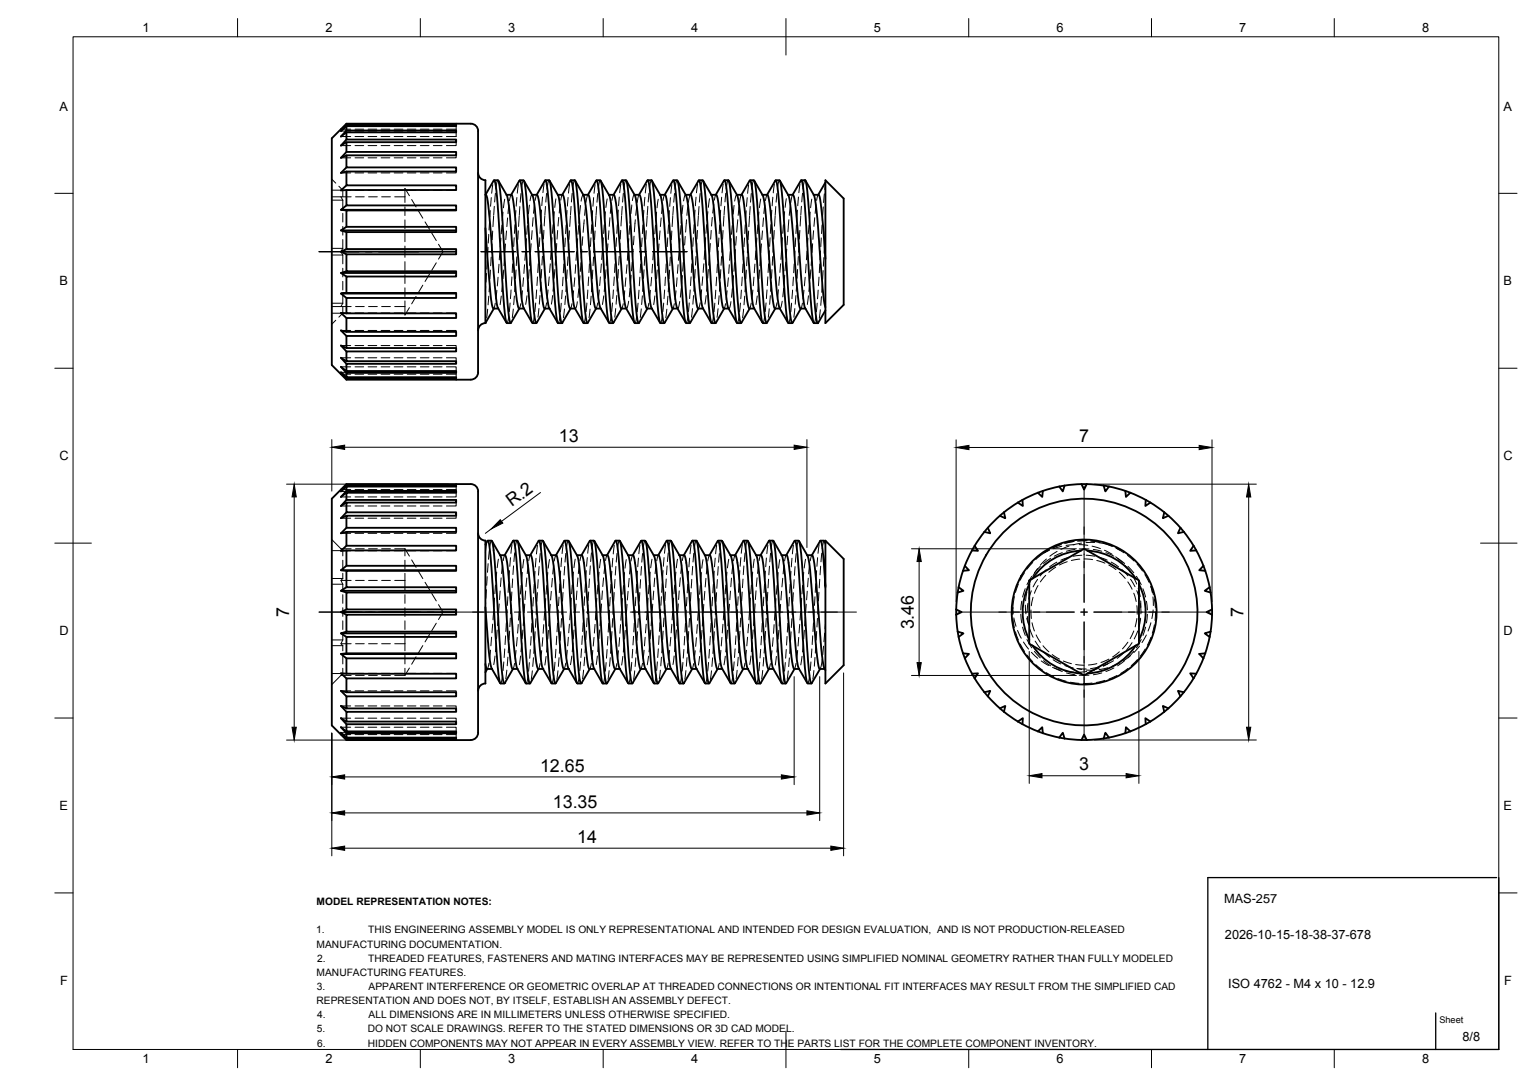
ISO-10303-21;
HEADER;
FILE_DESCRIPTION((''),'2;1');
FILE_NAME('ISO 4762 - M4 x 10 - 12.9.step','2026-10-05T22:33:56+05:00',(''),(''),'','','');
FILE_SCHEMA (('AUTOMOTIVE_DESIGN { 1 0 10303 214 3 1 1 }'));
ENDSEC;
DATA;
#10=MECHANICAL_DESIGN_GEOMETRIC_PRESENTATION_REPRESENTATION('',(#433),#16942);
#231=(
BOUNDED_CURVE()
B_SPLINE_CURVE(2,(#15819,#15820,#15821),.UNSPECIFIED.,.F.,.F.)
B_SPLINE_CURVE_WITH_KNOTS((3,3),(0.0385503582642466,0.0599944283303575),
 .UNSPECIFIED.)
CURVE()
GEOMETRIC_REPRESENTATION_ITEM()
RATIONAL_B_SPLINE_CURVE((1.0010577858677,1.00082309557272,1.))
REPRESENTATION_ITEM('')
) ;
#232=(
BOUNDED_CURVE()
B_SPLINE_CURVE(2,(#15833,#15834,#15835),.UNSPECIFIED.,.F.,.F.)
B_SPLINE_CURVE_WITH_KNOTS((3,3),(0.,0.0214440700661964),.UNSPECIFIED.)
CURVE()
GEOMETRIC_REPRESENTATION_ITEM()
RATIONAL_B_SPLINE_CURVE((1.,1.00082309556609,1.00105778585917))
REPRESENTATION_ITEM('')
) ;
#233=(
BOUNDED_CURVE()
B_SPLINE_CURVE(2,(#16126,#16127,#16128),.UNSPECIFIED.,.F.,.F.)
B_SPLINE_CURVE_WITH_KNOTS((3,3),(0.0385503582641958,0.0599944283303579),
 .UNSPECIFIED.)
CURVE()
GEOMETRIC_REPRESENTATION_ITEM()
RATIONAL_B_SPLINE_CURVE((1.00105778586472,1.00082309557041,1.))
REPRESENTATION_ITEM('')
) ;
#234=(
BOUNDED_CURVE()
B_SPLINE_CURVE(2,(#16135,#16136,#16137),.UNSPECIFIED.,.F.,.F.)
B_SPLINE_CURVE_WITH_KNOTS((3,3),(0.,0.0214440700661411),.UNSPECIFIED.)
CURVE()
GEOMETRIC_REPRESENTATION_ITEM()
RATIONAL_B_SPLINE_CURVE((1.,1.00082309557092,1.00105778586538))
REPRESENTATION_ITEM('')
) ;
#235=(
BOUNDED_CURVE()
B_SPLINE_CURVE(2,(#16140,#16141,#16142),.UNSPECIFIED.,.F.,.F.)
B_SPLINE_CURVE_WITH_KNOTS((3,3),(0.0385503582642588,0.0599944283303573),
 .UNSPECIFIED.)
CURVE()
GEOMETRIC_REPRESENTATION_ITEM()
RATIONAL_B_SPLINE_CURVE((1.00105778587296,1.00082309557682,1.))
REPRESENTATION_ITEM('')
) ;
#236=(
BOUNDED_CURVE()
B_SPLINE_CURVE(2,(#16149,#16150,#16151),.UNSPECIFIED.,.F.,.F.)
B_SPLINE_CURVE_WITH_KNOTS((3,3),(0.,0.0214440700661923),.UNSPECIFIED.)
CURVE()
GEOMETRIC_REPRESENTATION_ITEM()
RATIONAL_B_SPLINE_CURVE((1.,1.00082309556743,1.00105778586089))
REPRESENTATION_ITEM('')
) ;
#237=(
BOUNDED_CURVE()
B_SPLINE_CURVE(2,(#16154,#16155,#16156),.UNSPECIFIED.,.F.,.F.)
B_SPLINE_CURVE_WITH_KNOTS((3,3),(0.0385503582642198,0.0599944283303572),
 .UNSPECIFIED.)
CURVE()
GEOMETRIC_REPRESENTATION_ITEM()
RATIONAL_B_SPLINE_CURVE((1.00105778586562,1.00082309557111,1.))
REPRESENTATION_ITEM('')
) ;
#238=(
BOUNDED_CURVE()
B_SPLINE_CURVE(2,(#16163,#16164,#16165),.UNSPECIFIED.,.F.,.F.)
B_SPLINE_CURVE_WITH_KNOTS((3,3),(0.,0.0214440700661772),.UNSPECIFIED.)
CURVE()
GEOMETRIC_REPRESENTATION_ITEM()
RATIONAL_B_SPLINE_CURVE((1.,1.00082309556912,1.00105778586306))
REPRESENTATION_ITEM('')
) ;
#239=(
BOUNDED_CURVE()
B_SPLINE_CURVE(2,(#16168,#16169,#16170),.UNSPECIFIED.,.F.,.F.)
B_SPLINE_CURVE_WITH_KNOTS((3,3),(0.0385503582641919,0.0599944283303571),
 .UNSPECIFIED.)
CURVE()
GEOMETRIC_REPRESENTATION_ITEM()
RATIONAL_B_SPLINE_CURVE((1.00105778586425,1.00082309557004,1.))
REPRESENTATION_ITEM('')
) ;
#240=(
BOUNDED_CURVE()
B_SPLINE_CURVE(2,(#16177,#16178,#16179),.UNSPECIFIED.,.F.,.F.)
B_SPLINE_CURVE_WITH_KNOTS((3,3),(0.,0.02144407006609),.UNSPECIFIED.)
CURVE()
GEOMETRIC_REPRESENTATION_ITEM()
RATIONAL_B_SPLINE_CURVE((1.,1.0008230955718,1.00105778586652))
REPRESENTATION_ITEM('')
) ;
#241=(
BOUNDED_CURVE()
B_SPLINE_CURVE(2,(#16182,#16183,#16184),.UNSPECIFIED.,.F.,.F.)
B_SPLINE_CURVE_WITH_KNOTS((3,3),(0.0385503582642022,0.0599944283303558),
 .UNSPECIFIED.)
CURVE()
GEOMETRIC_REPRESENTATION_ITEM()
RATIONAL_B_SPLINE_CURVE((1.00105778586255,1.00082309556872,1.))
REPRESENTATION_ITEM('')
) ;
#242=(
BOUNDED_CURVE()
B_SPLINE_CURVE(2,(#16191,#16192,#16193),.UNSPECIFIED.,.F.,.F.)
B_SPLINE_CURVE_WITH_KNOTS((3,3),(0.,0.0214440700661625),.UNSPECIFIED.)
CURVE()
GEOMETRIC_REPRESENTATION_ITEM()
RATIONAL_B_SPLINE_CURVE((1.,1.00082309557089,1.00105778586534))
REPRESENTATION_ITEM('')
) ;
#243=(
BOUNDED_CURVE()
B_SPLINE_CURVE(2,(#16196,#16197,#16198),.UNSPECIFIED.,.F.,.F.)
B_SPLINE_CURVE_WITH_KNOTS((3,3),(0.038550358264205,0.0599944283303565),
 .UNSPECIFIED.)
CURVE()
GEOMETRIC_REPRESENTATION_ITEM()
RATIONAL_B_SPLINE_CURVE((1.00105778586624,1.00082309557159,1.))
REPRESENTATION_ITEM('')
) ;
#244=(
BOUNDED_CURVE()
B_SPLINE_CURVE(2,(#16205,#16206,#16207),.UNSPECIFIED.,.F.,.F.)
B_SPLINE_CURVE_WITH_KNOTS((3,3),(0.,0.0214440700661342),.UNSPECIFIED.)
CURVE()
GEOMETRIC_REPRESENTATION_ITEM()
RATIONAL_B_SPLINE_CURVE((1.,1.00082309557258,1.00105778586751))
REPRESENTATION_ITEM('')
) ;
#245=(
BOUNDED_CURVE()
B_SPLINE_CURVE(2,(#16210,#16211,#16212),.UNSPECIFIED.,.F.,.F.)
B_SPLINE_CURVE_WITH_KNOTS((3,3),(0.0385503582641691,0.0599944283303568),
 .UNSPECIFIED.)
CURVE()
GEOMETRIC_REPRESENTATION_ITEM()
RATIONAL_B_SPLINE_CURVE((1.00105778586269,1.00082309556883,1.))
REPRESENTATION_ITEM('')
) ;
#246=(
BOUNDED_CURVE()
B_SPLINE_CURVE(2,(#16219,#16220,#16221),.UNSPECIFIED.,.F.,.F.)
B_SPLINE_CURVE_WITH_KNOTS((3,3),(0.,0.0214440700661154),.UNSPECIFIED.)
CURVE()
GEOMETRIC_REPRESENTATION_ITEM()
RATIONAL_B_SPLINE_CURVE((1.,1.00082309557543,1.00105778587117))
REPRESENTATION_ITEM('')
) ;
#247=(
BOUNDED_CURVE()
B_SPLINE_CURVE(2,(#16224,#16225,#16226),.UNSPECIFIED.,.F.,.F.)
B_SPLINE_CURVE_WITH_KNOTS((3,3),(0.0385503582642171,0.0599944283303574),
 .UNSPECIFIED.)
CURVE()
GEOMETRIC_REPRESENTATION_ITEM()
RATIONAL_B_SPLINE_CURVE((1.00105778586904,1.00082309557377,1.))
REPRESENTATION_ITEM('')
) ;
#248=(
BOUNDED_CURVE()
B_SPLINE_CURVE(2,(#16233,#16234,#16235),.UNSPECIFIED.,.F.,.F.)
B_SPLINE_CURVE_WITH_KNOTS((3,3),(0.,0.0214440700661167),.UNSPECIFIED.)
CURVE()
GEOMETRIC_REPRESENTATION_ITEM()
RATIONAL_B_SPLINE_CURVE((1.,1.00082309557365,1.00105778586889))
REPRESENTATION_ITEM('')
) ;
#249=(
BOUNDED_CURVE()
B_SPLINE_CURVE(2,(#16238,#16239,#16240),.UNSPECIFIED.,.F.,.F.)
B_SPLINE_CURVE_WITH_KNOTS((3,3),(0.0385503582642811,0.0599944283303564),
 .UNSPECIFIED.)
CURVE()
GEOMETRIC_REPRESENTATION_ITEM()
RATIONAL_B_SPLINE_CURVE((1.00105778587046,1.00082309557487,1.))
REPRESENTATION_ITEM('')
) ;
#250=(
BOUNDED_CURVE()
B_SPLINE_CURVE(2,(#16247,#16248,#16249),.UNSPECIFIED.,.F.,.F.)
B_SPLINE_CURVE_WITH_KNOTS((3,3),(0.,0.0214440700661453),.UNSPECIFIED.)
CURVE()
GEOMETRIC_REPRESENTATION_ITEM()
RATIONAL_B_SPLINE_CURVE((1.,1.00082309557136,1.00105778586595))
REPRESENTATION_ITEM('')
) ;
#251=(
BOUNDED_CURVE()
B_SPLINE_CURVE(2,(#16252,#16253,#16254),.UNSPECIFIED.,.F.,.F.)
B_SPLINE_CURVE_WITH_KNOTS((3,3),(0.0385503582642705,0.0599944283303552),
 .UNSPECIFIED.)
CURVE()
GEOMETRIC_REPRESENTATION_ITEM()
RATIONAL_B_SPLINE_CURVE((1.00105778586715,1.0008230955723,1.))
REPRESENTATION_ITEM('')
) ;
#252=(
BOUNDED_CURVE()
B_SPLINE_CURVE(2,(#16261,#16262,#16263),.UNSPECIFIED.,.F.,.F.)
B_SPLINE_CURVE_WITH_KNOTS((3,3),(0.,0.0214440700661215),.UNSPECIFIED.)
CURVE()
GEOMETRIC_REPRESENTATION_ITEM()
RATIONAL_B_SPLINE_CURVE((1.,1.00082309557137,1.00105778586595))
REPRESENTATION_ITEM('')
) ;
#253=(
BOUNDED_CURVE()
B_SPLINE_CURVE(2,(#16266,#16267,#16268),.UNSPECIFIED.,.F.,.F.)
B_SPLINE_CURVE_WITH_KNOTS((3,3),(0.0385503582641931,0.0599944283303567),
 .UNSPECIFIED.)
CURVE()
GEOMETRIC_REPRESENTATION_ITEM()
RATIONAL_B_SPLINE_CURVE((1.00105778586386,1.00082309556974,1.))
REPRESENTATION_ITEM('')
) ;
#254=(
BOUNDED_CURVE()
B_SPLINE_CURVE(2,(#16275,#16276,#16277),.UNSPECIFIED.,.F.,.F.)
B_SPLINE_CURVE_WITH_KNOTS((3,3),(0.,0.0214440700661656),.UNSPECIFIED.)
CURVE()
GEOMETRIC_REPRESENTATION_ITEM()
RATIONAL_B_SPLINE_CURVE((1.,1.00082309557042,1.00105778586474))
REPRESENTATION_ITEM('')
) ;
#255=(
BOUNDED_CURVE()
B_SPLINE_CURVE(2,(#16280,#16281,#16282),.UNSPECIFIED.,.F.,.F.)
B_SPLINE_CURVE_WITH_KNOTS((3,3),(0.0385503582642439,0.0599944283303563),
 .UNSPECIFIED.)
CURVE()
GEOMETRIC_REPRESENTATION_ITEM()
RATIONAL_B_SPLINE_CURVE((1.00105778586994,1.00082309557447,1.))
REPRESENTATION_ITEM('')
) ;
#256=(
BOUNDED_CURVE()
B_SPLINE_CURVE(2,(#16289,#16290,#16291),.UNSPECIFIED.,.F.,.F.)
B_SPLINE_CURVE_WITH_KNOTS((3,3),(0.,0.0214440700660658),.UNSPECIFIED.)
CURVE()
GEOMETRIC_REPRESENTATION_ITEM()
RATIONAL_B_SPLINE_CURVE((1.,1.00082309557484,1.00105778587042))
REPRESENTATION_ITEM('')
) ;
#257=(
BOUNDED_CURVE()
B_SPLINE_CURVE(2,(#16294,#16295,#16296),.UNSPECIFIED.,.F.,.F.)
B_SPLINE_CURVE_WITH_KNOTS((3,3),(0.0385503582642125,0.0599944283303565),
 .UNSPECIFIED.)
CURVE()
GEOMETRIC_REPRESENTATION_ITEM()
RATIONAL_B_SPLINE_CURVE((1.00105778586599,1.0008230955714,1.))
REPRESENTATION_ITEM('')
) ;
#258=(
BOUNDED_CURVE()
B_SPLINE_CURVE(2,(#16303,#16304,#16305),.UNSPECIFIED.,.F.,.F.)
B_SPLINE_CURVE_WITH_KNOTS((3,3),(0.,0.0214440700661045),.UNSPECIFIED.)
CURVE()
GEOMETRIC_REPRESENTATION_ITEM()
RATIONAL_B_SPLINE_CURVE((1.,1.00082309557375,1.00105778586901))
REPRESENTATION_ITEM('')
) ;
#259=(
BOUNDED_CURVE()
B_SPLINE_CURVE(2,(#16308,#16309,#16310),.UNSPECIFIED.,.F.,.F.)
B_SPLINE_CURVE_WITH_KNOTS((3,3),(0.0385503582642445,0.0599944283303561),
 .UNSPECIFIED.)
CURVE()
GEOMETRIC_REPRESENTATION_ITEM()
RATIONAL_B_SPLINE_CURVE((1.00105778586579,1.00082309557124,1.))
REPRESENTATION_ITEM('')
) ;
#260=(
BOUNDED_CURVE()
B_SPLINE_CURVE(2,(#16317,#16318,#16319),.UNSPECIFIED.,.F.,.F.)
B_SPLINE_CURVE_WITH_KNOTS((3,3),(0.,0.021444070066132),.UNSPECIFIED.)
CURVE()
GEOMETRIC_REPRESENTATION_ITEM()
RATIONAL_B_SPLINE_CURVE((1.,1.00082309557227,1.00105778586711))
REPRESENTATION_ITEM('')
) ;
#261=(
BOUNDED_CURVE()
B_SPLINE_CURVE(2,(#16322,#16323,#16324),.UNSPECIFIED.,.F.,.F.)
B_SPLINE_CURVE_WITH_KNOTS((3,3),(0.03855035826422,0.0599944283303558),
 .UNSPECIFIED.)
CURVE()
GEOMETRIC_REPRESENTATION_ITEM()
RATIONAL_B_SPLINE_CURVE((1.00105778586627,1.00082309557161,1.))
REPRESENTATION_ITEM('')
) ;
#262=(
BOUNDED_CURVE()
B_SPLINE_CURVE(2,(#16331,#16332,#16333),.UNSPECIFIED.,.F.,.F.)
B_SPLINE_CURVE_WITH_KNOTS((3,3),(0.,0.0214440700661134),.UNSPECIFIED.)
CURVE()
GEOMETRIC_REPRESENTATION_ITEM()
RATIONAL_B_SPLINE_CURVE((1.,1.00082309557282,1.00105778586782))
REPRESENTATION_ITEM('')
) ;
#263=(
BOUNDED_CURVE()
B_SPLINE_CURVE(2,(#16336,#16337,#16338),.UNSPECIFIED.,.F.,.F.)
B_SPLINE_CURVE_WITH_KNOTS((3,3),(0.0385503582642076,0.0599944283303568),
 .UNSPECIFIED.)
CURVE()
GEOMETRIC_REPRESENTATION_ITEM()
RATIONAL_B_SPLINE_CURVE((1.00105778586756,1.00082309557262,1.))
REPRESENTATION_ITEM('')
) ;
#264=(
BOUNDED_CURVE()
B_SPLINE_CURVE(2,(#16345,#16346,#16347),.UNSPECIFIED.,.F.,.F.)
B_SPLINE_CURVE_WITH_KNOTS((3,3),(0.,0.0214440700660783),.UNSPECIFIED.)
CURVE()
GEOMETRIC_REPRESENTATION_ITEM()
RATIONAL_B_SPLINE_CURVE((1.,1.00082309557531,1.00105778587102))
REPRESENTATION_ITEM('')
) ;
#265=(
BOUNDED_CURVE()
B_SPLINE_CURVE(2,(#16350,#16351,#16352),.UNSPECIFIED.,.F.,.F.)
B_SPLINE_CURVE_WITH_KNOTS((3,3),(0.0385503582642354,0.0599944283303562),
 .UNSPECIFIED.)
CURVE()
GEOMETRIC_REPRESENTATION_ITEM()
RATIONAL_B_SPLINE_CURVE((1.0010577858655,1.00082309557101,1.))
REPRESENTATION_ITEM('')
) ;
#266=(
BOUNDED_CURVE()
B_SPLINE_CURVE(2,(#16359,#16360,#16361),.UNSPECIFIED.,.F.,.F.)
B_SPLINE_CURVE_WITH_KNOTS((3,3),(0.,0.021444070066152),.UNSPECIFIED.)
CURVE()
GEOMETRIC_REPRESENTATION_ITEM()
RATIONAL_B_SPLINE_CURVE((1.,1.00082309556975,1.00105778586387))
REPRESENTATION_ITEM('')
) ;
#267=(
BOUNDED_CURVE()
B_SPLINE_CURVE(2,(#16364,#16365,#16366),.UNSPECIFIED.,.F.,.F.)
B_SPLINE_CURVE_WITH_KNOTS((3,3),(0.0385503582642177,0.0599944283303568),
 .UNSPECIFIED.)
CURVE()
GEOMETRIC_REPRESENTATION_ITEM()
RATIONAL_B_SPLINE_CURVE((1.00105778586644,1.00082309557175,1.))
REPRESENTATION_ITEM('')
) ;
#268=(
BOUNDED_CURVE()
B_SPLINE_CURVE(2,(#16373,#16374,#16375),.UNSPECIFIED.,.F.,.F.)
B_SPLINE_CURVE_WITH_KNOTS((3,3),(0.,0.0214440700661323),.UNSPECIFIED.)
CURVE()
GEOMETRIC_REPRESENTATION_ITEM()
RATIONAL_B_SPLINE_CURVE((1.,1.00082309557161,1.00105778586626))
REPRESENTATION_ITEM('')
) ;
#269=(
BOUNDED_CURVE()
B_SPLINE_CURVE(2,(#16378,#16379,#16380),.UNSPECIFIED.,.F.,.F.)
B_SPLINE_CURVE_WITH_KNOTS((3,3),(0.0385503582642313,0.0599944283303566),
 .UNSPECIFIED.)
CURVE()
GEOMETRIC_REPRESENTATION_ITEM()
RATIONAL_B_SPLINE_CURVE((1.00105778586689,1.0008230955721,1.))
REPRESENTATION_ITEM('')
) ;
#270=(
BOUNDED_CURVE()
B_SPLINE_CURVE(2,(#16387,#16388,#16389),.UNSPECIFIED.,.F.,.F.)
B_SPLINE_CURVE_WITH_KNOTS((3,3),(0.,0.0214440700661231),.UNSPECIFIED.)
CURVE()
GEOMETRIC_REPRESENTATION_ITEM()
RATIONAL_B_SPLINE_CURVE((1.,1.00082309557192,1.00105778586666))
REPRESENTATION_ITEM('')
) ;
#271=(
BOUNDED_CURVE()
B_SPLINE_CURVE(2,(#16392,#16393,#16394),.UNSPECIFIED.,.F.,.F.)
B_SPLINE_CURVE_WITH_KNOTS((3,3),(0.0385503582642438,0.0599944283303561),
 .UNSPECIFIED.)
CURVE()
GEOMETRIC_REPRESENTATION_ITEM()
RATIONAL_B_SPLINE_CURVE((1.00105778586773,1.00082309557275,1.))
REPRESENTATION_ITEM('')
) ;
#272=(
BOUNDED_CURVE()
B_SPLINE_CURVE(2,(#16401,#16402,#16403),.UNSPECIFIED.,.F.,.F.)
B_SPLINE_CURVE_WITH_KNOTS((3,3),(0.,0.0214440700661489),.UNSPECIFIED.)
CURVE()
GEOMETRIC_REPRESENTATION_ITEM()
RATIONAL_B_SPLINE_CURVE((1.,1.00082309557108,1.00105778586558))
REPRESENTATION_ITEM('')
) ;
#273=(
BOUNDED_CURVE()
B_SPLINE_CURVE(2,(#16406,#16407,#16408),.UNSPECIFIED.,.F.,.F.)
B_SPLINE_CURVE_WITH_KNOTS((3,3),(0.0385503582642491,0.0599944283303561),
 .UNSPECIFIED.)
CURVE()
GEOMETRIC_REPRESENTATION_ITEM()
RATIONAL_B_SPLINE_CURVE((1.00105778586862,1.00082309557344,1.))
REPRESENTATION_ITEM('')
) ;
#274=(
BOUNDED_CURVE()
B_SPLINE_CURVE(2,(#16415,#16416,#16417),.UNSPECIFIED.,.F.,.F.)
B_SPLINE_CURVE_WITH_KNOTS((3,3),(0.,0.0214440700660912),.UNSPECIFIED.)
CURVE()
GEOMETRIC_REPRESENTATION_ITEM()
RATIONAL_B_SPLINE_CURVE((1.,1.00082309557531,1.00105778587103))
REPRESENTATION_ITEM('')
) ;
#275=(
BOUNDED_CURVE()
B_SPLINE_CURVE(2,(#16420,#16421,#16422),.UNSPECIFIED.,.F.,.F.)
B_SPLINE_CURVE_WITH_KNOTS((3,3),(0.0385503582642475,0.0599944283303563),
 .UNSPECIFIED.)
CURVE()
GEOMETRIC_REPRESENTATION_ITEM()
RATIONAL_B_SPLINE_CURVE((1.0010577858671,1.00082309557226,1.))
REPRESENTATION_ITEM('')
) ;
#276=(
BOUNDED_CURVE()
B_SPLINE_CURVE(2,(#16429,#16430,#16431),.UNSPECIFIED.,.F.,.F.)
B_SPLINE_CURVE_WITH_KNOTS((3,3),(0.,0.0214440700661173),.UNSPECIFIED.)
CURVE()
GEOMETRIC_REPRESENTATION_ITEM()
RATIONAL_B_SPLINE_CURVE((1.,1.00082309557298,1.00105778586803))
REPRESENTATION_ITEM('')
) ;
#277=(
BOUNDED_CURVE()
B_SPLINE_CURVE(2,(#16434,#16435,#16436),.UNSPECIFIED.,.F.,.F.)
B_SPLINE_CURVE_WITH_KNOTS((3,3),(0.0385503582641958,0.0599944283303564),
 .UNSPECIFIED.)
CURVE()
GEOMETRIC_REPRESENTATION_ITEM()
RATIONAL_B_SPLINE_CURVE((1.00105778586416,1.00082309556997,1.))
REPRESENTATION_ITEM('')
) ;
#278=(
BOUNDED_CURVE()
B_SPLINE_CURVE(2,(#16443,#16444,#16445),.UNSPECIFIED.,.F.,.F.)
B_SPLINE_CURVE_WITH_KNOTS((3,3),(0.,0.0214440700660895),.UNSPECIFIED.)
CURVE()
GEOMETRIC_REPRESENTATION_ITEM()
RATIONAL_B_SPLINE_CURVE((1.,1.00082309557376,1.00105778586903))
REPRESENTATION_ITEM('')
) ;
#279=(
BOUNDED_CURVE()
B_SPLINE_CURVE(2,(#16448,#16449,#16450),.UNSPECIFIED.,.F.,.F.)
B_SPLINE_CURVE_WITH_KNOTS((3,3),(0.0385503582642543,0.0599944283303558),
 .UNSPECIFIED.)
CURVE()
GEOMETRIC_REPRESENTATION_ITEM()
RATIONAL_B_SPLINE_CURVE((1.00105778586867,1.00082309557348,1.))
REPRESENTATION_ITEM('')
) ;
#280=(
BOUNDED_CURVE()
B_SPLINE_CURVE(2,(#16457,#16458,#16459),.UNSPECIFIED.,.F.,.F.)
B_SPLINE_CURVE_WITH_KNOTS((3,3),(0.,0.0214440700661381),.UNSPECIFIED.)
CURVE()
GEOMETRIC_REPRESENTATION_ITEM()
RATIONAL_B_SPLINE_CURVE((1.,1.00082309557261,1.00105778586756))
REPRESENTATION_ITEM('')
) ;
#281=(
BOUNDED_CURVE()
B_SPLINE_CURVE(2,(#16462,#16463,#16464),.UNSPECIFIED.,.F.,.F.)
B_SPLINE_CURVE_WITH_KNOTS((3,3),(0.0385503582642087,0.0599944283303561),
 .UNSPECIFIED.)
CURVE()
GEOMETRIC_REPRESENTATION_ITEM()
RATIONAL_B_SPLINE_CURVE((1.00105778586395,1.0008230955698,1.))
REPRESENTATION_ITEM('')
) ;
#282=(
BOUNDED_CURVE()
B_SPLINE_CURVE(2,(#16471,#16472,#16473),.UNSPECIFIED.,.F.,.F.)
B_SPLINE_CURVE_WITH_KNOTS((3,3),(0.,0.0214440700661082),.UNSPECIFIED.)
CURVE()
GEOMETRIC_REPRESENTATION_ITEM()
RATIONAL_B_SPLINE_CURVE((1.,1.00082309557413,1.00105778586951))
REPRESENTATION_ITEM('')
) ;
#283=(
BOUNDED_CURVE()
B_SPLINE_CURVE(2,(#16476,#16477,#16478),.UNSPECIFIED.,.F.,.F.)
B_SPLINE_CURVE_WITH_KNOTS((3,3),(0.0385503582642435,0.0599944283303565),
 .UNSPECIFIED.)
CURVE()
GEOMETRIC_REPRESENTATION_ITEM()
RATIONAL_B_SPLINE_CURVE((1.00105778586698,1.00082309557217,1.))
REPRESENTATION_ITEM('')
) ;
#284=(
BOUNDED_CURVE()
B_SPLINE_CURVE(2,(#16485,#16486,#16487),.UNSPECIFIED.,.F.,.F.)
B_SPLINE_CURVE_WITH_KNOTS((3,3),(0.,0.0214440700661165),.UNSPECIFIED.)
CURVE()
GEOMETRIC_REPRESENTATION_ITEM()
RATIONAL_B_SPLINE_CURVE((1.,1.00082309557299,1.00105778586805))
REPRESENTATION_ITEM('')
) ;
#285=(
BOUNDED_CURVE()
B_SPLINE_CURVE(2,(#16490,#16491,#16492),.UNSPECIFIED.,.F.,.F.)
B_SPLINE_CURVE_WITH_KNOTS((3,3),(0.0385503582642354,0.0599944283303561),
 .UNSPECIFIED.)
CURVE()
GEOMETRIC_REPRESENTATION_ITEM()
RATIONAL_B_SPLINE_CURVE((1.00105778586729,1.00082309557241,1.))
REPRESENTATION_ITEM('')
) ;
#286=(
BOUNDED_CURVE()
B_SPLINE_CURVE(2,(#16499,#16500,#16501),.UNSPECIFIED.,.F.,.F.)
B_SPLINE_CURVE_WITH_KNOTS((3,3),(0.,0.0214440700661208),.UNSPECIFIED.)
CURVE()
GEOMETRIC_REPRESENTATION_ITEM()
RATIONAL_B_SPLINE_CURVE((1.,1.00082309557164,1.0010577858663))
REPRESENTATION_ITEM('')
) ;
#287=(
BOUNDED_CURVE()
B_SPLINE_CURVE(2,(#16504,#16505,#16506),.UNSPECIFIED.,.F.,.F.)
B_SPLINE_CURVE_WITH_KNOTS((3,3),(0.0385503582642138,0.0599944283303558),
 .UNSPECIFIED.)
CURVE()
GEOMETRIC_REPRESENTATION_ITEM()
RATIONAL_B_SPLINE_CURVE((1.0010577858656,1.00082309557109,1.))
REPRESENTATION_ITEM('')
) ;
#288=(
BOUNDED_CURVE()
B_SPLINE_CURVE(2,(#16513,#16514,#16515),.UNSPECIFIED.,.F.,.F.)
B_SPLINE_CURVE_WITH_KNOTS((3,3),(0.,0.0214440700661239),.UNSPECIFIED.)
CURVE()
GEOMETRIC_REPRESENTATION_ITEM()
RATIONAL_B_SPLINE_CURVE((1.,1.00082309557102,1.0010577858655))
REPRESENTATION_ITEM('')
) ;
#289=(
BOUNDED_CURVE()
B_SPLINE_CURVE(2,(#16518,#16519,#16520),.UNSPECIFIED.,.F.,.F.)
B_SPLINE_CURVE_WITH_KNOTS((3,3),(0.0385503582643101,0.0599944283303554),
 .UNSPECIFIED.)
CURVE()
GEOMETRIC_REPRESENTATION_ITEM()
RATIONAL_B_SPLINE_CURVE((1.00105778587441,1.00082309557795,1.))
REPRESENTATION_ITEM('')
) ;
#290=(
BOUNDED_CURVE()
B_SPLINE_CURVE(2,(#16527,#16528,#16529),.UNSPECIFIED.,.F.,.F.)
B_SPLINE_CURVE_WITH_KNOTS((3,3),(0.,0.021444070066082),.UNSPECIFIED.)
CURVE()
GEOMETRIC_REPRESENTATION_ITEM()
RATIONAL_B_SPLINE_CURVE((1.,1.0008230955747,1.00105778587023))
REPRESENTATION_ITEM('')
) ;
#291=(
BOUNDED_CURVE()
B_SPLINE_CURVE(2,(#16532,#16533,#16534),.UNSPECIFIED.,.F.,.F.)
B_SPLINE_CURVE_WITH_KNOTS((3,3),(0.0385503582643354,0.0599944283303546),
 .UNSPECIFIED.)
CURVE()
GEOMETRIC_REPRESENTATION_ITEM()
RATIONAL_B_SPLINE_CURVE((1.00105778587483,1.00082309557827,1.))
REPRESENTATION_ITEM('')
) ;
#292=(
BOUNDED_CURVE()
B_SPLINE_CURVE(2,(#16541,#16542,#16543),.UNSPECIFIED.,.F.,.F.)
B_SPLINE_CURVE_WITH_KNOTS((3,3),(0.,0.0214440700660534),.UNSPECIFIED.)
CURVE()
GEOMETRIC_REPRESENTATION_ITEM()
RATIONAL_B_SPLINE_CURVE((1.,1.0008230955765,1.00105778587255))
REPRESENTATION_ITEM('')
) ;
#293=(
BOUNDED_CURVE()
B_SPLINE_CURVE(2,(#16546,#16547,#16548),.UNSPECIFIED.,.F.,.F.)
B_SPLINE_CURVE_WITH_KNOTS((3,3),(0.038550358264337,0.0599944283303554),
 .UNSPECIFIED.)
CURVE()
GEOMETRIC_REPRESENTATION_ITEM()
RATIONAL_B_SPLINE_CURVE((1.00105778587529,1.00082309557863,1.))
REPRESENTATION_ITEM('')
) ;
#294=(
BOUNDED_CURVE()
B_SPLINE_CURVE(2,(#16555,#16556,#16557),.UNSPECIFIED.,.F.,.F.)
B_SPLINE_CURVE_WITH_KNOTS((3,3),(0.,0.0214440700660699),.UNSPECIFIED.)
CURVE()
GEOMETRIC_REPRESENTATION_ITEM()
RATIONAL_B_SPLINE_CURVE((1.,1.00082309557688,1.00105778587304))
REPRESENTATION_ITEM('')
) ;
#295=(
BOUNDED_CURVE()
B_SPLINE_CURVE(2,(#16560,#16561,#16562),.UNSPECIFIED.,.F.,.F.)
B_SPLINE_CURVE_WITH_KNOTS((3,3),(0.0385503582642283,0.0599944283303555),
 .UNSPECIFIED.)
CURVE()
GEOMETRIC_REPRESENTATION_ITEM()
RATIONAL_B_SPLINE_CURVE((1.00105778586715,1.0008230955723,1.))
REPRESENTATION_ITEM('')
) ;
#296=(
BOUNDED_CURVE()
B_SPLINE_CURVE(2,(#16569,#16570,#16571),.UNSPECIFIED.,.F.,.F.)
B_SPLINE_CURVE_WITH_KNOTS((3,3),(0.,0.0214440700660926),.UNSPECIFIED.)
CURVE()
GEOMETRIC_REPRESENTATION_ITEM()
RATIONAL_B_SPLINE_CURVE((1.,1.00082309557397,1.0010577858693))
REPRESENTATION_ITEM('')
) ;
#297=(
BOUNDED_CURVE()
B_SPLINE_CURVE(2,(#16574,#16575,#16576),.UNSPECIFIED.,.F.,.F.)
B_SPLINE_CURVE_WITH_KNOTS((3,3),(0.0385503582642555,0.0599944283303555),
 .UNSPECIFIED.)
CURVE()
GEOMETRIC_REPRESENTATION_ITEM()
RATIONAL_B_SPLINE_CURVE((1.00105778587096,1.00082309557526,1.))
REPRESENTATION_ITEM('')
) ;
#298=(
BOUNDED_CURVE()
B_SPLINE_CURVE(2,(#16583,#16584,#16585),.UNSPECIFIED.,.F.,.F.)
B_SPLINE_CURVE_WITH_KNOTS((3,3),(0.,0.0214440700660555),.UNSPECIFIED.)
CURVE()
GEOMETRIC_REPRESENTATION_ITEM()
RATIONAL_B_SPLINE_CURVE((1.,1.00082309557703,1.00105778587323))
REPRESENTATION_ITEM('')
) ;
#299=(
BOUNDED_CURVE()
B_SPLINE_CURVE(2,(#16588,#16589,#16590),.UNSPECIFIED.,.F.,.F.)
B_SPLINE_CURVE_WITH_KNOTS((3,3),(0.0385503582642982,0.059994428330355),
 .UNSPECIFIED.)
CURVE()
GEOMETRIC_REPRESENTATION_ITEM()
RATIONAL_B_SPLINE_CURVE((1.00105778587101,1.0008230955753,1.))
REPRESENTATION_ITEM('')
) ;
#300=(
BOUNDED_CURVE()
B_SPLINE_CURVE(2,(#16597,#16598,#16599),.UNSPECIFIED.,.F.,.F.)
B_SPLINE_CURVE_WITH_KNOTS((3,3),(0.,0.0214440700660737),.UNSPECIFIED.)
CURVE()
GEOMETRIC_REPRESENTATION_ITEM()
RATIONAL_B_SPLINE_CURVE((1.,1.00082309557534,1.00105778587106))
REPRESENTATION_ITEM('')
) ;
#301=(
BOUNDED_CURVE()
B_SPLINE_CURVE(2,(#16602,#16603,#16604),.UNSPECIFIED.,.F.,.F.)
B_SPLINE_CURVE_WITH_KNOTS((3,3),(0.0385503582642702,0.0599944283303555),
 .UNSPECIFIED.)
CURVE()
GEOMETRIC_REPRESENTATION_ITEM()
RATIONAL_B_SPLINE_CURVE((1.00105778587074,1.00082309557509,1.))
REPRESENTATION_ITEM('')
) ;
#302=(
BOUNDED_CURVE()
B_SPLINE_CURVE(2,(#16611,#16612,#16613),.UNSPECIFIED.,.F.,.F.)
B_SPLINE_CURVE_WITH_KNOTS((3,3),(0.,0.0214440700660954),.UNSPECIFIED.)
CURVE()
GEOMETRIC_REPRESENTATION_ITEM()
RATIONAL_B_SPLINE_CURVE((1.,1.00082309557337,1.00105778586853))
REPRESENTATION_ITEM('')
) ;
#303=(
BOUNDED_CURVE()
B_SPLINE_CURVE(2,(#16626,#16627,#16628),.UNSPECIFIED.,.F.,.F.)
B_SPLINE_CURVE_WITH_KNOTS((3,3),(0.,0.0128119220385747),.UNSPECIFIED.)
CURVE()
GEOMETRIC_REPRESENTATION_ITEM()
RATIONAL_B_SPLINE_CURVE((1.,1.00225826788916,1.0035731078451))
REPRESENTATION_ITEM('')
) ;
#304=(
BOUNDED_CURVE()
B_SPLINE_CURVE(2,(#16632,#16633,#16634),.UNSPECIFIED.,.F.,.F.)
B_SPLINE_CURVE_WITH_KNOTS((3,3),(0.0485234510605496,0.0613353730991217),
 .UNSPECIFIED.)
CURVE()
GEOMETRIC_REPRESENTATION_ITEM()
RATIONAL_B_SPLINE_CURVE((1.00357310784516,1.0022582678892,1.))
REPRESENTATION_ITEM('')
) ;
#305=(
BOUNDED_CURVE()
B_SPLINE_CURVE(2,(#16636,#16637,#16638),.UNSPECIFIED.,.F.,.F.)
B_SPLINE_CURVE_WITH_KNOTS((3,3),(0.,0.0128119217509423),.UNSPECIFIED.)
CURVE()
GEOMETRIC_REPRESENTATION_ITEM()
RATIONAL_B_SPLINE_CURVE((1.,1.00225826778645,1.00357310769076))
REPRESENTATION_ITEM('')
) ;
#306=(
BOUNDED_CURVE()
B_SPLINE_CURVE(2,(#16642,#16643,#16644),.UNSPECIFIED.,.F.,.F.)
B_SPLINE_CURVE_WITH_KNOTS((3,3),(0.0485234554560875,0.0613353722533859),
 .UNSPECIFIED.)
CURVE()
GEOMETRIC_REPRESENTATION_ITEM()
RATIONAL_B_SPLINE_CURVE((1.00357310667489,1.00225826691386,1.))
REPRESENTATION_ITEM('')
) ;
#307=(
BOUNDED_CURVE()
B_SPLINE_CURVE(2,(#16646,#16647,#16648),.UNSPECIFIED.,.F.,.F.)
B_SPLINE_CURVE_WITH_KNOTS((3,3),(0.,0.0128119162220165),.UNSPECIFIED.)
CURVE()
GEOMETRIC_REPRESENTATION_ITEM()
RATIONAL_B_SPLINE_CURVE((1.,1.00225826670891,1.00357310636695))
REPRESENTATION_ITEM('')
) ;
#308=(
BOUNDED_CURVE()
B_SPLINE_CURVE(2,(#16652,#16653,#16654),.UNSPECIFIED.,.F.,.F.)
B_SPLINE_CURVE_WITH_KNOTS((3,3),(0.048523459293524,0.0613353705619148),
 .UNSPECIFIED.)
CURVE()
GEOMETRIC_REPRESENTATION_ITEM()
RATIONAL_B_SPLINE_CURVE((1.00357310535024,1.00225826583579,1.))
REPRESENTATION_ITEM('')
) ;
#309=(
BOUNDED_CURVE()
B_SPLINE_CURVE(2,(#16656,#16657,#16658),.UNSPECIFIED.,.F.,.F.)
B_SPLINE_CURVE_WITH_KNOTS((3,3),(0.,0.0128119109807577),.UNSPECIFIED.)
CURVE()
GEOMETRIC_REPRESENTATION_ITEM()
RATIONAL_B_SPLINE_CURVE((1.,1.002258265733,1.00357310519577))
REPRESENTATION_ITEM('')
) ;
#310=(
BOUNDED_CURVE()
B_SPLINE_CURVE(2,(#16662,#16663,#16664),.UNSPECIFIED.,.F.,.F.)
B_SPLINE_CURVE_WITH_KNOTS((3,3),(0.0485234587354268,0.0613353697161783),
 .UNSPECIFIED.)
CURVE()
GEOMETRIC_REPRESENTATION_ITEM()
RATIONAL_B_SPLINE_CURVE((1.00357310519621,1.00225826573327,1.))
REPRESENTATION_ITEM('')
) ;
#311=(
BOUNDED_CURVE()
B_SPLINE_CURVE(2,(#16666,#16667,#16668),.UNSPECIFIED.,.F.,.F.)
B_SPLINE_CURVE_WITH_KNOTS((3,3),(0.,0.0128119112683924),.UNSPECIFIED.)
CURVE()
GEOMETRIC_REPRESENTATION_ITEM()
RATIONAL_B_SPLINE_CURVE((1.,1.00225826583572,1.00357310535012))
REPRESENTATION_ITEM('')
) ;
#312=(
BOUNDED_CURVE()
B_SPLINE_CURVE(2,(#16672,#16673,#16674),.UNSPECIFIED.,.F.,.F.)
B_SPLINE_CURVE_WITH_KNOTS((3,3),(0.0485234543398934,0.0613353705619145),
 .UNSPECIFIED.)
CURVE()
GEOMETRIC_REPRESENTATION_ITEM()
RATIONAL_B_SPLINE_CURVE((1.00357310636678,1.0022582667088,1.))
REPRESENTATION_ITEM('')
) ;
#313=(
BOUNDED_CURVE()
B_SPLINE_CURVE(2,(#16677,#16678,#16679),.UNSPECIFIED.,.F.,.F.)
B_SPLINE_CURVE_WITH_KNOTS((3,3),(0.,0.0128119167973088),.UNSPECIFIED.)
CURVE()
GEOMETRIC_REPRESENTATION_ITEM()
RATIONAL_B_SPLINE_CURVE((1.,1.00225826691344,1.00357310667422))
REPRESENTATION_ITEM('')
) ;
#314=(
BOUNDED_CURVE()
B_SPLINE_CURVE(2,(#16682,#16683,#16684),.UNSPECIFIED.,.F.,.F.)
B_SPLINE_CURVE_WITH_KNOTS((3,3),(0.0485234505024517,0.0613353722533853),
 .UNSPECIFIED.)
CURVE()
GEOMETRIC_REPRESENTATION_ITEM()
RATIONAL_B_SPLINE_CURVE((1.00357310769125,1.00225826778676,1.))
REPRESENTATION_ITEM('')
) ;
#317=TOROIDAL_SURFACE('',#8634,2.154,0.2) ;
#318=TOROIDAL_SURFACE('',#8827,3.3,0.2) ;
#413=B_SPLINE_SURFACE_WITH_KNOTS('',3,3,((#14885,#14886,#14887,#14888,#14889,
#14890,#14891,#14892,#14893,#14894,#14895,#14896,#14897,#14898,#14899,#14900,
#14901,#14902,#14903,#14904,#14905,#14906,#14907,#14908,#14909,#14910,#14911,
#14912,#14913,#14914,#14915,#14916,#14917,#14918,#14919,#14920,#14921,#14922,
#14923,#14924,#14925,#14926,#14927,#14928,#14929,#14930,#14931,#14932,#14933,
#14934,#14935,#14936,#14937,#14938,#14939,#14940,#14941,#14942,#14943,#14944,
#14945,#14946,#14947,#14948,#14949,#14950,#14951,#14952,#14953,#14954,#14955,
#14956,#14957,#14958,#14959,#14960,#14961,#14962,#14963,#14964,#14965,#14966,
#14967,#14968,#14969,#14970,#14971,#14972,#14973),(#14974,#14975,#14976,
#14977,#14978,#14979,#14980,#14981,#14982,#14983,#14984,#14985,#14986,#14987,
#14988,#14989,#14990,#14991,#14992,#14993,#14994,#14995,#14996,#14997,#14998,
#14999,#15000,#15001,#15002,#15003,#15004,#15005,#15006,#15007,#15008,#15009,
#15010,#15011,#15012,#15013,#15014,#15015,#15016,#15017,#15018,#15019,#15020,
#15021,#15022,#15023,#15024,#15025,#15026,#15027,#15028,#15029,#15030,#15031,
#15032,#15033,#15034,#15035,#15036,#15037,#15038,#15039,#15040,#15041,#15042,
#15043,#15044,#15045,#15046,#15047,#15048,#15049,#15050,#15051,#15052,#15053,
#15054,#15055,#15056,#15057,#15058,#15059,#15060,#15061,#15062),(#15063,
#15064,#15065,#15066,#15067,#15068,#15069,#15070,#15071,#15072,#15073,#15074,
#15075,#15076,#15077,#15078,#15079,#15080,#15081,#15082,#15083,#15084,#15085,
#15086,#15087,#15088,#15089,#15090,#15091,#15092,#15093,#15094,#15095,#15096,
#15097,#15098,#15099,#15100,#15101,#15102,#15103,#15104,#15105,#15106,#15107,
#15108,#15109,#15110,#15111,#15112,#15113,#15114,#15115,#15116,#15117,#15118,
#15119,#15120,#15121,#15122,#15123,#15124,#15125,#15126,#15127,#15128,#15129,
#15130,#15131,#15132,#15133,#15134,#15135,#15136,#15137,#15138,#15139,#15140,
#15141,#15142,#15143,#15144,#15145,#15146,#15147,#15148,#15149,#15150,#15151),
(#15152,#15153,#15154,#15155,#15156,#15157,#15158,#15159,#15160,#15161,
#15162,#15163,#15164,#15165,#15166,#15167,#15168,#15169,#15170,#15171,#15172,
#15173,#15174,#15175,#15176,#15177,#15178,#15179,#15180,#15181,#15182,#15183,
#15184,#15185,#15186,#15187,#15188,#15189,#15190,#15191,#15192,#15193,#15194,
#15195,#15196,#15197,#15198,#15199,#15200,#15201,#15202,#15203,#15204,#15205,
#15206,#15207,#15208,#15209,#15210,#15211,#15212,#15213,#15214,#15215,#15216,
#15217,#15218,#15219,#15220,#15221,#15222,#15223,#15224,#15225,#15226,#15227,
#15228,#15229,#15230,#15231,#15232,#15233,#15234,#15235,#15236,#15237,#15238,
#15239,#15240)),.UNSPECIFIED.,.F.,.F.,.F.,(4,4),(4,1,1,1,1,1,1,1,1,1,1,
1,1,1,1,1,1,1,1,1,1,1,1,1,1,1,1,1,1,1,1,1,1,1,1,1,1,1,1,1,1,1,1,1,1,1,1,
1,1,1,1,1,1,1,1,1,1,1,1,1,1,1,1,1,1,1,1,1,1,1,1,1,1,1,1,1,1,1,1,1,1,1,1,
1,1,1,4),(0.,0.0460148164544131),(8.31058692273963,9.30525837539851,10.2999298280574,
11.2946012807163,12.2892727333752,13.2839441860341,14.2786156386929,15.2732870913518,
16.2679585440107,17.2626299966696,18.2573014493285,19.2519729019874,20.2466443546463,
21.2413158073051,22.235987259964,23.2306587126229,24.2253301652818,25.2200016179407,
26.2146730705996,27.2093445232584,28.2040159759173,29.1986874285762,30.1933588812351,
31.188030333894,32.1827017865529,33.1773732392118,34.1720446918706,35.1667161445295,
36.1613875971884,37.1560590498473,38.1507305025062,39.1454019551651,40.1400734078239,
41.1347448604828,42.1294163131417,43.1240877658006,44.1187592184595,45.1134306711184,
46.1081021237773,47.1027735764361,48.097445029095,49.0921164817539,50.0867879344128,
51.0814593870717,52.0761308397306,53.0708022923895,54.0654737450483,55.0601451977072,
56.0548166503661,57.049488103025,58.0441595556839,59.0388310083428,60.0335024610017,
61.0281739136605,62.0228453663194,63.0175168189783,64.0121882716372,65.0068597242961,
66.001531176955,66.9962026296138,67.9908740822727,68.9855455349316,69.9802169875905,
70.9748884402494,71.9695598929083,72.9642313455672,73.958902798226,74.9535742508849,
75.9482457035438,76.9429171562027,77.9375886088616,78.9322600615205,79.9269315141794,
80.9216029668382,81.9162744194971,82.910945872156,83.9056173248149,84.9002887774738,
85.8949602301327,86.8896316827915,87.8843031354504,88.8789745881093,89.8736460407682,
90.8683174934271,91.862988946086,92.8576603987449,93.8523318514037),
 .UNSPECIFIED.) ;
#414=B_SPLINE_SURFACE_WITH_KNOTS('',3,3,((#15446,#15447,#15448,#15449,#15450,
#15451,#15452,#15453,#15454,#15455,#15456,#15457,#15458,#15459,#15460,#15461,
#15462,#15463,#15464,#15465,#15466,#15467,#15468,#15469,#15470,#15471,#15472,
#15473,#15474,#15475,#15476,#15477,#15478,#15479,#15480,#15481,#15482,#15483,
#15484,#15485,#15486,#15487,#15488,#15489,#15490,#15491,#15492,#15493,#15494,
#15495,#15496,#15497,#15498,#15499,#15500,#15501,#15502,#15503,#15504,#15505,
#15506,#15507,#15508,#15509,#15510,#15511,#15512,#15513,#15514,#15515,#15516,
#15517,#15518,#15519,#15520,#15521,#15522,#15523,#15524,#15525,#15526,#15527,
#15528,#15529,#15530,#15531,#15532,#15533,#15534),(#15535,#15536,#15537,
#15538,#15539,#15540,#15541,#15542,#15543,#15544,#15545,#15546,#15547,#15548,
#15549,#15550,#15551,#15552,#15553,#15554,#15555,#15556,#15557,#15558,#15559,
#15560,#15561,#15562,#15563,#15564,#15565,#15566,#15567,#15568,#15569,#15570,
#15571,#15572,#15573,#15574,#15575,#15576,#15577,#15578,#15579,#15580,#15581,
#15582,#15583,#15584,#15585,#15586,#15587,#15588,#15589,#15590,#15591,#15592,
#15593,#15594,#15595,#15596,#15597,#15598,#15599,#15600,#15601,#15602,#15603,
#15604,#15605,#15606,#15607,#15608,#15609,#15610,#15611,#15612,#15613,#15614,
#15615,#15616,#15617,#15618,#15619,#15620,#15621,#15622,#15623),(#15624,
#15625,#15626,#15627,#15628,#15629,#15630,#15631,#15632,#15633,#15634,#15635,
#15636,#15637,#15638,#15639,#15640,#15641,#15642,#15643,#15644,#15645,#15646,
#15647,#15648,#15649,#15650,#15651,#15652,#15653,#15654,#15655,#15656,#15657,
#15658,#15659,#15660,#15661,#15662,#15663,#15664,#15665,#15666,#15667,#15668,
#15669,#15670,#15671,#15672,#15673,#15674,#15675,#15676,#15677,#15678,#15679,
#15680,#15681,#15682,#15683,#15684,#15685,#15686,#15687,#15688,#15689,#15690,
#15691,#15692,#15693,#15694,#15695,#15696,#15697,#15698,#15699,#15700,#15701,
#15702,#15703,#15704,#15705,#15706,#15707,#15708,#15709,#15710,#15711,#15712),
(#15713,#15714,#15715,#15716,#15717,#15718,#15719,#15720,#15721,#15722,
#15723,#15724,#15725,#15726,#15727,#15728,#15729,#15730,#15731,#15732,#15733,
#15734,#15735,#15736,#15737,#15738,#15739,#15740,#15741,#15742,#15743,#15744,
#15745,#15746,#15747,#15748,#15749,#15750,#15751,#15752,#15753,#15754,#15755,
#15756,#15757,#15758,#15759,#15760,#15761,#15762,#15763,#15764,#15765,#15766,
#15767,#15768,#15769,#15770,#15771,#15772,#15773,#15774,#15775,#15776,#15777,
#15778,#15779,#15780,#15781,#15782,#15783,#15784,#15785,#15786,#15787,#15788,
#15789,#15790,#15791,#15792,#15793,#15794,#15795,#15796,#15797,#15798,#15799,
#15800,#15801)),.UNSPECIFIED.,.F.,.F.,.F.,(4,4),(4,1,1,1,1,1,1,1,1,1,1,
1,1,1,1,1,1,1,1,1,1,1,1,1,1,1,1,1,1,1,1,1,1,1,1,1,1,1,1,1,1,1,1,1,1,1,1,
1,1,1,1,1,1,1,1,1,1,1,1,1,1,1,1,1,1,1,1,1,1,1,1,1,1,1,1,1,1,1,1,1,1,1,1,
1,1,1,4),(0.,0.0460148164544131),(11.6154215191105,12.6100929717694,13.6047644244283,
14.5994358770872,15.594107329746,16.5887787824049,17.5834502350638,18.5781216877227,
19.5727931403816,20.5674645930405,21.5621360456994,22.5568074983582,23.5514789510171,
24.546150403676,25.5408218563349,26.5354933089938,27.5301647616527,28.5248362143116,
29.5195076669704,30.5141791196293,31.5088505722882,32.5035220249471,33.498193477606,
34.4928649302649,35.4875363829238,36.4822078355826,37.4768792882415,38.4715507409004,
39.4662221935593,40.4608936462182,41.4555650988771,42.450236551536,43.4449080041948,
44.4395794568537,45.4342509095126,46.4289223621715,47.4235938148304,48.4182652674893,
49.4129367201481,50.407608172807,51.4022796254659,52.3969510781248,53.3916225307837,
54.3862939834426,55.3809654361015,56.3756368887603,57.3703083414192,58.3649797940781,
59.359651246737,60.3543226993959,61.3489941520548,62.3436656047136,63.3383370573725,
64.3330085100314,65.3276799626903,66.3223514153492,67.3170228680081,68.311694320667,
69.3063657733259,70.3010372259847,71.2957086786436,72.2903801313025,73.2850515839614,
74.2797230366203,75.2743944892792,76.2690659419381,77.2637373945969,78.2584088472558,
79.2530802999147,80.2477517525736,81.2424232052325,82.2370946578914,83.2317661105503,
84.2264375632091,85.221109015868,86.2157804685269,87.2104519211858,88.2051233738447,
89.1997948265036,90.1944662791624,91.1891377318213,92.1838091844802,93.1784806371391,
94.173152089798,95.1678235424569,96.1624949951158,97.1571664477746),
 .UNSPECIFIED.) ;
#419=SHAPE_REPRESENTATION_RELATIONSHIP('SRR','None',#17023,#426) ;
#426=ADVANCED_BREP_SHAPE_REPRESENTATION('',(#440),#16939) ;
#433=STYLED_ITEM('',(#17067),#440) ;
#440=MANIFOLD_SOLID_BREP('ISO 4762 - M4 x 10 - 12.9',#8182) ;
#625=B_SPLINE_CURVE_WITH_KNOTS('',3,(#13724,#13725,#13726,#13727,#13728,
#13729,#13730,#13731,#13732,#13733),.UNSPECIFIED.,.F.,.F.,(4,3,3,4),(-4.09254174883839,
-3.97868581063554,-2.98401435797666,-2.06514013327809),.UNSPECIFIED.) ;
#626=B_SPLINE_CURVE_WITH_KNOTS('',3,(#13736,#13737,#13738,#13739,#13740,
#13741,#13742),.UNSPECIFIED.,.F.,.F.,(4,3,4),(0.,0.994671452658877,1.11419103802963),
 .UNSPECIFIED.) ;
#627=B_SPLINE_CURVE_WITH_KNOTS('',3,(#13747,#13748,#13749,#13750,#13751,
#13752,#13753,#13754,#13755,#13756,#13757,#13758,#13759,#13760,#13761,#13762,
#13763,#13764,#13765,#13766,#13767,#13768),.UNSPECIFIED.,.F.,.F.,(4,3,3,
3,3,3,3,4),(-10.375727056018,-9.94671452658885,-8.95204307392997,-7.95737162127108,
-6.96270016861219,-5.96802871595331,-4.97335726329442,-4.09254174883839),
 .UNSPECIFIED.) ;
#628=B_SPLINE_CURVE_WITH_KNOTS('',3,(#13769,#13770,#13771,#13772,#13773,
#13774,#13775,#13776,#13777,#13778,#13779,#13780,#13781,#13782,#13783,#13784,
#13785,#13786,#13787,#13788,#13789,#13790),.UNSPECIFIED.,.F.,.F.,(4,3,3,
3,3,3,3,4),(1.11419103802963,1.98934290531777,2.98401435797665,3.97868581063554,
4.97335726329443,5.96802871595332,6.96270016861221,7.3973763452092),
 .UNSPECIFIED.) ;
#629=B_SPLINE_CURVE_WITH_KNOTS('',3,(#13795,#13796,#13797,#13798,#13799,
#13800,#13801,#13802,#13803,#13804,#13805,#13806,#13807,#13808,#13809,#13810,
#13811,#13812,#13813,#13814,#13815,#13816),.UNSPECIFIED.,.F.,.F.,(4,3,3,
3,3,3,3,4),(-16.6589123631976,-15.9147432425422,-14.9200717898833,-13.9254003372244,
-12.9307288845655,-11.9360574319066,-10.9413859792477,-10.375727056018),
 .UNSPECIFIED.) ;
#630=B_SPLINE_CURVE_WITH_KNOTS('',3,(#13817,#13818,#13819,#13820,#13821,
#13822,#13823,#13824,#13825,#13826,#13827,#13828,#13829,#13830,#13831,#13832,
#13833,#13834,#13835,#13836,#13837,#13838),.UNSPECIFIED.,.F.,.F.,(4,3,3,
3,3,3,3,4),(7.3973763452092,7.95737162127109,8.95204307392997,9.94671452658885,
10.9413859792477,11.9360574319066,12.9307288845655,13.6805616523888),
 .UNSPECIFIED.) ;
#631=B_SPLINE_CURVE_WITH_KNOTS('',3,(#13843,#13844,#13845,#13846,#13847,
#13848,#13849,#13850,#13851,#13852,#13853,#13854,#13855,#13856,#13857,#13858,
#13859,#13860,#13861,#13862,#13863,#13864,#13865,#13866,#13867),
 .UNSPECIFIED.,.F.,.F.,(4,3,3,3,3,3,3,3,4),(-22.9420976703771,-22.8774434111544,
-21.8827719584955,-20.8881005058366,-19.8934290531777,-18.8987576005188,
-17.9040861478599,-16.9094146952011,-16.6589123631976),.UNSPECIFIED.) ;
#632=B_SPLINE_CURVE_WITH_KNOTS('',3,(#13868,#13869,#13870,#13871,#13872,
#13873,#13874,#13875,#13876,#13877,#13878,#13879,#13880,#13881,#13882,#13883,
#13884,#13885,#13886,#13887,#13888,#13889,#13890,#13891,#13892),
 .UNSPECIFIED.,.F.,.F.,(4,3,3,3,3,3,3,3,4),(13.6805616523888,13.9254003372244,
14.9200717898833,15.9147432425422,16.909414695201,17.9040861478599,18.8987576005188,
19.8934290531777,19.9637469595684),.UNSPECIFIED.) ;
#633=B_SPLINE_CURVE_WITH_KNOTS('',3,(#13897,#13898,#13899,#13900,#13901,
#13902,#13903,#13904,#13905,#13906,#13907,#13908,#13909,#13910,#13911,#13912,
#13913,#13914,#13915,#13916,#13917,#13918),.UNSPECIFIED.,.F.,.F.,(4,3,3,
3,3,3,3,4),(-29.2252829775567,-28.8454721271077,-27.8508006744488,-26.8561292217899,
-25.861457769131,-24.8667863164721,-23.8721148638132,-22.9420976703771),
 .UNSPECIFIED.) ;
#634=B_SPLINE_CURVE_WITH_KNOTS('',3,(#13919,#13920,#13921,#13922,#13923,
#13924,#13925,#13926,#13927,#13928,#13929,#13930,#13931,#13932,#13933,#13934,
#13935,#13936,#13937,#13938,#13939,#13940),.UNSPECIFIED.,.F.,.F.,(4,3,3,
3,3,3,3,4),(19.9637469595684,20.8881005058366,21.8827719584955,22.8774434111544,
23.8721148638132,24.8667863164721,25.861457769131,26.246932266748),
 .UNSPECIFIED.) ;
#635=B_SPLINE_CURVE_WITH_KNOTS('',3,(#13945,#13946,#13947,#13948,#13949,
#13950,#13951,#13952,#13953,#13954,#13955,#13956,#13957,#13958,#13959,#13960,
#13961,#13962,#13963,#13964,#13965,#13966),.UNSPECIFIED.,.F.,.F.,(4,3,3,
3,3,3,3,4),(-35.5084682847363,-34.813500843061,-33.8188293904021,-32.8241579377432,
-31.8294864850843,-30.8348150324254,-29.8401435797666,-29.2252829775567),
 .UNSPECIFIED.) ;
#636=B_SPLINE_CURVE_WITH_KNOTS('',3,(#13967,#13968,#13969,#13970,#13971,
#13972,#13973,#13974,#13975,#13976,#13977,#13978,#13979,#13980,#13981,#13982,
#13983,#13984,#13985,#13986,#13987,#13988),.UNSPECIFIED.,.F.,.F.,(4,3,3,
3,3,3,3,4),(26.246932266748,26.8561292217899,27.8508006744488,28.8454721271077,
29.8401435797665,30.8348150324254,31.8294864850843,32.5301175739276),
 .UNSPECIFIED.) ;
#637=B_SPLINE_CURVE_WITH_KNOTS('',3,(#13993,#13994,#13995,#13996,#13997,
#13998,#13999,#14000,#14001,#14002,#14003,#14004,#14005,#14006,#14007,#14008,
#14009,#14010,#14011,#14012,#14013,#14014,#14015,#14016,#14017),
 .UNSPECIFIED.,.F.,.F.,(4,3,3,3,3,3,3,3,4),(-41.7916535919159,-41.7762010116732,
-40.7815295590143,-39.7868581063554,-38.7921866536965,-37.7975152010376,
-36.8028437483788,-35.8081722957199,-35.5084682847363),.UNSPECIFIED.) ;
#638=B_SPLINE_CURVE_WITH_KNOTS('',3,(#14018,#14019,#14020,#14021,#14022,
#14023,#14024,#14025,#14026,#14027,#14028,#14029,#14030,#14031,#14032,#14033,
#14034,#14035,#14036,#14037,#14038,#14039,#14040,#14041,#14042),
 .UNSPECIFIED.,.F.,.F.,(4,3,3,3,3,3,3,3,4),(32.5301175739276,32.8241579377432,
33.8188293904021,34.813500843061,35.8081722957199,36.8028437483787,37.7975152010376,
38.7921866536965,38.8133028811071),.UNSPECIFIED.) ;
#639=B_SPLINE_CURVE_WITH_KNOTS('',3,(#14047,#14048,#14049,#14050,#14051,
#14052,#14053,#14054,#14055,#14056,#14057,#14058,#14059,#14060,#14061,#14062,
#14063,#14064,#14065,#14066,#14067,#14068),.UNSPECIFIED.,.F.,.F.,(4,3,3,
3,3,3,3,4),(-48.0748388990955,-47.7442297276265,-46.7495582749676,-45.7548868223087,
-44.7602153696498,-43.765543916991,-42.7708724643321,-41.7916535919159),
 .UNSPECIFIED.) ;
#640=B_SPLINE_CURVE_WITH_KNOTS('',3,(#14069,#14070,#14071,#14072,#14073,
#14074,#14075,#14076,#14077,#14078,#14079,#14080,#14081,#14082,#14083,#14084,
#14085,#14086,#14087,#14088,#14089,#14090),.UNSPECIFIED.,.F.,.F.,(4,3,3,
3,3,3,3,4),(38.8133028811071,39.7868581063554,40.7815295590143,41.7762010116732,
42.7708724643321,43.7655439169909,44.7602153696498,45.0964881882867),
 .UNSPECIFIED.) ;
#641=B_SPLINE_CURVE_WITH_KNOTS('',3,(#14095,#14096,#14097,#14098,#14099,
#14100,#14101,#14102,#14103,#14104,#14105,#14106,#14107,#14108,#14109,#14110,
#14111,#14112,#14113,#14114,#14115,#14116),.UNSPECIFIED.,.F.,.F.,(4,3,3,
3,3,3,3,4),(-54.3580242062751,-53.7122584435798,-52.7175869909209,-51.722915538262,
-50.7282440856032,-49.7335726329443,-48.7389011802854,-48.0748388990955),
 .UNSPECIFIED.) ;
#642=B_SPLINE_CURVE_WITH_KNOTS('',3,(#14117,#14118,#14119,#14120,#14121,
#14122,#14123,#14124,#14125,#14126,#14127,#14128,#14129,#14130,#14131,#14132,
#14133,#14134,#14135,#14136,#14137,#14138),.UNSPECIFIED.,.F.,.F.,(4,3,3,
3,3,3,3,4),(45.0964881882867,45.7548868223087,46.7495582749676,47.7442297276265,
48.7389011802854,49.7335726329443,50.7282440856031,51.3796734954663),
 .UNSPECIFIED.) ;
#643=B_SPLINE_CURVE_WITH_KNOTS('',3,(#14143,#14144,#14145,#14146,#14147,
#14148,#14149,#14150,#14151,#14152,#14153,#14154,#14155,#14156,#14157,#14158,
#14159,#14160,#14161,#14162,#14163,#14164),.UNSPECIFIED.,.F.,.F.,(4,3,3,
3,3,3,3,4),(-60.6412095134547,-59.6802871595331,-58.6856157068742,-57.6909442542154,
-56.6962728015565,-55.7016013488976,-54.7069298962387,-54.3580242062751),
 .UNSPECIFIED.) ;
#644=B_SPLINE_CURVE_WITH_KNOTS('',3,(#14165,#14166,#14167,#14168,#14169,
#14170,#14171,#14172,#14173,#14174,#14175,#14176,#14177,#14178,#14179,#14180,
#14181,#14182,#14183,#14184,#14185,#14186),.UNSPECIFIED.,.F.,.F.,(4,3,3,
3,3,3,3,4),(51.3796734954663,51.722915538262,52.7175869909209,53.7122584435798,
54.7069298962387,55.7016013488976,56.6962728015565,57.6628588026459),
 .UNSPECIFIED.) ;
#645=B_SPLINE_CURVE_WITH_KNOTS('',3,(#14191,#14192,#14193,#14194,#14195,
#14196,#14197,#14198,#14199,#14200,#14201,#14202,#14203,#14204,#14205,#14206,
#14207,#14208,#14209,#14210,#14211,#14212,#14213,#14214,#14215),
 .UNSPECIFIED.,.F.,.F.,(4,3,3,3,3,3,3,3,4),(-66.9243948206343,-66.6429873281453,
-65.6483158754864,-64.6536444228275,-63.6589729701686,-62.6643015175098,
-61.6696300648509,-60.674958612192,-60.6412095134547),.UNSPECIFIED.) ;
#646=B_SPLINE_CURVE_WITH_KNOTS('',3,(#14216,#14217,#14218,#14219,#14220,
#14221,#14222,#14223,#14224,#14225,#14226,#14227,#14228,#14229,#14230,#14231,
#14232,#14233,#14234,#14235,#14236,#14237,#14238,#14239,#14240),
 .UNSPECIFIED.,.F.,.F.,(4,3,3,3,3,3,3,3,4),(57.6628588026459,57.6909442542153,
58.6856157068742,59.6802871595331,60.674958612192,61.6696300648509,62.6643015175098,
63.6589729701687,63.9460441098255),.UNSPECIFIED.) ;
#647=B_SPLINE_CURVE_WITH_KNOTS('',3,(#14245,#14246,#14247,#14248,#14249,
#14250,#14251,#14252,#14253,#14254,#14255,#14256,#14257,#14258,#14259,#14260,
#14261,#14262,#14263,#14264,#14265,#14266),.UNSPECIFIED.,.F.,.F.,(4,3,3,
3,3,3,3,4),(-73.2075801278139,-72.6110160440986,-71.6163445914397,-70.6216731387808,
-69.627001686122,-68.6323302334631,-67.6376587808042,-66.9243948206343),
 .UNSPECIFIED.) ;
#648=B_SPLINE_CURVE_WITH_KNOTS('',3,(#14267,#14268,#14269,#14270,#14271,
#14272,#14273,#14274,#14275,#14276,#14277,#14278,#14279,#14280,#14281,#14282,
#14283,#14284,#14285,#14286,#14287,#14288),.UNSPECIFIED.,.F.,.F.,(4,3,3,
3,3,3,3,4),(63.9460441098255,64.6536444228276,65.6483158754864,66.6429873281453,
67.6376587808042,68.6323302334631,69.627001686122,70.2292294170051),
 .UNSPECIFIED.) ;
#649=B_SPLINE_CURVE_WITH_KNOTS('',3,(#14293,#14294,#14295,#14296,#14297,
#14298,#14299,#14300,#14301,#14302,#14303,#14304,#14305,#14306,#14307,#14308,
#14309,#14310,#14311,#14312,#14313,#14314),.UNSPECIFIED.,.F.,.F.,(4,3,3,
3,3,3,3,4),(-79.4907654349935,-78.5790447600519,-77.5843733073931,-76.5897018547342,
-75.5950304020753,-74.6003589494164,-73.6056874967575,-73.2075801278139),
 .UNSPECIFIED.) ;
#650=B_SPLINE_CURVE_WITH_KNOTS('',3,(#14315,#14316,#14317,#14318,#14319,
#14320,#14321,#14322,#14323,#14324,#14325,#14326,#14327,#14328,#14329,#14330,
#14331,#14332,#14333,#14334,#14335,#14336),.UNSPECIFIED.,.F.,.F.,(4,3,3,
3,3,3,3,4),(70.2292294170051,70.6216731387808,71.6163445914397,72.6110160440986,
73.6056874967575,74.6003589494164,75.5950304020753,76.5124147241847),
 .UNSPECIFIED.) ;
#651=B_SPLINE_CURVE_WITH_KNOTS('',3,(#14343,#14344,#14345,#14346,#14347,
#14348,#14349,#14350,#14351,#14352,#14353,#14354,#14355,#14356,#14357,#14358,
#14359,#14360,#14361,#14362,#14363,#14364),.UNSPECIFIED.,.F.,.F.,(4,3,3,
3,3,3,3,4),(-85.5417449286641,-84.5470734760052,-83.5524020233464,-82.5577305706875,
-81.5630591180286,-80.5683876653697,-79.5737162127108,-79.4907654349935),
 .UNSPECIFIED.) ;
#652=B_SPLINE_CURVE_WITH_KNOTS('',3,(#14365,#14366,#14367,#14368,#14369,
#14370,#14371,#14372,#14373,#14374,#14375,#14376,#14377,#14378,#14379,#14380,
#14381,#14382,#14383,#14384,#14385,#14386,#14387,#14388,#14389),
 .UNSPECIFIED.,.F.,.F.,(4,3,3,3,3,3,3,3,4),(76.5124147241847,76.5897018547341,
77.584373307393,78.5790447600519,79.5737162127108,80.5683876653697,81.5630591180286,
82.5577305706875,82.7956000313643),.UNSPECIFIED.) ;
#653=B_SPLINE_CURVE_WITH_KNOTS('',3,(#14395,#14396,#14397,#14398,#14399,
#14400,#14401,#14402),.UNSPECIFIED.,.F.,.F.,(4,1,1,1,1,4),(91.106186954104,
91.1891377318213,92.1838091844802,93.1784806371391,94.173152089798,95.0920263144966),
 .UNSPECIFIED.) ;
#654=B_SPLINE_CURVE_WITH_KNOTS('',3,(#14405,#14406,#14407,#14408,#14409,
#14410),.UNSPECIFIED.,.F.,.F.,(4,1,1,4),(91.106186954104,91.862988946086,
92.8576603987449,93.8523318514037),.UNSPECIFIED.) ;
#655=B_SPLINE_CURVE_WITH_KNOTS('',3,(#14415,#14416,#14417,#14418,#14419,
#14420,#14421,#14422,#14423,#14424),.UNSPECIFIED.,.F.,.F.,(4,1,1,1,1,1,
1,4),(84.8230016469244,85.221109015868,86.2157804685269,87.2104519211858,
88.2051233738447,89.1997948265036,90.1944662791624,91.106186954104),
 .UNSPECIFIED.) ;
#656=B_SPLINE_CURVE_WITH_KNOTS('',3,(#14425,#14426,#14427,#14428,#14429,
#14430,#14431,#14432,#14433,#14434,#14435),.UNSPECIFIED.,.F.,.F.,(4,1,1,
1,1,1,1,1,4),(84.8230016469244,84.9002887774738,85.8949602301327,86.8896316827915,
87.8843031354504,88.8789745881093,89.8736460407682,90.8683174934271,91.106186954104),
 .UNSPECIFIED.) ;
#657=B_SPLINE_CURVE_WITH_KNOTS('',3,(#14440,#14441,#14442,#14443,#14444,
#14445,#14446,#14447,#14448,#14449),.UNSPECIFIED.,.F.,.F.,(4,1,1,1,1,1,
1,4),(78.5398163397448,79.2530802999147,80.2477517525736,81.2424232052325,
82.2370946578914,83.2317661105503,84.2264375632091,84.8230016469244),
 .UNSPECIFIED.) ;
#658=B_SPLINE_CURVE_WITH_KNOTS('',3,(#14450,#14451,#14452,#14453,#14454,
#14455,#14456,#14457,#14458,#14459),.UNSPECIFIED.,.F.,.F.,(4,1,1,1,1,1,
1,4),(78.5398163397448,78.9322600615205,79.9269315141794,80.9216029668382,
81.9162744194971,82.910945872156,83.9056173248149,84.8230016469244),
 .UNSPECIFIED.) ;
#659=B_SPLINE_CURVE_WITH_KNOTS('',3,(#14464,#14465,#14466,#14467,#14468,
#14469,#14470,#14471,#14472,#14473,#14474),.UNSPECIFIED.,.F.,.F.,(4,1,1,
1,1,1,1,1,4),(72.2566310325652,72.2903801313025,73.2850515839614,74.2797230366203,
75.2743944892792,76.2690659419381,77.2637373945969,78.2584088472558,78.5398163397448),
 .UNSPECIFIED.) ;
#660=B_SPLINE_CURVE_WITH_KNOTS('',3,(#14475,#14476,#14477,#14478,#14479,
#14480,#14481,#14482,#14483,#14484),.UNSPECIFIED.,.F.,.F.,(4,1,1,1,1,1,
1,4),(72.2566310325652,72.9642313455672,73.958902798226,74.9535742508849,
75.9482457035438,76.9429171562027,77.9375886088616,78.5398163397448),
 .UNSPECIFIED.) ;
#661=B_SPLINE_CURVE_WITH_KNOTS('',3,(#14489,#14490,#14491,#14492,#14493,
#14494,#14495,#14496,#14497,#14498),.UNSPECIFIED.,.F.,.F.,(4,1,1,1,1,1,
1,4),(65.9734457253856,66.3223514153492,67.3170228680081,68.311694320667,
69.3063657733259,70.3010372259847,71.2957086786436,72.2566310325652),
 .UNSPECIFIED.) ;
#662=B_SPLINE_CURVE_WITH_KNOTS('',3,(#14499,#14500,#14501,#14502,#14503,
#14504,#14505,#14506,#14507,#14508,#14509),.UNSPECIFIED.,.F.,.F.,(4,1,1,
1,1,1,1,1,4),(65.9734457253856,66.001531176955,66.9962026296138,67.9908740822727,
68.9855455349316,69.9802169875905,70.9748884402494,71.9695598929083,72.2566310325652),
 .UNSPECIFIED.) ;
#663=B_SPLINE_CURVE_WITH_KNOTS('',3,(#14514,#14515,#14516,#14517,#14518,
#14519,#14520,#14521,#14522,#14523),.UNSPECIFIED.,.F.,.F.,(4,1,1,1,1,1,
1,4),(59.6902604182061,60.3543226993959,61.3489941520548,62.3436656047136,
63.3383370573725,64.3330085100314,65.3276799626903,65.9734457253856),
 .UNSPECIFIED.) ;
#664=B_SPLINE_CURVE_WITH_KNOTS('',3,(#14524,#14525,#14526,#14527,#14528,
#14529,#14530,#14531,#14532,#14533),.UNSPECIFIED.,.F.,.F.,(4,1,1,1,1,1,
1,4),(59.690260418206,60.0335024610017,61.0281739136605,62.0228453663194,
63.0175168189783,64.0121882716372,65.0068597242961,65.9734457253856),
 .UNSPECIFIED.) ;
#665=B_SPLINE_CURVE_WITH_KNOTS('',3,(#14538,#14539,#14540,#14541,#14542,
#14543,#14544,#14545,#14546,#14547),.UNSPECIFIED.,.F.,.F.,(4,1,1,1,1,1,
1,4),(53.4070751110265,54.3862939834426,55.3809654361015,56.3756368887603,
57.3703083414192,58.3649797940781,59.359651246737,59.6902604182061),
 .UNSPECIFIED.) ;
#666=B_SPLINE_CURVE_WITH_KNOTS('',3,(#14548,#14549,#14550,#14551,#14552,
#14553,#14554,#14555,#14556,#14557),.UNSPECIFIED.,.F.,.F.,(4,1,1,1,1,1,
1,4),(53.4070751110265,54.0654737450483,55.0601451977072,56.0548166503661,
57.049488103025,58.0441595556839,59.0388310083428,59.690260418206),
 .UNSPECIFIED.) ;
#667=B_SPLINE_CURVE_WITH_KNOTS('',3,(#14562,#14563,#14564,#14565,#14566,
#14567,#14568,#14569,#14570,#14571,#14572),.UNSPECIFIED.,.F.,.F.,(4,1,1,
1,1,1,1,1,4),(47.1238898038469,47.4235938148304,48.4182652674893,49.4129367201481,
50.407608172807,51.4022796254659,52.3969510781248,53.3916225307837,53.4070751110265),
 .UNSPECIFIED.) ;
#668=B_SPLINE_CURVE_WITH_KNOTS('',3,(#14573,#14574,#14575,#14576,#14577,
#14578,#14579,#14580,#14581,#14582),.UNSPECIFIED.,.F.,.F.,(4,1,1,1,1,1,
1,4),(47.1238898038469,48.097445029095,49.0921164817539,50.0867879344128,
51.0814593870717,52.0761308397306,53.0708022923895,53.4070751110265),
 .UNSPECIFIED.) ;
#669=B_SPLINE_CURVE_WITH_KNOTS('',3,(#14587,#14588,#14589,#14590,#14591,
#14592,#14593,#14594,#14595,#14596),.UNSPECIFIED.,.F.,.F.,(4,1,1,1,1,1,
1,4),(40.8407044966672,41.4555650988771,42.450236551536,43.4449080041948,
44.4395794568537,45.4342509095126,46.4289223621715,47.1238898038469),
 .UNSPECIFIED.) ;
#670=B_SPLINE_CURVE_WITH_KNOTS('',3,(#14597,#14598,#14599,#14600,#14601,
#14602,#14603,#14604,#14605,#14606,#14607),.UNSPECIFIED.,.F.,.F.,(4,1,1,
1,1,1,1,1,4),(40.8407044966673,41.1347448604828,42.1294163131417,43.1240877658006,
44.1187592184595,45.1134306711184,46.1081021237773,47.1027735764361,47.1238898038469),
 .UNSPECIFIED.) ;
#671=B_SPLINE_CURVE_WITH_KNOTS('',3,(#14612,#14613,#14614,#14615,#14616,
#14617,#14618,#14619,#14620,#14621),.UNSPECIFIED.,.F.,.F.,(4,1,1,1,1,1,
1,4),(34.5575191894877,35.4875363829238,36.4822078355826,37.4768792882415,
38.4715507409004,39.4662221935593,40.4608936462182,40.8407044966672),
 .UNSPECIFIED.) ;
#672=B_SPLINE_CURVE_WITH_KNOTS('',3,(#14622,#14623,#14624,#14625,#14626,
#14627,#14628,#14629,#14630,#14631),.UNSPECIFIED.,.F.,.F.,(4,1,1,1,1,1,
1,4),(34.5575191894877,35.1667161445295,36.1613875971884,37.1560590498473,
38.1507305025062,39.1454019551651,40.1400734078239,40.8407044966673),
 .UNSPECIFIED.) ;
#673=B_SPLINE_CURVE_WITH_KNOTS('',3,(#14636,#14637,#14638,#14639,#14640,
#14641,#14642,#14643,#14644,#14645,#14646),.UNSPECIFIED.,.F.,.F.,(4,1,1,
1,1,1,1,1,4),(28.2743338823081,28.5248362143116,29.5195076669704,30.5141791196293,
31.5088505722882,32.5035220249471,33.498193477606,34.4928649302649,34.5575191894877),
 .UNSPECIFIED.) ;
#674=B_SPLINE_CURVE_WITH_KNOTS('',3,(#14647,#14648,#14649,#14650,#14651,
#14652,#14653,#14654,#14655,#14656),.UNSPECIFIED.,.F.,.F.,(4,1,1,1,1,1,
1,4),(28.2743338823081,29.1986874285762,30.1933588812351,31.188030333894,
32.1827017865529,33.1773732392118,34.1720446918706,34.5575191894877),
 .UNSPECIFIED.) ;
#675=B_SPLINE_CURVE_WITH_KNOTS('',3,(#14661,#14662,#14663,#14664,#14665,
#14666,#14667,#14668,#14669,#14670),.UNSPECIFIED.,.F.,.F.,(4,1,1,1,1,1,
1,4),(21.9911485751285,22.5568074983582,23.5514789510171,24.546150403676,
25.5408218563349,26.5354933089938,27.5301647616527,28.2743338823081),
 .UNSPECIFIED.) ;
#676=B_SPLINE_CURVE_WITH_KNOTS('',3,(#14671,#14672,#14673,#14674,#14675,
#14676,#14677,#14678,#14679,#14680,#14681),.UNSPECIFIED.,.F.,.F.,(4,1,1,
1,1,1,1,1,4),(21.9911485751285,22.235987259964,23.2306587126229,24.2253301652818,
25.2200016179407,26.2146730705996,27.2093445232584,28.2040159759173,28.2743338823081),
 .UNSPECIFIED.) ;
#677=B_SPLINE_CURVE_WITH_KNOTS('',3,(#14686,#14687,#14688,#14689,#14690,
#14691,#14692,#14693,#14694,#14695),.UNSPECIFIED.,.F.,.F.,(4,1,1,1,1,1,
1,4),(15.7079632679489,16.5887787824049,17.5834502350638,18.5781216877227,
19.5727931403816,20.5674645930405,21.5621360456994,21.9911485751285),
 .UNSPECIFIED.) ;
#678=B_SPLINE_CURVE_WITH_KNOTS('',3,(#14696,#14697,#14698,#14699,#14700,
#14701,#14702,#14703,#14704,#14705),.UNSPECIFIED.,.F.,.F.,(4,1,1,1,1,1,
1,4),(15.7079632679489,16.2679585440107,17.2626299966696,18.2573014493285,
19.2519729019874,20.2466443546463,21.2413158073051,21.9911485751285),
 .UNSPECIFIED.) ;
#679=B_SPLINE_CURVE_WITH_KNOTS('',3,(#14707,#14708,#14709,#14710,#14711,
#14712,#14713,#14714,#14715,#14716,#14717,#14718,#14719,#14720,#14721,#14722,
#14723,#14724,#14725,#14726,#14727,#14728,#14729,#14730,#14731,#14732,#14733,
#14734,#14735,#14736,#14737,#14738,#14739,#14740,#14741,#14742,#14743,#14744,
#14745,#14746,#14747,#14748,#14749,#14750,#14751,#14752,#14753,#14754,#14755,
#14756,#14757,#14758,#14759,#14760,#14761,#14762,#14763,#14764,#14765,#14766,
#14767,#14768,#14769,#14770,#14771,#14772,#14773,#14774,#14775,#14776,#14777,
#14778,#14779,#14780,#14781,#14782,#14783,#14784,#14785,#14786,#14787,#14788,
#14789,#14790,#14791,#14792,#14793,#14794),.UNSPECIFIED.,.F.,.F.,(4,3,3,
3,3,3,3,3,3,3,3,3,3,3,3,3,3,3,3,3,3,3,3,3,3,3,3,3,3,4),(-0.366397579005862,
-0.354400153901985,-0.336404777063956,-0.325308561006329,-0.321425114196814,
-0.302615912560535,-0.288115700084732,-0.282369417309185,-0.278676253632104,
-0.259267773940829,-0.239450435117437,-0.226241379526605,-0.219675125726992,
-0.215147934128903,-0.211940642009688,-0.191508203259365,-0.186614212754108,
-0.166896800453023,-0.156170429838319,-0.146894080558608,-0.143763204851242,
-0.123283757624856,-0.102374268823611,-0.0813088122791208,-0.0759017170823301,
-0.0722481990532672,-0.0506067082153849,-0.0289141439014962,-0.00768477071724965,
0.),.UNSPECIFIED.) ;
#680=B_SPLINE_CURVE_WITH_KNOTS('',3,(#14797,#14798,#14799,#14800,#14801,
#14802,#14803,#14804,#14805,#14806,#14807,#14808,#14809,#14810,#14811,#14812,
#14813,#14814,#14815,#14816,#14817,#14818,#14819,#14820,#14821,#14822,#14823,
#14824,#14825,#14826,#14827,#14828,#14829,#14830,#14831,#14832,#14833,#14834,
#14835,#14836,#14837,#14838,#14839,#14840,#14841,#14842,#14843,#14844,#14845,
#14846,#14847,#14848,#14849,#14850,#14851,#14852,#14853,#14854,#14855,#14856,
#14857,#14858,#14859,#14860,#14861,#14862,#14863,#14864,#14865,#14866,#14867,
#14868,#14869,#14870,#14871,#14872,#14873,#14874,#14875,#14876,#14877,#14878,
#14879,#14880,#14881,#14882,#14883,#14884),.UNSPECIFIED.,.F.,.F.,(4,3,3,
3,3,3,3,3,3,3,3,3,3,3,3,3,3,3,3,3,3,3,3,3,3,3,3,3,3,4),(-0.364629307890639,
-0.349849466571909,-0.328248388013126,-0.317414684226437,-0.313033716262076,
-0.291718379827004,-0.275966596123573,-0.26769149370129,-0.263902447125792,
-0.26027159190815,-0.239539956910309,-0.219314376336061,-0.205911809801935,
-0.194395827041001,-0.191067917075939,-0.171483017238108,-0.165704110199559,
-0.144723738467068,-0.135144345214647,-0.126400867612846,-0.123094476845862,
-0.103639598986686,-0.0842677857508656,-0.0652966313372813,-0.0619884758863919,
-0.0584739564360926,-0.0398922435233024,-0.0216481816196747,-0.00398472010826969,
0.),.UNSPECIFIED.) ;
#681=B_SPLINE_CURVE_WITH_KNOTS('',3,(#15241,#15242,#15243,#15244),
 .UNSPECIFIED.,.F.,.F.,(4,4),(82.7956000313643,83.4766047953861),
 .UNSPECIFIED.) ;
#682=B_SPLINE_CURVE_WITH_KNOTS('',3,(#15246,#15247,#15248,#15249,#15250,
#15251,#15252,#15253,#15254,#15255,#15256,#15257,#15258,#15259,#15260,#15261,
#15262,#15263,#15264,#15265,#15266,#15267,#15268,#15269,#15270,#15271,#15272,
#15273,#15274,#15275,#15276,#15277,#15278,#15279,#15280,#15281,#15282,#15283,
#15284,#15285,#15286,#15287,#15288,#15289,#15290,#15291,#15292,#15293,#15294,
#15295,#15296,#15297,#15298,#15299,#15300,#15301,#15302,#15303,#15304,#15305,
#15306,#15307,#15308,#15309,#15310,#15311,#15312,#15313,#15314,#15315,#15316,
#15317,#15318,#15319,#15320,#15321,#15322,#15323,#15324,#15325,#15326,#15327,
#15328,#15329,#15330,#15331,#15332,#15333),.UNSPECIFIED.,.F.,.F.,(4,3,3,
3,3,3,3,3,3,3,3,3,3,3,3,3,3,3,3,3,3,3,3,3,3,3,3,3,3,4),(-0.366397579005832,
-0.35440015390196,-0.336404774950202,-0.325308556551589,-0.321425108353319,
-0.302615905227926,-0.288115693668699,-0.282369381594845,-0.278676239117541,
-0.259267757976344,-0.239450419326581,-0.226241367683462,-0.219675101906396,
-0.215147723883162,-0.211940603206927,-0.19150816459754,-0.186614212754105,
-0.166896799655008,-0.15617042880848,-0.146894076502295,-0.14376319718546,
-0.123283748791081,-0.102374258882692,-0.0813088023174796,-0.0759017003095587,
-0.0722481957683859,-0.0506067042383249,-0.0289141405258821,-0.00768477040946941,
0.),.UNSPECIFIED.) ;
#683=B_SPLINE_CURVE_WITH_KNOTS('',3,(#15334,#15335,#15336,#15337,#15338,
#15339,#15340,#15341,#15342),.UNSPECIFIED.,.F.,.F.,(4,1,1,1,1,1,4),(10.3757270560177,
11.2946012807163,12.2892727333752,13.2839441860341,14.2786156386929,15.2732870913518,
15.7079632679489),.UNSPECIFIED.) ;
#684=B_SPLINE_CURVE_WITH_KNOTS('',3,(#15347,#15348,#15349,#15350,#15351,
#15352,#15353,#15354,#15355,#15356,#15357,#15358,#15359,#15360,#15361,#15362,
#15363,#15364,#15365,#15366,#15367,#15368,#15369,#15370,#15371,#15372,#15373,
#15374,#15375,#15376,#15377,#15378,#15379,#15380,#15381,#15382,#15383,#15384,
#15385,#15386,#15387,#15388,#15389,#15390,#15391,#15392,#15393,#15394,#15395,
#15396,#15397,#15398,#15399,#15400,#15401,#15402,#15403,#15404,#15405,#15406,
#15407,#15408,#15409,#15410,#15411,#15412,#15413,#15414,#15415,#15416,#15417,
#15418,#15419,#15420,#15421,#15422,#15423,#15424,#15425,#15426,#15427,#15428,
#15429,#15430,#15431,#15432,#15433,#15434),.UNSPECIFIED.,.F.,.F.,(4,3,3,
3,3,3,3,3,3,3,3,3,3,3,3,3,3,3,3,3,3,3,3,3,3,3,3,3,3,4),(-0.364629307890559,
-0.349849466571842,-0.328248388005598,-0.317414684778512,-0.313033717426747,
-0.291718381011116,-0.275966597159668,-0.267691495007892,-0.263902448445838,
-0.260271592580404,-0.239539957901017,-0.219314379339481,-0.205911812054494,
-0.194395830861808,-0.191067922191916,-0.171483024299037,-0.165704110199532,
-0.144723710840863,-0.135144314569244,-0.126400708769428,-0.123094450949365,
-0.103639573299063,-0.0842677588660923,-0.0652966020700892,-0.0619884278297192,
-0.0584739451235707,-0.0398922301008105,-0.0216481651996582,-0.00398470002455966,
0.),.UNSPECIFIED.) ;
#685=B_SPLINE_CURVE_WITH_KNOTS('',3,(#15438,#15439,#15440,#15441,#15442,
#15443,#15444,#15445),.UNSPECIFIED.,.F.,.F.,(4,1,1,1,1,4),(11.6154215191105,
12.6100929717694,13.6047644244283,14.5994358770872,15.594107329746,15.7079632679489),
 .UNSPECIFIED.) ;
#729=FACE_BOUND('',#1827,.T.) ;
#730=FACE_BOUND('',#1942,.T.) ;
#836=PLANE('',#8627) ;
#837=PLANE('',#8629) ;
#838=PLANE('',#8639) ;
#839=PLANE('',#8643) ;
#840=PLANE('',#8644) ;
#841=PLANE('',#8645) ;
#842=PLANE('',#8647) ;
#843=PLANE('',#8722) ;
#844=PLANE('',#8723) ;
#845=PLANE('',#8724) ;
#846=PLANE('',#8725) ;
#847=PLANE('',#8726) ;
#848=PLANE('',#8727) ;
#849=PLANE('',#8728) ;
#850=PLANE('',#8729) ;
#851=PLANE('',#8730) ;
#852=PLANE('',#8731) ;
#853=PLANE('',#8732) ;
#854=PLANE('',#8733) ;
#855=PLANE('',#8734) ;
#856=PLANE('',#8735) ;
#857=PLANE('',#8736) ;
#858=PLANE('',#8737) ;
#859=PLANE('',#8738) ;
#860=PLANE('',#8739) ;
#861=PLANE('',#8740) ;
#862=PLANE('',#8741) ;
#863=PLANE('',#8742) ;
#864=PLANE('',#8743) ;
#865=PLANE('',#8744) ;
#866=PLANE('',#8745) ;
#867=PLANE('',#8746) ;
#868=PLANE('',#8747) ;
#869=PLANE('',#8748) ;
#870=PLANE('',#8749) ;
#871=PLANE('',#8750) ;
#872=PLANE('',#8751) ;
#873=PLANE('',#8752) ;
#874=PLANE('',#8753) ;
#875=PLANE('',#8754) ;
#876=PLANE('',#8755) ;
#877=PLANE('',#8756) ;
#878=PLANE('',#8757) ;
#879=PLANE('',#8758) ;
#880=PLANE('',#8759) ;
#881=PLANE('',#8760) ;
#882=PLANE('',#8761) ;
#883=PLANE('',#8762) ;
#884=PLANE('',#8763) ;
#885=PLANE('',#8764) ;
#886=PLANE('',#8765) ;
#887=PLANE('',#8766) ;
#888=PLANE('',#8767) ;
#889=PLANE('',#8768) ;
#890=PLANE('',#8769) ;
#891=PLANE('',#8770) ;
#892=PLANE('',#8771) ;
#893=PLANE('',#8772) ;
#894=PLANE('',#8773) ;
#895=PLANE('',#8774) ;
#896=PLANE('',#8775) ;
#897=PLANE('',#8776) ;
#898=PLANE('',#8777) ;
#899=PLANE('',#8778) ;
#900=PLANE('',#8779) ;
#901=PLANE('',#8780) ;
#902=PLANE('',#8781) ;
#903=PLANE('',#8782) ;
#904=PLANE('',#8783) ;
#905=PLANE('',#8784) ;
#906=PLANE('',#8785) ;
#907=PLANE('',#8786) ;
#908=PLANE('',#8787) ;
#909=PLANE('',#8788) ;
#910=PLANE('',#8789) ;
#911=PLANE('',#8790) ;
#912=PLANE('',#8791) ;
#913=PLANE('',#8792) ;
#914=PLANE('',#8793) ;
#915=PLANE('',#8794) ;
#916=PLANE('',#8795) ;
#917=PLANE('',#8796) ;
#918=PLANE('',#8797) ;
#919=PLANE('',#8798) ;
#920=PLANE('',#8799) ;
#921=PLANE('',#8800) ;
#922=PLANE('',#8801) ;
#923=PLANE('',#8802) ;
#924=PLANE('',#8803) ;
#925=PLANE('',#8804) ;
#926=PLANE('',#8805) ;
#927=PLANE('',#8806) ;
#928=PLANE('',#8807) ;
#929=PLANE('',#8808) ;
#930=PLANE('',#8809) ;
#931=PLANE('',#8810) ;
#932=PLANE('',#8811) ;
#933=PLANE('',#8812) ;
#934=PLANE('',#8813) ;
#935=PLANE('',#8814) ;
#936=PLANE('',#8815) ;
#937=PLANE('',#8816) ;
#938=PLANE('',#8817) ;
#939=PLANE('',#8818) ;
#940=PLANE('',#8819) ;
#941=PLANE('',#8820) ;
#942=PLANE('',#8821) ;
#943=PLANE('',#8822) ;
#944=PLANE('',#8823) ;
#945=PLANE('',#8824) ;
#946=PLANE('',#8825) ;
#947=PLANE('',#8826) ;
#948=PLANE('',#8831) ;
#949=PLANE('',#8852) ;
#950=PLANE('',#8853) ;
#951=PLANE('',#8854) ;
#952=PLANE('',#8855) ;
#953=PLANE('',#8856) ;
#954=PLANE('',#8857) ;
#955=PLANE('',#8858) ;
#956=PLANE('',#8859) ;
#957=PLANE('',#8860) ;
#958=PLANE('',#8861) ;
#959=PLANE('',#8863) ;
#960=PLANE('',#8865) ;
#961=PLANE('',#8867) ;
#962=PLANE('',#8869) ;
#963=PLANE('',#8871) ;
#964=PLANE('',#8874) ;
#965=PLANE('',#8875) ;
#966=PLANE('',#8876) ;
#1018=CYLINDRICAL_SURFACE('',#8597,1.954) ;
#1019=CYLINDRICAL_SURFACE('',#8599,1.954) ;
#1020=CYLINDRICAL_SURFACE('',#8600,1.954) ;
#1021=CYLINDRICAL_SURFACE('',#8601,1.954) ;
#1022=CYLINDRICAL_SURFACE('',#8602,1.954) ;
#1023=CYLINDRICAL_SURFACE('',#8603,1.954) ;
#1024=CYLINDRICAL_SURFACE('',#8604,1.954) ;
#1025=CYLINDRICAL_SURFACE('',#8605,1.954) ;
#1026=CYLINDRICAL_SURFACE('',#8606,1.954) ;
#1027=CYLINDRICAL_SURFACE('',#8607,1.954) ;
#1028=CYLINDRICAL_SURFACE('',#8608,1.954) ;
#1029=CYLINDRICAL_SURFACE('',#8609,1.954) ;
#1030=CYLINDRICAL_SURFACE('',#8610,1.954) ;
#1031=CYLINDRICAL_SURFACE('',#8611,1.954) ;
#1032=CYLINDRICAL_SURFACE('',#8613,1.5555) ;
#1033=CYLINDRICAL_SURFACE('',#8615,1.5555) ;
#1034=CYLINDRICAL_SURFACE('',#8616,1.5555) ;
#1035=CYLINDRICAL_SURFACE('',#8617,1.5555) ;
#1036=CYLINDRICAL_SURFACE('',#8618,1.5555) ;
#1037=CYLINDRICAL_SURFACE('',#8619,1.5555) ;
#1038=CYLINDRICAL_SURFACE('',#8620,1.5555) ;
#1039=CYLINDRICAL_SURFACE('',#8621,1.5555) ;
#1040=CYLINDRICAL_SURFACE('',#8622,1.5555) ;
#1041=CYLINDRICAL_SURFACE('',#8623,1.5555) ;
#1042=CYLINDRICAL_SURFACE('',#8624,1.5555) ;
#1043=CYLINDRICAL_SURFACE('',#8625,1.5555) ;
#1044=CYLINDRICAL_SURFACE('',#8626,1.5555) ;
#1045=CYLINDRICAL_SURFACE('',#8633,1.5555) ;
#1046=CYLINDRICAL_SURFACE('',#8637,1.954) ;
#1047=CYLINDRICAL_SURFACE('',#8648,3.5) ;
#1048=CYLINDRICAL_SURFACE('',#8840,1.68205080756887) ;
#1049=CYLINDRICAL_SURFACE('',#8842,1.68205080756887) ;
#1050=CYLINDRICAL_SURFACE('',#8844,1.68205080756887) ;
#1051=CYLINDRICAL_SURFACE('',#8846,1.68205080756887) ;
#1052=CYLINDRICAL_SURFACE('',#8848,1.68205080756887) ;
#1053=CYLINDRICAL_SURFACE('',#8850,1.68205080756887) ;
#1307=FACE_OUTER_BOUND('',#1792,.T.) ;
#1308=FACE_OUTER_BOUND('',#1793,.T.) ;
#1309=FACE_OUTER_BOUND('',#1794,.T.) ;
#1310=FACE_OUTER_BOUND('',#1795,.T.) ;
#1311=FACE_OUTER_BOUND('',#1796,.T.) ;
#1312=FACE_OUTER_BOUND('',#1797,.T.) ;
#1313=FACE_OUTER_BOUND('',#1798,.T.) ;
#1314=FACE_OUTER_BOUND('',#1799,.T.) ;
#1315=FACE_OUTER_BOUND('',#1800,.T.) ;
#1316=FACE_OUTER_BOUND('',#1801,.T.) ;
#1317=FACE_OUTER_BOUND('',#1802,.T.) ;
#1318=FACE_OUTER_BOUND('',#1803,.T.) ;
#1319=FACE_OUTER_BOUND('',#1804,.T.) ;
#1320=FACE_OUTER_BOUND('',#1805,.T.) ;
#1321=FACE_OUTER_BOUND('',#1806,.T.) ;
#1322=FACE_OUTER_BOUND('',#1807,.T.) ;
#1323=FACE_OUTER_BOUND('',#1808,.T.) ;
#1324=FACE_OUTER_BOUND('',#1809,.T.) ;
#1325=FACE_OUTER_BOUND('',#1810,.T.) ;
#1326=FACE_OUTER_BOUND('',#1811,.T.) ;
#1327=FACE_OUTER_BOUND('',#1812,.T.) ;
#1328=FACE_OUTER_BOUND('',#1813,.T.) ;
#1329=FACE_OUTER_BOUND('',#1814,.T.) ;
#1330=FACE_OUTER_BOUND('',#1815,.T.) ;
#1331=FACE_OUTER_BOUND('',#1816,.T.) ;
#1332=FACE_OUTER_BOUND('',#1817,.T.) ;
#1333=FACE_OUTER_BOUND('',#1818,.T.) ;
#1334=FACE_OUTER_BOUND('',#1819,.T.) ;
#1335=FACE_OUTER_BOUND('',#1820,.T.) ;
#1336=FACE_OUTER_BOUND('',#1821,.T.) ;
#1337=FACE_OUTER_BOUND('',#1822,.T.) ;
#1338=FACE_OUTER_BOUND('',#1823,.T.) ;
#1339=FACE_OUTER_BOUND('',#1824,.T.) ;
#1340=FACE_OUTER_BOUND('',#1825,.T.) ;
#1341=FACE_OUTER_BOUND('',#1826,.T.) ;
#1342=FACE_OUTER_BOUND('',#1828,.T.) ;
#1343=FACE_OUTER_BOUND('',#1829,.T.) ;
#1344=FACE_OUTER_BOUND('',#1830,.T.) ;
#1345=FACE_OUTER_BOUND('',#1831,.T.) ;
#1346=FACE_OUTER_BOUND('',#1832,.T.) ;
#1347=FACE_OUTER_BOUND('',#1833,.T.) ;
#1348=FACE_OUTER_BOUND('',#1834,.T.) ;
#1349=FACE_OUTER_BOUND('',#1835,.T.) ;
#1350=FACE_OUTER_BOUND('',#1836,.T.) ;
#1351=FACE_OUTER_BOUND('',#1837,.T.) ;
#1352=FACE_OUTER_BOUND('',#1838,.T.) ;
#1353=FACE_OUTER_BOUND('',#1839,.T.) ;
#1354=FACE_OUTER_BOUND('',#1840,.T.) ;
#1355=FACE_OUTER_BOUND('',#1841,.T.) ;
#1356=FACE_OUTER_BOUND('',#1842,.T.) ;
#1357=FACE_OUTER_BOUND('',#1843,.T.) ;
#1358=FACE_OUTER_BOUND('',#1844,.T.) ;
#1359=FACE_OUTER_BOUND('',#1845,.T.) ;
#1360=FACE_OUTER_BOUND('',#1846,.T.) ;
#1361=FACE_OUTER_BOUND('',#1847,.T.) ;
#1362=FACE_OUTER_BOUND('',#1848,.T.) ;
#1363=FACE_OUTER_BOUND('',#1849,.T.) ;
#1364=FACE_OUTER_BOUND('',#1850,.T.) ;
#1365=FACE_OUTER_BOUND('',#1851,.T.) ;
#1366=FACE_OUTER_BOUND('',#1852,.T.) ;
#1367=FACE_OUTER_BOUND('',#1853,.T.) ;
#1368=FACE_OUTER_BOUND('',#1854,.T.) ;
#1369=FACE_OUTER_BOUND('',#1855,.T.) ;
#1370=FACE_OUTER_BOUND('',#1856,.T.) ;
#1371=FACE_OUTER_BOUND('',#1857,.T.) ;
#1372=FACE_OUTER_BOUND('',#1858,.T.) ;
#1373=FACE_OUTER_BOUND('',#1859,.T.) ;
#1374=FACE_OUTER_BOUND('',#1860,.T.) ;
#1375=FACE_OUTER_BOUND('',#1861,.T.) ;
#1376=FACE_OUTER_BOUND('',#1862,.T.) ;
#1377=FACE_OUTER_BOUND('',#1863,.T.) ;
#1378=FACE_OUTER_BOUND('',#1864,.T.) ;
#1379=FACE_OUTER_BOUND('',#1865,.T.) ;
#1380=FACE_OUTER_BOUND('',#1866,.T.) ;
#1381=FACE_OUTER_BOUND('',#1867,.T.) ;
#1382=FACE_OUTER_BOUND('',#1868,.T.) ;
#1383=FACE_OUTER_BOUND('',#1869,.T.) ;
#1384=FACE_OUTER_BOUND('',#1870,.T.) ;
#1385=FACE_OUTER_BOUND('',#1871,.T.) ;
#1386=FACE_OUTER_BOUND('',#1872,.T.) ;
#1387=FACE_OUTER_BOUND('',#1873,.T.) ;
#1388=FACE_OUTER_BOUND('',#1874,.T.) ;
#1389=FACE_OUTER_BOUND('',#1875,.T.) ;
#1390=FACE_OUTER_BOUND('',#1876,.T.) ;
#1391=FACE_OUTER_BOUND('',#1877,.T.) ;
#1392=FACE_OUTER_BOUND('',#1878,.T.) ;
#1393=FACE_OUTER_BOUND('',#1879,.T.) ;
#1394=FACE_OUTER_BOUND('',#1880,.T.) ;
#1395=FACE_OUTER_BOUND('',#1881,.T.) ;
#1396=FACE_OUTER_BOUND('',#1882,.T.) ;
#1397=FACE_OUTER_BOUND('',#1883,.T.) ;
#1398=FACE_OUTER_BOUND('',#1884,.T.) ;
#1399=FACE_OUTER_BOUND('',#1885,.T.) ;
#1400=FACE_OUTER_BOUND('',#1886,.T.) ;
#1401=FACE_OUTER_BOUND('',#1887,.T.) ;
#1402=FACE_OUTER_BOUND('',#1888,.T.) ;
#1403=FACE_OUTER_BOUND('',#1889,.T.) ;
#1404=FACE_OUTER_BOUND('',#1890,.T.) ;
#1405=FACE_OUTER_BOUND('',#1891,.T.) ;
#1406=FACE_OUTER_BOUND('',#1892,.T.) ;
#1407=FACE_OUTER_BOUND('',#1893,.T.) ;
#1408=FACE_OUTER_BOUND('',#1894,.T.) ;
#1409=FACE_OUTER_BOUND('',#1895,.T.) ;
#1410=FACE_OUTER_BOUND('',#1896,.T.) ;
#1411=FACE_OUTER_BOUND('',#1897,.T.) ;
#1412=FACE_OUTER_BOUND('',#1898,.T.) ;
#1413=FACE_OUTER_BOUND('',#1899,.T.) ;
#1414=FACE_OUTER_BOUND('',#1900,.T.) ;
#1415=FACE_OUTER_BOUND('',#1901,.T.) ;
#1416=FACE_OUTER_BOUND('',#1902,.T.) ;
#1417=FACE_OUTER_BOUND('',#1903,.T.) ;
#1418=FACE_OUTER_BOUND('',#1904,.T.) ;
#1419=FACE_OUTER_BOUND('',#1905,.T.) ;
#1420=FACE_OUTER_BOUND('',#1906,.T.) ;
#1421=FACE_OUTER_BOUND('',#1907,.T.) ;
#1422=FACE_OUTER_BOUND('',#1908,.T.) ;
#1423=FACE_OUTER_BOUND('',#1909,.T.) ;
#1424=FACE_OUTER_BOUND('',#1910,.T.) ;
#1425=FACE_OUTER_BOUND('',#1911,.T.) ;
#1426=FACE_OUTER_BOUND('',#1912,.T.) ;
#1427=FACE_OUTER_BOUND('',#1913,.T.) ;
#1428=FACE_OUTER_BOUND('',#1914,.T.) ;
#1429=FACE_OUTER_BOUND('',#1915,.T.) ;
#1430=FACE_OUTER_BOUND('',#1916,.T.) ;
#1431=FACE_OUTER_BOUND('',#1917,.T.) ;
#1432=FACE_OUTER_BOUND('',#1918,.T.) ;
#1433=FACE_OUTER_BOUND('',#1919,.T.) ;
#1434=FACE_OUTER_BOUND('',#1920,.T.) ;
#1435=FACE_OUTER_BOUND('',#1921,.T.) ;
#1436=FACE_OUTER_BOUND('',#1922,.T.) ;
#1437=FACE_OUTER_BOUND('',#1923,.T.) ;
#1438=FACE_OUTER_BOUND('',#1924,.T.) ;
#1439=FACE_OUTER_BOUND('',#1925,.T.) ;
#1440=FACE_OUTER_BOUND('',#1926,.T.) ;
#1441=FACE_OUTER_BOUND('',#1927,.T.) ;
#1442=FACE_OUTER_BOUND('',#1928,.T.) ;
#1443=FACE_OUTER_BOUND('',#1929,.T.) ;
#1444=FACE_OUTER_BOUND('',#1930,.T.) ;
#1445=FACE_OUTER_BOUND('',#1931,.T.) ;
#1446=FACE_OUTER_BOUND('',#1932,.T.) ;
#1447=FACE_OUTER_BOUND('',#1933,.T.) ;
#1448=FACE_OUTER_BOUND('',#1934,.T.) ;
#1449=FACE_OUTER_BOUND('',#1935,.T.) ;
#1450=FACE_OUTER_BOUND('',#1936,.T.) ;
#1451=FACE_OUTER_BOUND('',#1937,.T.) ;
#1452=FACE_OUTER_BOUND('',#1938,.T.) ;
#1453=FACE_OUTER_BOUND('',#1939,.T.) ;
#1454=FACE_OUTER_BOUND('',#1940,.T.) ;
#1455=FACE_OUTER_BOUND('',#1941,.T.) ;
#1456=FACE_OUTER_BOUND('',#1943,.T.) ;
#1457=FACE_OUTER_BOUND('',#1944,.T.) ;
#1458=FACE_OUTER_BOUND('',#1945,.T.) ;
#1459=FACE_OUTER_BOUND('',#1946,.T.) ;
#1460=FACE_OUTER_BOUND('',#1947,.T.) ;
#1461=FACE_OUTER_BOUND('',#1948,.T.) ;
#1462=FACE_OUTER_BOUND('',#1949,.T.) ;
#1463=FACE_OUTER_BOUND('',#1950,.T.) ;
#1464=FACE_OUTER_BOUND('',#1951,.T.) ;
#1465=FACE_OUTER_BOUND('',#1952,.T.) ;
#1466=FACE_OUTER_BOUND('',#1953,.T.) ;
#1467=FACE_OUTER_BOUND('',#1954,.T.) ;
#1468=FACE_OUTER_BOUND('',#1955,.T.) ;
#1469=FACE_OUTER_BOUND('',#1956,.T.) ;
#1470=FACE_OUTER_BOUND('',#1957,.T.) ;
#1471=FACE_OUTER_BOUND('',#1958,.T.) ;
#1472=FACE_OUTER_BOUND('',#1959,.T.) ;
#1473=FACE_OUTER_BOUND('',#1960,.T.) ;
#1474=FACE_OUTER_BOUND('',#1961,.T.) ;
#1475=FACE_OUTER_BOUND('',#1962,.T.) ;
#1476=FACE_OUTER_BOUND('',#1963,.T.) ;
#1477=FACE_OUTER_BOUND('',#1964,.T.) ;
#1478=FACE_OUTER_BOUND('',#1965,.T.) ;
#1479=FACE_OUTER_BOUND('',#1966,.T.) ;
#1480=FACE_OUTER_BOUND('',#1967,.T.) ;
#1481=FACE_OUTER_BOUND('',#1968,.T.) ;
#1792=EDGE_LOOP('',(#6627,#6628,#6629,#6630)) ;
#1793=EDGE_LOOP('',(#6631,#6632,#6633,#6634)) ;
#1794=EDGE_LOOP('',(#6635,#6636,#6637,#6638)) ;
#1795=EDGE_LOOP('',(#6639,#6640,#6641,#6642)) ;
#1796=EDGE_LOOP('',(#6643,#6644,#6645,#6646)) ;
#1797=EDGE_LOOP('',(#6647,#6648,#6649,#6650)) ;
#1798=EDGE_LOOP('',(#6651,#6652,#6653,#6654)) ;
#1799=EDGE_LOOP('',(#6655,#6656,#6657,#6658)) ;
#1800=EDGE_LOOP('',(#6659,#6660,#6661,#6662)) ;
#1801=EDGE_LOOP('',(#6663,#6664,#6665,#6666)) ;
#1802=EDGE_LOOP('',(#6667,#6668,#6669,#6670)) ;
#1803=EDGE_LOOP('',(#6671,#6672,#6673,#6674)) ;
#1804=EDGE_LOOP('',(#6675,#6676,#6677,#6678)) ;
#1805=EDGE_LOOP('',(#6679,#6680,#6681,#6682,#6683)) ;
#1806=EDGE_LOOP('',(#6684,#6685,#6686,#6687)) ;
#1807=EDGE_LOOP('',(#6688,#6689,#6690,#6691)) ;
#1808=EDGE_LOOP('',(#6692,#6693,#6694,#6695)) ;
#1809=EDGE_LOOP('',(#6696,#6697,#6698,#6699)) ;
#1810=EDGE_LOOP('',(#6700,#6701,#6702,#6703)) ;
#1811=EDGE_LOOP('',(#6704,#6705,#6706,#6707)) ;
#1812=EDGE_LOOP('',(#6708,#6709,#6710,#6711)) ;
#1813=EDGE_LOOP('',(#6712,#6713,#6714,#6715)) ;
#1814=EDGE_LOOP('',(#6716,#6717,#6718,#6719)) ;
#1815=EDGE_LOOP('',(#6720,#6721,#6722,#6723)) ;
#1816=EDGE_LOOP('',(#6724,#6725,#6726,#6727)) ;
#1817=EDGE_LOOP('',(#6728,#6729,#6730,#6731)) ;
#1818=EDGE_LOOP('',(#6732,#6733,#6734,#6735)) ;
#1819=EDGE_LOOP('',(#6736,#6737,#6738,#6739)) ;
#1820=EDGE_LOOP('',(#6740,#6741,#6742,#6743,#6744,#6745,#6746,#6747,#6748,
#6749,#6750,#6751,#6752,#6753,#6754,#6755,#6756,#6757,#6758,#6759,#6760,
#6761,#6762,#6763,#6764,#6765,#6766,#6767,#6768,#6769,#6770)) ;
#1821=EDGE_LOOP('',(#6771,#6772,#6773,#6774,#6775)) ;
#1822=EDGE_LOOP('',(#6776,#6777,#6778,#6779)) ;
#1823=EDGE_LOOP('',(#6780,#6781,#6782,#6783,#6784,#6785,#6786,#6787,#6788,
#6789,#6790,#6791,#6792,#6793,#6794,#6795,#6796,#6797,#6798,#6799,#6800,
#6801,#6802,#6803,#6804,#6805,#6806,#6807,#6808,#6809)) ;
#1824=EDGE_LOOP('',(#6810,#6811,#6812,#6813,#6814,#6815)) ;
#1825=EDGE_LOOP('',(#6816,#6817,#6818)) ;
#1826=EDGE_LOOP('',(#6819)) ;
#1827=EDGE_LOOP('',(#6820)) ;
#1828=EDGE_LOOP('',(#6821,#6822,#6823,#6824,#6825,#6826)) ;
#1829=EDGE_LOOP('',(#6827)) ;
#1830=EDGE_LOOP('',(#6828,#6829,#6830,#6831)) ;
#1831=EDGE_LOOP('',(#6832,#6833,#6834)) ;
#1832=EDGE_LOOP('',(#6835,#6836,#6837,#6838)) ;
#1833=EDGE_LOOP('',(#6839,#6840,#6841,#6842,#6843,#6844,#6845,#6846,#6847,
#6848,#6849,#6850,#6851,#6852,#6853,#6854,#6855,#6856,#6857,#6858,#6859,
#6860,#6861,#6862,#6863,#6864,#6865,#6866,#6867,#6868,#6869,#6870,#6871,
#6872,#6873,#6874,#6875,#6876,#6877,#6878,#6879,#6880,#6881,#6882,#6883,
#6884,#6885,#6886,#6887,#6888,#6889,#6890,#6891,#6892,#6893,#6894,#6895,
#6896,#6897,#6898,#6899,#6900,#6901,#6902,#6903,#6904,#6905,#6906,#6907,
#6908,#6909,#6910,#6911,#6912,#6913,#6914,#6915,#6916,#6917,#6918,#6919,
#6920,#6921,#6922,#6923,#6924,#6925,#6926,#6927,#6928,#6929,#6930,#6931,
#6932,#6933,#6934,#6935,#6936,#6937,#6938,#6939,#6940,#6941,#6942,#6943,
#6944,#6945,#6946,#6947,#6948,#6949,#6950,#6951,#6952,#6953,#6954,#6955,
#6956,#6957,#6958,#6959,#6960,#6961,#6962,#6963,#6964,#6965,#6966,#6967,
#6968,#6969,#6970,#6971,#6972,#6973,#6974,#6975,#6976,#6977,#6978,#6979,
#6980,#6981,#6982,#6983,#6984,#6985,#6986)) ;
#1834=EDGE_LOOP('',(#6987,#6988,#6989,#6990)) ;
#1835=EDGE_LOOP('',(#6991,#6992,#6993)) ;
#1836=EDGE_LOOP('',(#6994,#6995,#6996,#6997)) ;
#1837=EDGE_LOOP('',(#6998,#6999,#7000,#7001)) ;
#1838=EDGE_LOOP('',(#7002,#7003,#7004)) ;
#1839=EDGE_LOOP('',(#7005,#7006,#7007,#7008)) ;
#1840=EDGE_LOOP('',(#7009,#7010,#7011,#7012)) ;
#1841=EDGE_LOOP('',(#7013,#7014,#7015)) ;
#1842=EDGE_LOOP('',(#7016,#7017,#7018,#7019)) ;
#1843=EDGE_LOOP('',(#7020,#7021,#7022,#7023)) ;
#1844=EDGE_LOOP('',(#7024,#7025,#7026)) ;
#1845=EDGE_LOOP('',(#7027,#7028,#7029,#7030)) ;
#1846=EDGE_LOOP('',(#7031,#7032,#7033,#7034)) ;
#1847=EDGE_LOOP('',(#7035,#7036,#7037)) ;
#1848=EDGE_LOOP('',(#7038,#7039,#7040,#7041)) ;
#1849=EDGE_LOOP('',(#7042,#7043,#7044,#7045)) ;
#1850=EDGE_LOOP('',(#7046,#7047,#7048)) ;
#1851=EDGE_LOOP('',(#7049,#7050,#7051,#7052)) ;
#1852=EDGE_LOOP('',(#7053,#7054,#7055,#7056)) ;
#1853=EDGE_LOOP('',(#7057,#7058,#7059)) ;
#1854=EDGE_LOOP('',(#7060,#7061,#7062,#7063)) ;
#1855=EDGE_LOOP('',(#7064,#7065,#7066,#7067)) ;
#1856=EDGE_LOOP('',(#7068,#7069,#7070,#7071)) ;
#1857=EDGE_LOOP('',(#7072,#7073,#7074,#7075)) ;
#1858=EDGE_LOOP('',(#7076,#7077,#7078,#7079)) ;
#1859=EDGE_LOOP('',(#7080,#7081,#7082)) ;
#1860=EDGE_LOOP('',(#7083,#7084,#7085,#7086)) ;
#1861=EDGE_LOOP('',(#7087,#7088,#7089,#7090)) ;
#1862=EDGE_LOOP('',(#7091,#7092,#7093)) ;
#1863=EDGE_LOOP('',(#7094,#7095,#7096,#7097)) ;
#1864=EDGE_LOOP('',(#7098,#7099,#7100,#7101)) ;
#1865=EDGE_LOOP('',(#7102,#7103,#7104)) ;
#1866=EDGE_LOOP('',(#7105,#7106,#7107,#7108)) ;
#1867=EDGE_LOOP('',(#7109,#7110,#7111,#7112)) ;
#1868=EDGE_LOOP('',(#7113,#7114,#7115)) ;
#1869=EDGE_LOOP('',(#7116,#7117,#7118,#7119)) ;
#1870=EDGE_LOOP('',(#7120,#7121,#7122,#7123)) ;
#1871=EDGE_LOOP('',(#7124,#7125,#7126)) ;
#1872=EDGE_LOOP('',(#7127,#7128,#7129,#7130)) ;
#1873=EDGE_LOOP('',(#7131,#7132,#7133,#7134)) ;
#1874=EDGE_LOOP('',(#7135,#7136,#7137)) ;
#1875=EDGE_LOOP('',(#7138,#7139,#7140,#7141)) ;
#1876=EDGE_LOOP('',(#7142,#7143,#7144,#7145)) ;
#1877=EDGE_LOOP('',(#7146,#7147,#7148)) ;
#1878=EDGE_LOOP('',(#7149,#7150,#7151,#7152)) ;
#1879=EDGE_LOOP('',(#7153,#7154,#7155,#7156)) ;
#1880=EDGE_LOOP('',(#7157,#7158,#7159)) ;
#1881=EDGE_LOOP('',(#7160,#7161,#7162,#7163)) ;
#1882=EDGE_LOOP('',(#7164,#7165,#7166,#7167)) ;
#1883=EDGE_LOOP('',(#7168,#7169,#7170)) ;
#1884=EDGE_LOOP('',(#7171,#7172,#7173,#7174)) ;
#1885=EDGE_LOOP('',(#7175,#7176,#7177,#7178)) ;
#1886=EDGE_LOOP('',(#7179,#7180,#7181)) ;
#1887=EDGE_LOOP('',(#7182,#7183,#7184,#7185)) ;
#1888=EDGE_LOOP('',(#7186,#7187,#7188,#7189)) ;
#1889=EDGE_LOOP('',(#7190,#7191,#7192)) ;
#1890=EDGE_LOOP('',(#7193,#7194,#7195,#7196)) ;
#1891=EDGE_LOOP('',(#7197,#7198,#7199,#7200)) ;
#1892=EDGE_LOOP('',(#7201,#7202,#7203)) ;
#1893=EDGE_LOOP('',(#7204,#7205,#7206,#7207)) ;
#1894=EDGE_LOOP('',(#7208,#7209,#7210,#7211)) ;
#1895=EDGE_LOOP('',(#7212,#7213,#7214)) ;
#1896=EDGE_LOOP('',(#7215,#7216,#7217,#7218)) ;
#1897=EDGE_LOOP('',(#7219,#7220,#7221,#7222)) ;
#1898=EDGE_LOOP('',(#7223,#7224,#7225)) ;
#1899=EDGE_LOOP('',(#7226,#7227,#7228,#7229)) ;
#1900=EDGE_LOOP('',(#7230,#7231,#7232,#7233)) ;
#1901=EDGE_LOOP('',(#7234,#7235,#7236)) ;
#1902=EDGE_LOOP('',(#7237,#7238,#7239,#7240)) ;
#1903=EDGE_LOOP('',(#7241,#7242,#7243,#7244)) ;
#1904=EDGE_LOOP('',(#7245,#7246,#7247)) ;
#1905=EDGE_LOOP('',(#7248,#7249,#7250,#7251)) ;
#1906=EDGE_LOOP('',(#7252,#7253,#7254,#7255)) ;
#1907=EDGE_LOOP('',(#7256,#7257,#7258)) ;
#1908=EDGE_LOOP('',(#7259,#7260,#7261,#7262)) ;
#1909=EDGE_LOOP('',(#7263,#7264,#7265,#7266)) ;
#1910=EDGE_LOOP('',(#7267,#7268,#7269)) ;
#1911=EDGE_LOOP('',(#7270,#7271,#7272,#7273)) ;
#1912=EDGE_LOOP('',(#7274,#7275,#7276,#7277)) ;
#1913=EDGE_LOOP('',(#7278,#7279,#7280)) ;
#1914=EDGE_LOOP('',(#7281,#7282,#7283,#7284)) ;
#1915=EDGE_LOOP('',(#7285,#7286,#7287,#7288)) ;
#1916=EDGE_LOOP('',(#7289,#7290,#7291)) ;
#1917=EDGE_LOOP('',(#7292,#7293,#7294,#7295)) ;
#1918=EDGE_LOOP('',(#7296,#7297,#7298,#7299)) ;
#1919=EDGE_LOOP('',(#7300,#7301,#7302)) ;
#1920=EDGE_LOOP('',(#7303,#7304,#7305,#7306)) ;
#1921=EDGE_LOOP('',(#7307,#7308,#7309,#7310)) ;
#1922=EDGE_LOOP('',(#7311,#7312,#7313)) ;
#1923=EDGE_LOOP('',(#7314,#7315,#7316,#7317)) ;
#1924=EDGE_LOOP('',(#7318,#7319,#7320,#7321)) ;
#1925=EDGE_LOOP('',(#7322,#7323,#7324)) ;
#1926=EDGE_LOOP('',(#7325,#7326,#7327,#7328)) ;
#1927=EDGE_LOOP('',(#7329,#7330,#7331,#7332)) ;
#1928=EDGE_LOOP('',(#7333,#7334,#7335)) ;
#1929=EDGE_LOOP('',(#7336,#7337,#7338,#7339)) ;
#1930=EDGE_LOOP('',(#7340,#7341,#7342,#7343)) ;
#1931=EDGE_LOOP('',(#7344,#7345,#7346)) ;
#1932=EDGE_LOOP('',(#7347,#7348,#7349,#7350)) ;
#1933=EDGE_LOOP('',(#7351,#7352,#7353,#7354)) ;
#1934=EDGE_LOOP('',(#7355,#7356,#7357)) ;
#1935=EDGE_LOOP('',(#7358,#7359,#7360,#7361)) ;
#1936=EDGE_LOOP('',(#7362,#7363,#7364,#7365)) ;
#1937=EDGE_LOOP('',(#7366,#7367,#7368)) ;
#1938=EDGE_LOOP('',(#7369,#7370,#7371,#7372)) ;
#1939=EDGE_LOOP('',(#7373,#7374,#7375,#7376)) ;
#1940=EDGE_LOOP('',(#7377,#7378,#7379,#7380,#7381,#7382,#7383,#7384,#7385,
#7386,#7387,#7388,#7389,#7390,#7391,#7392,#7393,#7394,#7395,#7396,#7397,
#7398,#7399,#7400,#7401,#7402,#7403,#7404,#7405,#7406,#7407,#7408,#7409,
#7410,#7411,#7412,#7413,#7414,#7415,#7416,#7417,#7418,#7419,#7420,#7421,
#7422,#7423,#7424,#7425,#7426,#7427,#7428,#7429,#7430,#7431,#7432,#7433,
#7434,#7435,#7436,#7437,#7438,#7439,#7440,#7441,#7442,#7443,#7444,#7445,
#7446,#7447,#7448,#7449,#7450,#7451,#7452,#7453,#7454,#7455,#7456,#7457,
#7458,#7459,#7460,#7461,#7462,#7463,#7464,#7465,#7466,#7467,#7468,#7469,
#7470,#7471,#7472,#7473,#7474,#7475,#7476,#7477,#7478,#7479,#7480,#7481,
#7482,#7483,#7484,#7485,#7486,#7487)) ;
#1941=EDGE_LOOP('',(#7488)) ;
#1942=EDGE_LOOP('',(#7489)) ;
#1943=EDGE_LOOP('',(#7490,#7491,#7492,#7493,#7494,#7495,#7496,#7497,#7498,
#7499,#7500,#7501,#7502,#7503,#7504,#7505,#7506,#7507,#7508,#7509,#7510)) ;
#1944=EDGE_LOOP('',(#7511,#7512,#7513,#7514)) ;
#1945=EDGE_LOOP('',(#7515,#7516,#7517,#7518)) ;
#1946=EDGE_LOOP('',(#7519,#7520,#7521,#7522)) ;
#1947=EDGE_LOOP('',(#7523,#7524,#7525,#7526)) ;
#1948=EDGE_LOOP('',(#7527,#7528,#7529,#7530)) ;
#1949=EDGE_LOOP('',(#7531,#7532,#7533,#7534)) ;
#1950=EDGE_LOOP('',(#7535,#7536,#7537,#7538,#7539,#7540,#7541,#7542)) ;
#1951=EDGE_LOOP('',(#7543,#7544,#7545,#7546,#7547,#7548,#7549,#7550)) ;
#1952=EDGE_LOOP('',(#7551,#7552,#7553,#7554,#7555,#7556,#7557,#7558)) ;
#1953=EDGE_LOOP('',(#7559,#7560)) ;
#1954=EDGE_LOOP('',(#7561,#7562)) ;
#1955=EDGE_LOOP('',(#7563,#7564)) ;
#1956=EDGE_LOOP('',(#7565,#7566)) ;
#1957=EDGE_LOOP('',(#7567,#7568)) ;
#1958=EDGE_LOOP('',(#7569,#7570)) ;
#1959=EDGE_LOOP('',(#7571,#7572)) ;
#1960=EDGE_LOOP('',(#7573,#7574)) ;
#1961=EDGE_LOOP('',(#7575,#7576)) ;
#1962=EDGE_LOOP('',(#7577,#7578)) ;
#1963=EDGE_LOOP('',(#7579,#7580)) ;
#1964=EDGE_LOOP('',(#7581,#7582)) ;
#1965=EDGE_LOOP('',(#7583,#7584,#7585,#7586,#7587,#7588,#7589,#7590)) ;
#1966=EDGE_LOOP('',(#7591,#7592,#7593,#7594,#7595,#7596,#7597,#7598)) ;
#1967=EDGE_LOOP('',(#7599,#7600,#7601,#7602,#7603,#7604,#7605,#7606)) ;
#1968=EDGE_LOOP('',(#7607,#7608,#7609,#7610,#7611,#7612,#7613,#7614)) ;
#2287=LINE('',#13722,#2849) ;
#2288=LINE('',#13746,#2850) ;
#2289=LINE('',#13794,#2851) ;
#2290=LINE('',#13842,#2852) ;
#2291=LINE('',#13896,#2853) ;
#2292=LINE('',#13944,#2854) ;
#2293=LINE('',#13992,#2855) ;
#2294=LINE('',#14046,#2856) ;
#2295=LINE('',#14094,#2857) ;
#2296=LINE('',#14142,#2858) ;
#2297=LINE('',#14190,#2859) ;
#2298=LINE('',#14244,#2860) ;
#2299=LINE('',#14292,#2861) ;
#2300=LINE('',#14340,#2862) ;
#2301=LINE('',#14393,#2863) ;
#2302=LINE('',#14414,#2864) ;
#2303=LINE('',#14439,#2865) ;
#2304=LINE('',#14463,#2866) ;
#2305=LINE('',#14488,#2867) ;
#2306=LINE('',#14513,#2868) ;
#2307=LINE('',#14537,#2869) ;
#2308=LINE('',#14561,#2870) ;
#2309=LINE('',#14586,#2871) ;
#2310=LINE('',#14611,#2872) ;
#2311=LINE('',#14635,#2873) ;
#2312=LINE('',#14660,#2874) ;
#2313=LINE('',#14685,#2875) ;
#2314=LINE('',#15813,#2876) ;
#2315=LINE('',#15823,#2877) ;
#2316=LINE('',#15825,#2878) ;
#2317=LINE('',#15826,#2879) ;
#2318=LINE('',#15830,#2880) ;
#2319=LINE('',#15836,#2881) ;
#2320=LINE('',#15841,#2882) ;
#2321=LINE('',#15845,#2883) ;
#2322=LINE('',#15849,#2884) ;
#2323=LINE('',#15853,#2885) ;
#2324=LINE('',#15857,#2886) ;
#2325=LINE('',#15861,#2887) ;
#2326=LINE('',#15865,#2888) ;
#2327=LINE('',#15869,#2889) ;
#2328=LINE('',#15873,#2890) ;
#2329=LINE('',#15877,#2891) ;
#2330=LINE('',#15881,#2892) ;
#2331=LINE('',#15885,#2893) ;
#2332=LINE('',#15889,#2894) ;
#2333=LINE('',#15893,#2895) ;
#2334=LINE('',#15897,#2896) ;
#2335=LINE('',#15901,#2897) ;
#2336=LINE('',#15905,#2898) ;
#2337=LINE('',#15909,#2899) ;
#2338=LINE('',#15913,#2900) ;
#2339=LINE('',#15917,#2901) ;
#2340=LINE('',#15921,#2902) ;
#2341=LINE('',#15925,#2903) ;
#2342=LINE('',#15929,#2904) ;
#2343=LINE('',#15933,#2905) ;
#2344=LINE('',#15937,#2906) ;
#2345=LINE('',#15941,#2907) ;
#2346=LINE('',#15945,#2908) ;
#2347=LINE('',#15949,#2909) ;
#2348=LINE('',#15953,#2910) ;
#2349=LINE('',#15957,#2911) ;
#2350=LINE('',#15961,#2912) ;
#2351=LINE('',#15965,#2913) ;
#2352=LINE('',#15969,#2914) ;
#2353=LINE('',#15973,#2915) ;
#2354=LINE('',#15977,#2916) ;
#2355=LINE('',#15981,#2917) ;
#2356=LINE('',#15985,#2918) ;
#2357=LINE('',#15989,#2919) ;
#2358=LINE('',#15993,#2920) ;
#2359=LINE('',#15997,#2921) ;
#2360=LINE('',#16001,#2922) ;
#2361=LINE('',#16005,#2923) ;
#2362=LINE('',#16009,#2924) ;
#2363=LINE('',#16013,#2925) ;
#2364=LINE('',#16017,#2926) ;
#2365=LINE('',#16021,#2927) ;
#2366=LINE('',#16025,#2928) ;
#2367=LINE('',#16029,#2929) ;
#2368=LINE('',#16033,#2930) ;
#2369=LINE('',#16037,#2931) ;
#2370=LINE('',#16041,#2932) ;
#2371=LINE('',#16045,#2933) ;
#2372=LINE('',#16049,#2934) ;
#2373=LINE('',#16053,#2935) ;
#2374=LINE('',#16057,#2936) ;
#2375=LINE('',#16061,#2937) ;
#2376=LINE('',#16066,#2938) ;
#2377=LINE('',#16070,#2939) ;
#2378=LINE('',#16074,#2940) ;
#2379=LINE('',#16078,#2941) ;
#2380=LINE('',#16082,#2942) ;
#2381=LINE('',#16086,#2943) ;
#2382=LINE('',#16090,#2944) ;
#2383=LINE('',#16094,#2945) ;
#2384=LINE('',#16098,#2946) ;
#2385=LINE('',#16102,#2947) ;
#2386=LINE('',#16106,#2948) ;
#2387=LINE('',#16110,#2949) ;
#2388=LINE('',#16114,#2950) ;
#2389=LINE('',#16118,#2951) ;
#2390=LINE('',#16122,#2952) ;
#2391=LINE('',#16130,#2953) ;
#2392=LINE('',#16131,#2954) ;
#2393=LINE('',#16133,#2955) ;
#2394=LINE('',#16144,#2956) ;
#2395=LINE('',#16145,#2957) ;
#2396=LINE('',#16147,#2958) ;
#2397=LINE('',#16158,#2959) ;
#2398=LINE('',#16159,#2960) ;
#2399=LINE('',#16161,#2961) ;
#2400=LINE('',#16172,#2962) ;
#2401=LINE('',#16173,#2963) ;
#2402=LINE('',#16175,#2964) ;
#2403=LINE('',#16186,#2965) ;
#2404=LINE('',#16187,#2966) ;
#2405=LINE('',#16189,#2967) ;
#2406=LINE('',#16200,#2968) ;
#2407=LINE('',#16201,#2969) ;
#2408=LINE('',#16203,#2970) ;
#2409=LINE('',#16214,#2971) ;
#2410=LINE('',#16215,#2972) ;
#2411=LINE('',#16217,#2973) ;
#2412=LINE('',#16228,#2974) ;
#2413=LINE('',#16229,#2975) ;
#2414=LINE('',#16231,#2976) ;
#2415=LINE('',#16242,#2977) ;
#2416=LINE('',#16243,#2978) ;
#2417=LINE('',#16245,#2979) ;
#2418=LINE('',#16256,#2980) ;
#2419=LINE('',#16257,#2981) ;
#2420=LINE('',#16259,#2982) ;
#2421=LINE('',#16270,#2983) ;
#2422=LINE('',#16271,#2984) ;
#2423=LINE('',#16273,#2985) ;
#2424=LINE('',#16284,#2986) ;
#2425=LINE('',#16285,#2987) ;
#2426=LINE('',#16287,#2988) ;
#2427=LINE('',#16298,#2989) ;
#2428=LINE('',#16299,#2990) ;
#2429=LINE('',#16301,#2991) ;
#2430=LINE('',#16312,#2992) ;
#2431=LINE('',#16313,#2993) ;
#2432=LINE('',#16315,#2994) ;
#2433=LINE('',#16326,#2995) ;
#2434=LINE('',#16327,#2996) ;
#2435=LINE('',#16329,#2997) ;
#2436=LINE('',#16340,#2998) ;
#2437=LINE('',#16341,#2999) ;
#2438=LINE('',#16343,#3000) ;
#2439=LINE('',#16354,#3001) ;
#2440=LINE('',#16355,#3002) ;
#2441=LINE('',#16357,#3003) ;
#2442=LINE('',#16368,#3004) ;
#2443=LINE('',#16369,#3005) ;
#2444=LINE('',#16371,#3006) ;
#2445=LINE('',#16382,#3007) ;
#2446=LINE('',#16383,#3008) ;
#2447=LINE('',#16385,#3009) ;
#2448=LINE('',#16396,#3010) ;
#2449=LINE('',#16397,#3011) ;
#2450=LINE('',#16399,#3012) ;
#2451=LINE('',#16410,#3013) ;
#2452=LINE('',#16411,#3014) ;
#2453=LINE('',#16413,#3015) ;
#2454=LINE('',#16424,#3016) ;
#2455=LINE('',#16425,#3017) ;
#2456=LINE('',#16427,#3018) ;
#2457=LINE('',#16438,#3019) ;
#2458=LINE('',#16439,#3020) ;
#2459=LINE('',#16441,#3021) ;
#2460=LINE('',#16452,#3022) ;
#2461=LINE('',#16453,#3023) ;
#2462=LINE('',#16455,#3024) ;
#2463=LINE('',#16466,#3025) ;
#2464=LINE('',#16467,#3026) ;
#2465=LINE('',#16469,#3027) ;
#2466=LINE('',#16480,#3028) ;
#2467=LINE('',#16481,#3029) ;
#2468=LINE('',#16483,#3030) ;
#2469=LINE('',#16494,#3031) ;
#2470=LINE('',#16495,#3032) ;
#2471=LINE('',#16497,#3033) ;
#2472=LINE('',#16508,#3034) ;
#2473=LINE('',#16509,#3035) ;
#2474=LINE('',#16511,#3036) ;
#2475=LINE('',#16522,#3037) ;
#2476=LINE('',#16523,#3038) ;
#2477=LINE('',#16525,#3039) ;
#2478=LINE('',#16536,#3040) ;
#2479=LINE('',#16537,#3041) ;
#2480=LINE('',#16539,#3042) ;
#2481=LINE('',#16550,#3043) ;
#2482=LINE('',#16551,#3044) ;
#2483=LINE('',#16553,#3045) ;
#2484=LINE('',#16564,#3046) ;
#2485=LINE('',#16565,#3047) ;
#2486=LINE('',#16567,#3048) ;
#2487=LINE('',#16578,#3049) ;
#2488=LINE('',#16579,#3050) ;
#2489=LINE('',#16581,#3051) ;
#2490=LINE('',#16592,#3052) ;
#2491=LINE('',#16593,#3053) ;
#2492=LINE('',#16595,#3054) ;
#2493=LINE('',#16606,#3055) ;
#2494=LINE('',#16607,#3056) ;
#2495=LINE('',#16609,#3057) ;
#2496=LINE('',#16619,#3058) ;
#2497=LINE('',#16675,#3059) ;
#2498=LINE('',#16687,#3060) ;
#2499=LINE('',#16689,#3061) ;
#2500=LINE('',#16693,#3062) ;
#2501=LINE('',#16696,#3063) ;
#2502=LINE('',#16699,#3064) ;
#2503=LINE('',#16701,#3065) ;
#2504=LINE('',#16705,#3066) ;
#2505=LINE('',#16708,#3067) ;
#2506=LINE('',#16711,#3068) ;
#2507=LINE('',#16713,#3069) ;
#2508=LINE('',#16717,#3070) ;
#2509=LINE('',#16720,#3071) ;
#2510=LINE('',#16722,#3072) ;
#2511=LINE('',#16724,#3073) ;
#2512=LINE('',#16726,#3074) ;
#2513=LINE('',#16727,#3075) ;
#2514=LINE('',#16729,#3076) ;
#2515=LINE('',#16731,#3077) ;
#2516=LINE('',#16732,#3078) ;
#2517=LINE('',#16734,#3079) ;
#2518=LINE('',#16736,#3080) ;
#2519=LINE('',#16737,#3081) ;
#2520=LINE('',#16741,#3082) ;
#2521=LINE('',#16744,#3083) ;
#2522=LINE('',#16746,#3084) ;
#2523=LINE('',#16750,#3085) ;
#2524=LINE('',#16753,#3086) ;
#2525=LINE('',#16762,#3087) ;
#2526=LINE('',#16766,#3088) ;
#2527=LINE('',#16768,#3089) ;
#2528=LINE('',#16769,#3090) ;
#2849=VECTOR('',#9933,2.) ;
#2850=VECTOR('',#9938,2.) ;
#2851=VECTOR('',#9941,2.) ;
#2852=VECTOR('',#9944,2.) ;
#2853=VECTOR('',#9947,2.) ;
#2854=VECTOR('',#9950,2.) ;
#2855=VECTOR('',#9953,2.) ;
#2856=VECTOR('',#9956,2.) ;
#2857=VECTOR('',#9959,2.) ;
#2858=VECTOR('',#9962,2.) ;
#2859=VECTOR('',#9965,2.) ;
#2860=VECTOR('',#9968,2.) ;
#2861=VECTOR('',#9971,2.) ;
#2862=VECTOR('',#9974,2.) ;
#2863=VECTOR('',#9979,1.5555) ;
#2864=VECTOR('',#9984,1.5555) ;
#2865=VECTOR('',#9987,1.5555) ;
#2866=VECTOR('',#9990,1.5555) ;
#2867=VECTOR('',#9993,1.5555) ;
#2868=VECTOR('',#9996,1.5555) ;
#2869=VECTOR('',#9999,1.5555) ;
#2870=VECTOR('',#10002,1.5555) ;
#2871=VECTOR('',#10005,1.5555) ;
#2872=VECTOR('',#10008,1.5555) ;
#2873=VECTOR('',#10011,1.5555) ;
#2874=VECTOR('',#10014,1.5555) ;
#2875=VECTOR('',#10017,1.5555) ;
#2876=VECTOR('',#10048,1.704) ;
#2877=VECTOR('',#10055,10.) ;
#2878=VECTOR('',#10056,10.) ;
#2879=VECTOR('',#10057,10.) ;
#2880=VECTOR('',#10062,10.) ;
#2881=VECTOR('',#10065,10.) ;
#2882=VECTOR('',#10070,10.) ;
#2883=VECTOR('',#10073,10.) ;
#2884=VECTOR('',#10076,10.) ;
#2885=VECTOR('',#10079,10.) ;
#2886=VECTOR('',#10082,10.) ;
#2887=VECTOR('',#10085,10.) ;
#2888=VECTOR('',#10088,10.) ;
#2889=VECTOR('',#10091,10.) ;
#2890=VECTOR('',#10094,10.) ;
#2891=VECTOR('',#10097,10.) ;
#2892=VECTOR('',#10100,10.) ;
#2893=VECTOR('',#10103,10.) ;
#2894=VECTOR('',#10106,10.) ;
#2895=VECTOR('',#10109,10.) ;
#2896=VECTOR('',#10112,10.) ;
#2897=VECTOR('',#10115,10.) ;
#2898=VECTOR('',#10118,10.) ;
#2899=VECTOR('',#10121,10.) ;
#2900=VECTOR('',#10124,10.) ;
#2901=VECTOR('',#10127,10.) ;
#2902=VECTOR('',#10130,10.) ;
#2903=VECTOR('',#10133,10.) ;
#2904=VECTOR('',#10136,10.) ;
#2905=VECTOR('',#10139,10.) ;
#2906=VECTOR('',#10142,10.) ;
#2907=VECTOR('',#10145,10.) ;
#2908=VECTOR('',#10148,10.) ;
#2909=VECTOR('',#10151,10.) ;
#2910=VECTOR('',#10154,10.) ;
#2911=VECTOR('',#10157,10.) ;
#2912=VECTOR('',#10160,10.) ;
#2913=VECTOR('',#10163,10.) ;
#2914=VECTOR('',#10166,10.) ;
#2915=VECTOR('',#10169,10.) ;
#2916=VECTOR('',#10172,10.) ;
#2917=VECTOR('',#10175,10.) ;
#2918=VECTOR('',#10178,10.) ;
#2919=VECTOR('',#10181,10.) ;
#2920=VECTOR('',#10184,10.) ;
#2921=VECTOR('',#10187,10.) ;
#2922=VECTOR('',#10190,10.) ;
#2923=VECTOR('',#10193,10.) ;
#2924=VECTOR('',#10196,10.) ;
#2925=VECTOR('',#10199,10.) ;
#2926=VECTOR('',#10202,10.) ;
#2927=VECTOR('',#10205,10.) ;
#2928=VECTOR('',#10208,10.) ;
#2929=VECTOR('',#10211,10.) ;
#2930=VECTOR('',#10214,10.) ;
#2931=VECTOR('',#10217,10.) ;
#2932=VECTOR('',#10220,10.) ;
#2933=VECTOR('',#10223,10.) ;
#2934=VECTOR('',#10226,10.) ;
#2935=VECTOR('',#10229,10.) ;
#2936=VECTOR('',#10232,10.) ;
#2937=VECTOR('',#10235,3.5) ;
#2938=VECTOR('',#10240,10.) ;
#2939=VECTOR('',#10243,10.) ;
#2940=VECTOR('',#10246,10.) ;
#2941=VECTOR('',#10249,10.) ;
#2942=VECTOR('',#10252,10.) ;
#2943=VECTOR('',#10255,10.) ;
#2944=VECTOR('',#10258,10.) ;
#2945=VECTOR('',#10261,10.) ;
#2946=VECTOR('',#10264,10.) ;
#2947=VECTOR('',#10267,10.) ;
#2948=VECTOR('',#10270,10.) ;
#2949=VECTOR('',#10273,10.) ;
#2950=VECTOR('',#10276,10.) ;
#2951=VECTOR('',#10279,10.) ;
#2952=VECTOR('',#10282,10.) ;
#2953=VECTOR('',#10287,10.) ;
#2954=VECTOR('',#10288,10.) ;
#2955=VECTOR('',#10291,10.) ;
#2956=VECTOR('',#10296,10.) ;
#2957=VECTOR('',#10297,10.) ;
#2958=VECTOR('',#10300,10.) ;
#2959=VECTOR('',#10305,10.) ;
#2960=VECTOR('',#10306,10.) ;
#2961=VECTOR('',#10309,10.) ;
#2962=VECTOR('',#10314,10.) ;
#2963=VECTOR('',#10315,10.) ;
#2964=VECTOR('',#10318,10.) ;
#2965=VECTOR('',#10323,10.) ;
#2966=VECTOR('',#10324,10.) ;
#2967=VECTOR('',#10327,10.) ;
#2968=VECTOR('',#10332,10.) ;
#2969=VECTOR('',#10333,10.) ;
#2970=VECTOR('',#10336,10.) ;
#2971=VECTOR('',#10341,10.) ;
#2972=VECTOR('',#10342,10.) ;
#2973=VECTOR('',#10345,10.) ;
#2974=VECTOR('',#10350,10.) ;
#2975=VECTOR('',#10351,10.) ;
#2976=VECTOR('',#10354,10.) ;
#2977=VECTOR('',#10359,10.) ;
#2978=VECTOR('',#10360,10.) ;
#2979=VECTOR('',#10363,10.) ;
#2980=VECTOR('',#10368,10.) ;
#2981=VECTOR('',#10369,10.) ;
#2982=VECTOR('',#10372,10.) ;
#2983=VECTOR('',#10377,10.) ;
#2984=VECTOR('',#10378,10.) ;
#2985=VECTOR('',#10381,10.) ;
#2986=VECTOR('',#10386,10.) ;
#2987=VECTOR('',#10387,10.) ;
#2988=VECTOR('',#10390,10.) ;
#2989=VECTOR('',#10395,10.) ;
#2990=VECTOR('',#10396,10.) ;
#2991=VECTOR('',#10399,10.) ;
#2992=VECTOR('',#10404,10.) ;
#2993=VECTOR('',#10405,10.) ;
#2994=VECTOR('',#10408,10.) ;
#2995=VECTOR('',#10413,10.) ;
#2996=VECTOR('',#10414,10.) ;
#2997=VECTOR('',#10417,10.) ;
#2998=VECTOR('',#10422,10.) ;
#2999=VECTOR('',#10423,10.) ;
#3000=VECTOR('',#10426,10.) ;
#3001=VECTOR('',#10431,10.) ;
#3002=VECTOR('',#10432,10.) ;
#3003=VECTOR('',#10435,10.) ;
#3004=VECTOR('',#10440,10.) ;
#3005=VECTOR('',#10441,10.) ;
#3006=VECTOR('',#10444,10.) ;
#3007=VECTOR('',#10449,10.) ;
#3008=VECTOR('',#10450,10.) ;
#3009=VECTOR('',#10453,10.) ;
#3010=VECTOR('',#10458,10.) ;
#3011=VECTOR('',#10459,10.) ;
#3012=VECTOR('',#10462,10.) ;
#3013=VECTOR('',#10467,10.) ;
#3014=VECTOR('',#10468,10.) ;
#3015=VECTOR('',#10471,10.) ;
#3016=VECTOR('',#10476,10.) ;
#3017=VECTOR('',#10477,10.) ;
#3018=VECTOR('',#10480,10.) ;
#3019=VECTOR('',#10485,10.) ;
#3020=VECTOR('',#10486,10.) ;
#3021=VECTOR('',#10489,10.) ;
#3022=VECTOR('',#10494,10.) ;
#3023=VECTOR('',#10495,10.) ;
#3024=VECTOR('',#10498,10.) ;
#3025=VECTOR('',#10503,10.) ;
#3026=VECTOR('',#10504,10.) ;
#3027=VECTOR('',#10507,10.) ;
#3028=VECTOR('',#10512,10.) ;
#3029=VECTOR('',#10513,10.) ;
#3030=VECTOR('',#10516,10.) ;
#3031=VECTOR('',#10521,10.) ;
#3032=VECTOR('',#10522,10.) ;
#3033=VECTOR('',#10525,10.) ;
#3034=VECTOR('',#10530,10.) ;
#3035=VECTOR('',#10531,10.) ;
#3036=VECTOR('',#10534,10.) ;
#3037=VECTOR('',#10539,10.) ;
#3038=VECTOR('',#10540,10.) ;
#3039=VECTOR('',#10543,10.) ;
#3040=VECTOR('',#10548,10.) ;
#3041=VECTOR('',#10549,10.) ;
#3042=VECTOR('',#10552,10.) ;
#3043=VECTOR('',#10557,10.) ;
#3044=VECTOR('',#10558,10.) ;
#3045=VECTOR('',#10561,10.) ;
#3046=VECTOR('',#10566,10.) ;
#3047=VECTOR('',#10567,10.) ;
#3048=VECTOR('',#10570,10.) ;
#3049=VECTOR('',#10575,10.) ;
#3050=VECTOR('',#10576,10.) ;
#3051=VECTOR('',#10579,10.) ;
#3052=VECTOR('',#10584,10.) ;
#3053=VECTOR('',#10585,10.) ;
#3054=VECTOR('',#10588,10.) ;
#3055=VECTOR('',#10593,10.) ;
#3056=VECTOR('',#10594,10.) ;
#3057=VECTOR('',#10597,10.) ;
#3058=VECTOR('',#10608,3.3) ;
#3059=VECTOR('',#10625,1.83205080756888) ;
#3060=VECTOR('',#10630,10.) ;
#3061=VECTOR('',#10631,10.) ;
#3062=VECTOR('',#10636,10.) ;
#3063=VECTOR('',#10639,10.) ;
#3064=VECTOR('',#10642,10.) ;
#3065=VECTOR('',#10643,10.) ;
#3066=VECTOR('',#10648,10.) ;
#3067=VECTOR('',#10651,10.) ;
#3068=VECTOR('',#10654,10.) ;
#3069=VECTOR('',#10655,10.) ;
#3070=VECTOR('',#10660,10.) ;
#3071=VECTOR('',#10663,10.) ;
#3072=VECTOR('',#10666,10.) ;
#3073=VECTOR('',#10667,10.) ;
#3074=VECTOR('',#10668,10.) ;
#3075=VECTOR('',#10669,10.) ;
#3076=VECTOR('',#10672,10.) ;
#3077=VECTOR('',#10673,10.) ;
#3078=VECTOR('',#10674,10.) ;
#3079=VECTOR('',#10677,10.) ;
#3080=VECTOR('',#10678,10.) ;
#3081=VECTOR('',#10679,10.) ;
#3082=VECTOR('',#10686,10.) ;
#3083=VECTOR('',#10691,10.) ;
#3084=VECTOR('',#10694,10.) ;
#3085=VECTOR('',#10697,10.) ;
#3086=VECTOR('',#10702,10.) ;
#3087=VECTOR('',#10719,10.) ;
#3088=VECTOR('',#10724,0.866025403784438) ;
#3089=VECTOR('',#10727,10.) ;
#3090=VECTOR('',#10728,10.) ;
#3274=CIRCLE('',#8598,1.954) ;
#3275=CIRCLE('',#8612,1.954) ;
#3276=CIRCLE('',#8614,1.5555) ;
#3277=CIRCLE('',#8628,1.954) ;
#3278=CIRCLE('',#8630,1.954) ;
#3279=CIRCLE('',#8631,1.5555) ;
#3280=CIRCLE('',#8632,1.954) ;
#3281=CIRCLE('',#8635,0.2) ;
#3282=CIRCLE('',#8636,2.154) ;
#3283=CIRCLE('',#8638,1.954) ;
#3284=CIRCLE('',#8640,3.3) ;
#3285=CIRCLE('',#8642,1.454) ;
#3286=CIRCLE('',#8646,3.5) ;
#3287=CIRCLE('',#8649,3.5) ;
#3288=CIRCLE('',#8650,3.5) ;
#3289=CIRCLE('',#8651,3.5) ;
#3290=CIRCLE('',#8652,3.5) ;
#3291=CIRCLE('',#8653,3.5) ;
#3292=CIRCLE('',#8654,3.5) ;
#3293=CIRCLE('',#8655,3.5) ;
#3294=CIRCLE('',#8656,3.5) ;
#3295=CIRCLE('',#8657,3.5) ;
#3296=CIRCLE('',#8658,3.5) ;
#3297=CIRCLE('',#8659,3.5) ;
#3298=CIRCLE('',#8660,3.5) ;
#3299=CIRCLE('',#8661,3.5) ;
#3300=CIRCLE('',#8662,3.5) ;
#3301=CIRCLE('',#8663,3.5) ;
#3302=CIRCLE('',#8664,3.5) ;
#3303=CIRCLE('',#8665,3.5) ;
#3304=CIRCLE('',#8666,3.5) ;
#3305=CIRCLE('',#8667,3.5) ;
#3306=CIRCLE('',#8668,3.5) ;
#3307=CIRCLE('',#8669,3.5) ;
#3308=CIRCLE('',#8670,3.5) ;
#3309=CIRCLE('',#8671,3.5) ;
#3310=CIRCLE('',#8672,3.5) ;
#3311=CIRCLE('',#8673,3.5) ;
#3312=CIRCLE('',#8674,3.5) ;
#3313=CIRCLE('',#8675,3.5) ;
#3314=CIRCLE('',#8676,3.5) ;
#3315=CIRCLE('',#8677,3.5) ;
#3316=CIRCLE('',#8678,3.5) ;
#3317=CIRCLE('',#8679,3.5) ;
#3318=CIRCLE('',#8680,3.5) ;
#3319=CIRCLE('',#8681,3.5) ;
#3320=CIRCLE('',#8682,3.5) ;
#3321=CIRCLE('',#8683,3.5) ;
#3322=CIRCLE('',#8684,3.5) ;
#3323=CIRCLE('',#8685,3.5) ;
#3324=CIRCLE('',#8686,3.5) ;
#3325=CIRCLE('',#8687,3.5) ;
#3326=CIRCLE('',#8688,3.5) ;
#3327=CIRCLE('',#8689,3.5) ;
#3328=CIRCLE('',#8690,3.5) ;
#3329=CIRCLE('',#8691,3.5) ;
#3330=CIRCLE('',#8692,3.5) ;
#3331=CIRCLE('',#8693,3.5) ;
#3332=CIRCLE('',#8694,3.5) ;
#3333=CIRCLE('',#8695,3.5) ;
#3334=CIRCLE('',#8696,3.5) ;
#3335=CIRCLE('',#8697,3.5) ;
#3336=CIRCLE('',#8698,3.5) ;
#3337=CIRCLE('',#8699,3.5) ;
#3338=CIRCLE('',#8700,3.5) ;
#3339=CIRCLE('',#8701,3.5) ;
#3340=CIRCLE('',#8702,3.5) ;
#3341=CIRCLE('',#8703,3.5) ;
#3342=CIRCLE('',#8704,3.5) ;
#3343=CIRCLE('',#8705,3.5) ;
#3344=CIRCLE('',#8706,3.5) ;
#3345=CIRCLE('',#8707,3.5) ;
#3346=CIRCLE('',#8708,3.5) ;
#3347=CIRCLE('',#8709,3.5) ;
#3348=CIRCLE('',#8710,3.5) ;
#3349=CIRCLE('',#8711,3.5) ;
#3350=CIRCLE('',#8712,3.5) ;
#3351=CIRCLE('',#8713,3.5) ;
#3352=CIRCLE('',#8714,3.5) ;
#3353=CIRCLE('',#8715,3.5) ;
#3354=CIRCLE('',#8716,3.5) ;
#3355=CIRCLE('',#8717,3.5) ;
#3356=CIRCLE('',#8718,3.5) ;
#3357=CIRCLE('',#8719,3.5) ;
#3358=CIRCLE('',#8720,3.5) ;
#3359=CIRCLE('',#8721,3.5) ;
#3360=CIRCLE('',#8828,0.2) ;
#3361=CIRCLE('',#8830,3.1) ;
#3362=CIRCLE('',#8832,1.98205080756888) ;
#3363=CIRCLE('',#8834,1.68205080756887) ;
#3364=CIRCLE('',#8835,1.68205080756887) ;
#3365=CIRCLE('',#8836,1.68205080756887) ;
#3366=CIRCLE('',#8837,1.68205080756887) ;
#3367=CIRCLE('',#8838,1.68205080756887) ;
#3368=CIRCLE('',#8839,1.68205080756887) ;
#3369=CIRCLE('',#8841,1.68205080756887) ;
#3370=CIRCLE('',#8843,1.68205080756887) ;
#3371=CIRCLE('',#8845,1.68205080756887) ;
#3372=CIRCLE('',#8847,1.68205080756887) ;
#3373=CIRCLE('',#8849,1.68205080756887) ;
#3374=CIRCLE('',#8851,1.68205080756887) ;
#3375=CIRCLE('',#8862,1.73205080756887) ;
#3376=CIRCLE('',#8864,1.73205080756887) ;
#3377=CIRCLE('',#8866,1.73205080756887) ;
#3378=CIRCLE('',#8868,1.73205080756887) ;
#3379=CIRCLE('',#8870,1.73205080756887) ;
#3380=CIRCLE('',#8872,1.73205080756887) ;
#3821=VERTEX_POINT('',#13720) ;
#3822=VERTEX_POINT('',#13721) ;
#3823=VERTEX_POINT('',#13723) ;
#3824=VERTEX_POINT('',#13734) ;
#3825=VERTEX_POINT('',#13744) ;
#3826=VERTEX_POINT('',#13745) ;
#3827=VERTEX_POINT('',#13792) ;
#3828=VERTEX_POINT('',#13793) ;
#3829=VERTEX_POINT('',#13840) ;
#3830=VERTEX_POINT('',#13841) ;
#3831=VERTEX_POINT('',#13894) ;
#3832=VERTEX_POINT('',#13895) ;
#3833=VERTEX_POINT('',#13942) ;
#3834=VERTEX_POINT('',#13943) ;
#3835=VERTEX_POINT('',#13990) ;
#3836=VERTEX_POINT('',#13991) ;
#3837=VERTEX_POINT('',#14044) ;
#3838=VERTEX_POINT('',#14045) ;
#3839=VERTEX_POINT('',#14092) ;
#3840=VERTEX_POINT('',#14093) ;
#3841=VERTEX_POINT('',#14140) ;
#3842=VERTEX_POINT('',#14141) ;
#3843=VERTEX_POINT('',#14188) ;
#3844=VERTEX_POINT('',#14189) ;
#3845=VERTEX_POINT('',#14242) ;
#3846=VERTEX_POINT('',#14243) ;
#3847=VERTEX_POINT('',#14290) ;
#3848=VERTEX_POINT('',#14291) ;
#3849=VERTEX_POINT('',#14338) ;
#3850=VERTEX_POINT('',#14339) ;
#3851=VERTEX_POINT('',#14341) ;
#3852=VERTEX_POINT('',#14391) ;
#3853=VERTEX_POINT('',#14392) ;
#3854=VERTEX_POINT('',#14394) ;
#3855=VERTEX_POINT('',#14403) ;
#3856=VERTEX_POINT('',#14412) ;
#3857=VERTEX_POINT('',#14413) ;
#3858=VERTEX_POINT('',#14437) ;
#3859=VERTEX_POINT('',#14438) ;
#3860=VERTEX_POINT('',#14461) ;
#3861=VERTEX_POINT('',#14462) ;
#3862=VERTEX_POINT('',#14486) ;
#3863=VERTEX_POINT('',#14487) ;
#3864=VERTEX_POINT('',#14511) ;
#3865=VERTEX_POINT('',#14512) ;
#3866=VERTEX_POINT('',#14535) ;
#3867=VERTEX_POINT('',#14536) ;
#3868=VERTEX_POINT('',#14559) ;
#3869=VERTEX_POINT('',#14560) ;
#3870=VERTEX_POINT('',#14584) ;
#3871=VERTEX_POINT('',#14585) ;
#3872=VERTEX_POINT('',#14609) ;
#3873=VERTEX_POINT('',#14610) ;
#3874=VERTEX_POINT('',#14633) ;
#3875=VERTEX_POINT('',#14634) ;
#3876=VERTEX_POINT('',#14658) ;
#3877=VERTEX_POINT('',#14659) ;
#3878=VERTEX_POINT('',#14683) ;
#3879=VERTEX_POINT('',#14684) ;
#3880=VERTEX_POINT('',#14795) ;
#3881=VERTEX_POINT('',#15245) ;
#3882=VERTEX_POINT('',#15344) ;
#3883=VERTEX_POINT('',#15346) ;
#3884=VERTEX_POINT('',#15803) ;
#3885=VERTEX_POINT('',#15809) ;
#3886=VERTEX_POINT('',#15812) ;
#3887=VERTEX_POINT('',#15817) ;
#3888=VERTEX_POINT('',#15818) ;
#3889=VERTEX_POINT('',#15822) ;
#3890=VERTEX_POINT('',#15824) ;
#3891=VERTEX_POINT('',#15828) ;
#3892=VERTEX_POINT('',#15832) ;
#3893=VERTEX_POINT('',#15838) ;
#3894=VERTEX_POINT('',#15840) ;
#3895=VERTEX_POINT('',#15842) ;
#3896=VERTEX_POINT('',#15844) ;
#3897=VERTEX_POINT('',#15846) ;
#3898=VERTEX_POINT('',#15848) ;
#3899=VERTEX_POINT('',#15850) ;
#3900=VERTEX_POINT('',#15852) ;
#3901=VERTEX_POINT('',#15854) ;
#3902=VERTEX_POINT('',#15856) ;
#3903=VERTEX_POINT('',#15858) ;
#3904=VERTEX_POINT('',#15860) ;
#3905=VERTEX_POINT('',#15862) ;
#3906=VERTEX_POINT('',#15864) ;
#3907=VERTEX_POINT('',#15866) ;
#3908=VERTEX_POINT('',#15868) ;
#3909=VERTEX_POINT('',#15870) ;
#3910=VERTEX_POINT('',#15872) ;
#3911=VERTEX_POINT('',#15874) ;
#3912=VERTEX_POINT('',#15876) ;
#3913=VERTEX_POINT('',#15878) ;
#3914=VERTEX_POINT('',#15880) ;
#3915=VERTEX_POINT('',#15882) ;
#3916=VERTEX_POINT('',#15884) ;
#3917=VERTEX_POINT('',#15886) ;
#3918=VERTEX_POINT('',#15888) ;
#3919=VERTEX_POINT('',#15890) ;
#3920=VERTEX_POINT('',#15892) ;
#3921=VERTEX_POINT('',#15894) ;
#3922=VERTEX_POINT('',#15896) ;
#3923=VERTEX_POINT('',#15898) ;
#3924=VERTEX_POINT('',#15900) ;
#3925=VERTEX_POINT('',#15902) ;
#3926=VERTEX_POINT('',#15904) ;
#3927=VERTEX_POINT('',#15906) ;
#3928=VERTEX_POINT('',#15908) ;
#3929=VERTEX_POINT('',#15910) ;
#3930=VERTEX_POINT('',#15912) ;
#3931=VERTEX_POINT('',#15914) ;
#3932=VERTEX_POINT('',#15916) ;
#3933=VERTEX_POINT('',#15918) ;
#3934=VERTEX_POINT('',#15920) ;
#3935=VERTEX_POINT('',#15922) ;
#3936=VERTEX_POINT('',#15924) ;
#3937=VERTEX_POINT('',#15926) ;
#3938=VERTEX_POINT('',#15928) ;
#3939=VERTEX_POINT('',#15930) ;
#3940=VERTEX_POINT('',#15932) ;
#3941=VERTEX_POINT('',#15934) ;
#3942=VERTEX_POINT('',#15936) ;
#3943=VERTEX_POINT('',#15938) ;
#3944=VERTEX_POINT('',#15940) ;
#3945=VERTEX_POINT('',#15942) ;
#3946=VERTEX_POINT('',#15944) ;
#3947=VERTEX_POINT('',#15946) ;
#3948=VERTEX_POINT('',#15948) ;
#3949=VERTEX_POINT('',#15950) ;
#3950=VERTEX_POINT('',#15952) ;
#3951=VERTEX_POINT('',#15954) ;
#3952=VERTEX_POINT('',#15956) ;
#3953=VERTEX_POINT('',#15958) ;
#3954=VERTEX_POINT('',#15960) ;
#3955=VERTEX_POINT('',#15962) ;
#3956=VERTEX_POINT('',#15964) ;
#3957=VERTEX_POINT('',#15966) ;
#3958=VERTEX_POINT('',#15968) ;
#3959=VERTEX_POINT('',#15970) ;
#3960=VERTEX_POINT('',#15972) ;
#3961=VERTEX_POINT('',#15974) ;
#3962=VERTEX_POINT('',#15976) ;
#3963=VERTEX_POINT('',#15978) ;
#3964=VERTEX_POINT('',#15980) ;
#3965=VERTEX_POINT('',#15982) ;
#3966=VERTEX_POINT('',#15984) ;
#3967=VERTEX_POINT('',#15986) ;
#3968=VERTEX_POINT('',#15988) ;
#3969=VERTEX_POINT('',#15990) ;
#3970=VERTEX_POINT('',#15992) ;
#3971=VERTEX_POINT('',#15994) ;
#3972=VERTEX_POINT('',#15996) ;
#3973=VERTEX_POINT('',#15998) ;
#3974=VERTEX_POINT('',#16000) ;
#3975=VERTEX_POINT('',#16002) ;
#3976=VERTEX_POINT('',#16004) ;
#3977=VERTEX_POINT('',#16006) ;
#3978=VERTEX_POINT('',#16008) ;
#3979=VERTEX_POINT('',#16010) ;
#3980=VERTEX_POINT('',#16012) ;
#3981=VERTEX_POINT('',#16014) ;
#3982=VERTEX_POINT('',#16016) ;
#3983=VERTEX_POINT('',#16018) ;
#3984=VERTEX_POINT('',#16020) ;
#3985=VERTEX_POINT('',#16022) ;
#3986=VERTEX_POINT('',#16024) ;
#3987=VERTEX_POINT('',#16026) ;
#3988=VERTEX_POINT('',#16028) ;
#3989=VERTEX_POINT('',#16030) ;
#3990=VERTEX_POINT('',#16032) ;
#3991=VERTEX_POINT('',#16034) ;
#3992=VERTEX_POINT('',#16036) ;
#3993=VERTEX_POINT('',#16038) ;
#3994=VERTEX_POINT('',#16040) ;
#3995=VERTEX_POINT('',#16042) ;
#3996=VERTEX_POINT('',#16044) ;
#3997=VERTEX_POINT('',#16046) ;
#3998=VERTEX_POINT('',#16048) ;
#3999=VERTEX_POINT('',#16050) ;
#4000=VERTEX_POINT('',#16052) ;
#4001=VERTEX_POINT('',#16054) ;
#4002=VERTEX_POINT('',#16056) ;
#4003=VERTEX_POINT('',#16058) ;
#4004=VERTEX_POINT('',#16060) ;
#4005=VERTEX_POINT('',#16063) ;
#4006=VERTEX_POINT('',#16065) ;
#4007=VERTEX_POINT('',#16067) ;
#4008=VERTEX_POINT('',#16069) ;
#4009=VERTEX_POINT('',#16071) ;
#4010=VERTEX_POINT('',#16073) ;
#4011=VERTEX_POINT('',#16075) ;
#4012=VERTEX_POINT('',#16077) ;
#4013=VERTEX_POINT('',#16079) ;
#4014=VERTEX_POINT('',#16081) ;
#4015=VERTEX_POINT('',#16083) ;
#4016=VERTEX_POINT('',#16085) ;
#4017=VERTEX_POINT('',#16087) ;
#4018=VERTEX_POINT('',#16089) ;
#4019=VERTEX_POINT('',#16091) ;
#4020=VERTEX_POINT('',#16093) ;
#4021=VERTEX_POINT('',#16095) ;
#4022=VERTEX_POINT('',#16097) ;
#4023=VERTEX_POINT('',#16099) ;
#4024=VERTEX_POINT('',#16101) ;
#4025=VERTEX_POINT('',#16103) ;
#4026=VERTEX_POINT('',#16105) ;
#4027=VERTEX_POINT('',#16107) ;
#4028=VERTEX_POINT('',#16109) ;
#4029=VERTEX_POINT('',#16111) ;
#4030=VERTEX_POINT('',#16113) ;
#4031=VERTEX_POINT('',#16115) ;
#4032=VERTEX_POINT('',#16117) ;
#4033=VERTEX_POINT('',#16119) ;
#4034=VERTEX_POINT('',#16121) ;
#4035=VERTEX_POINT('',#16125) ;
#4036=VERTEX_POINT('',#16129) ;
#4037=VERTEX_POINT('',#16139) ;
#4038=VERTEX_POINT('',#16143) ;
#4039=VERTEX_POINT('',#16153) ;
#4040=VERTEX_POINT('',#16157) ;
#4041=VERTEX_POINT('',#16167) ;
#4042=VERTEX_POINT('',#16171) ;
#4043=VERTEX_POINT('',#16181) ;
#4044=VERTEX_POINT('',#16185) ;
#4045=VERTEX_POINT('',#16195) ;
#4046=VERTEX_POINT('',#16199) ;
#4047=VERTEX_POINT('',#16209) ;
#4048=VERTEX_POINT('',#16213) ;
#4049=VERTEX_POINT('',#16223) ;
#4050=VERTEX_POINT('',#16227) ;
#4051=VERTEX_POINT('',#16237) ;
#4052=VERTEX_POINT('',#16241) ;
#4053=VERTEX_POINT('',#16251) ;
#4054=VERTEX_POINT('',#16255) ;
#4055=VERTEX_POINT('',#16265) ;
#4056=VERTEX_POINT('',#16269) ;
#4057=VERTEX_POINT('',#16279) ;
#4058=VERTEX_POINT('',#16283) ;
#4059=VERTEX_POINT('',#16293) ;
#4060=VERTEX_POINT('',#16297) ;
#4061=VERTEX_POINT('',#16307) ;
#4062=VERTEX_POINT('',#16311) ;
#4063=VERTEX_POINT('',#16321) ;
#4064=VERTEX_POINT('',#16325) ;
#4065=VERTEX_POINT('',#16335) ;
#4066=VERTEX_POINT('',#16339) ;
#4067=VERTEX_POINT('',#16349) ;
#4068=VERTEX_POINT('',#16353) ;
#4069=VERTEX_POINT('',#16363) ;
#4070=VERTEX_POINT('',#16367) ;
#4071=VERTEX_POINT('',#16377) ;
#4072=VERTEX_POINT('',#16381) ;
#4073=VERTEX_POINT('',#16391) ;
#4074=VERTEX_POINT('',#16395) ;
#4075=VERTEX_POINT('',#16405) ;
#4076=VERTEX_POINT('',#16409) ;
#4077=VERTEX_POINT('',#16419) ;
#4078=VERTEX_POINT('',#16423) ;
#4079=VERTEX_POINT('',#16433) ;
#4080=VERTEX_POINT('',#16437) ;
#4081=VERTEX_POINT('',#16447) ;
#4082=VERTEX_POINT('',#16451) ;
#4083=VERTEX_POINT('',#16461) ;
#4084=VERTEX_POINT('',#16465) ;
#4085=VERTEX_POINT('',#16475) ;
#4086=VERTEX_POINT('',#16479) ;
#4087=VERTEX_POINT('',#16489) ;
#4088=VERTEX_POINT('',#16493) ;
#4089=VERTEX_POINT('',#16503) ;
#4090=VERTEX_POINT('',#16507) ;
#4091=VERTEX_POINT('',#16517) ;
#4092=VERTEX_POINT('',#16521) ;
#4093=VERTEX_POINT('',#16531) ;
#4094=VERTEX_POINT('',#16535) ;
#4095=VERTEX_POINT('',#16545) ;
#4096=VERTEX_POINT('',#16549) ;
#4097=VERTEX_POINT('',#16559) ;
#4098=VERTEX_POINT('',#16563) ;
#4099=VERTEX_POINT('',#16573) ;
#4100=VERTEX_POINT('',#16577) ;
#4101=VERTEX_POINT('',#16587) ;
#4102=VERTEX_POINT('',#16591) ;
#4103=VERTEX_POINT('',#16601) ;
#4104=VERTEX_POINT('',#16605) ;
#4105=VERTEX_POINT('',#16617) ;
#4106=VERTEX_POINT('',#16621) ;
#4107=VERTEX_POINT('',#16624) ;
#4108=VERTEX_POINT('',#16625) ;
#4109=VERTEX_POINT('',#16629) ;
#4110=VERTEX_POINT('',#16631) ;
#4111=VERTEX_POINT('',#16635) ;
#4112=VERTEX_POINT('',#16639) ;
#4113=VERTEX_POINT('',#16641) ;
#4114=VERTEX_POINT('',#16645) ;
#4115=VERTEX_POINT('',#16649) ;
#4116=VERTEX_POINT('',#16651) ;
#4117=VERTEX_POINT('',#16655) ;
#4118=VERTEX_POINT('',#16659) ;
#4119=VERTEX_POINT('',#16661) ;
#4120=VERTEX_POINT('',#16665) ;
#4121=VERTEX_POINT('',#16669) ;
#4122=VERTEX_POINT('',#16671) ;
#4123=VERTEX_POINT('',#16676) ;
#4124=VERTEX_POINT('',#16680) ;
#4125=VERTEX_POINT('',#16686) ;
#4126=VERTEX_POINT('',#16688) ;
#4127=VERTEX_POINT('',#16692) ;
#4128=VERTEX_POINT('',#16694) ;
#4129=VERTEX_POINT('',#16698) ;
#4130=VERTEX_POINT('',#16700) ;
#4131=VERTEX_POINT('',#16704) ;
#4132=VERTEX_POINT('',#16706) ;
#4133=VERTEX_POINT('',#16710) ;
#4134=VERTEX_POINT('',#16712) ;
#4135=VERTEX_POINT('',#16716) ;
#4136=VERTEX_POINT('',#16718) ;
#4137=VERTEX_POINT('',#16723) ;
#4138=VERTEX_POINT('',#16725) ;
#4139=VERTEX_POINT('',#16730) ;
#4140=VERTEX_POINT('',#16735) ;
#4141=VERTEX_POINT('',#16748) ;
#4142=VERTEX_POINT('',#16749) ;
#4143=VERTEX_POINT('',#16765) ;
#4811=EDGE_CURVE('',#3821,#3822,#2287,.T.) ;
#4812=EDGE_CURVE('',#3821,#3823,#625,.T.) ;
#4813=EDGE_CURVE('',#3824,#3823,#3274,.T.) ;
#4814=EDGE_CURVE('',#3824,#3822,#626,.T.) ;
#4815=EDGE_CURVE('',#3825,#3826,#2288,.T.) ;
#4816=EDGE_CURVE('',#3825,#3821,#627,.T.) ;
#4817=EDGE_CURVE('',#3822,#3826,#628,.T.) ;
#4818=EDGE_CURVE('',#3827,#3828,#2289,.T.) ;
#4819=EDGE_CURVE('',#3827,#3825,#629,.T.) ;
#4820=EDGE_CURVE('',#3826,#3828,#630,.T.) ;
#4821=EDGE_CURVE('',#3829,#3830,#2290,.T.) ;
#4822=EDGE_CURVE('',#3829,#3827,#631,.T.) ;
#4823=EDGE_CURVE('',#3828,#3830,#632,.T.) ;
#4824=EDGE_CURVE('',#3831,#3832,#2291,.T.) ;
#4825=EDGE_CURVE('',#3831,#3829,#633,.T.) ;
#4826=EDGE_CURVE('',#3830,#3832,#634,.T.) ;
#4827=EDGE_CURVE('',#3833,#3834,#2292,.T.) ;
#4828=EDGE_CURVE('',#3833,#3831,#635,.T.) ;
#4829=EDGE_CURVE('',#3832,#3834,#636,.T.) ;
#4830=EDGE_CURVE('',#3835,#3836,#2293,.T.) ;
#4831=EDGE_CURVE('',#3835,#3833,#637,.T.) ;
#4832=EDGE_CURVE('',#3834,#3836,#638,.T.) ;
#4833=EDGE_CURVE('',#3837,#3838,#2294,.T.) ;
#4834=EDGE_CURVE('',#3837,#3835,#639,.T.) ;
#4835=EDGE_CURVE('',#3836,#3838,#640,.T.) ;
#4836=EDGE_CURVE('',#3839,#3840,#2295,.T.) ;
#4837=EDGE_CURVE('',#3839,#3837,#641,.T.) ;
#4838=EDGE_CURVE('',#3838,#3840,#642,.T.) ;
#4839=EDGE_CURVE('',#3841,#3842,#2296,.T.) ;
#4840=EDGE_CURVE('',#3841,#3839,#643,.T.) ;
#4841=EDGE_CURVE('',#3840,#3842,#644,.T.) ;
#4842=EDGE_CURVE('',#3843,#3844,#2297,.T.) ;
#4843=EDGE_CURVE('',#3843,#3841,#645,.T.) ;
#4844=EDGE_CURVE('',#3842,#3844,#646,.T.) ;
#4845=EDGE_CURVE('',#3845,#3846,#2298,.T.) ;
#4846=EDGE_CURVE('',#3845,#3843,#647,.T.) ;
#4847=EDGE_CURVE('',#3844,#3846,#648,.T.) ;
#4848=EDGE_CURVE('',#3847,#3848,#2299,.T.) ;
#4849=EDGE_CURVE('',#3847,#3845,#649,.T.) ;
#4850=EDGE_CURVE('',#3846,#3848,#650,.T.) ;
#4851=EDGE_CURVE('',#3849,#3850,#2300,.T.) ;
#4852=EDGE_CURVE('',#3851,#3849,#3275,.T.) ;
#4853=EDGE_CURVE('',#3851,#3847,#651,.T.) ;
#4854=EDGE_CURVE('',#3848,#3850,#652,.T.) ;
#4855=EDGE_CURVE('',#3852,#3853,#2301,.T.) ;
#4856=EDGE_CURVE('',#3852,#3854,#653,.T.) ;
#4857=EDGE_CURVE('',#3855,#3854,#3276,.T.) ;
#4858=EDGE_CURVE('',#3853,#3855,#654,.T.) ;
#4859=EDGE_CURVE('',#3856,#3857,#2302,.T.) ;
#4860=EDGE_CURVE('',#3856,#3852,#655,.T.) ;
#4861=EDGE_CURVE('',#3857,#3853,#656,.T.) ;
#4862=EDGE_CURVE('',#3858,#3859,#2303,.T.) ;
#4863=EDGE_CURVE('',#3858,#3856,#657,.T.) ;
#4864=EDGE_CURVE('',#3859,#3857,#658,.T.) ;
#4865=EDGE_CURVE('',#3860,#3861,#2304,.T.) ;
#4866=EDGE_CURVE('',#3860,#3858,#659,.T.) ;
#4867=EDGE_CURVE('',#3861,#3859,#660,.T.) ;
#4868=EDGE_CURVE('',#3862,#3863,#2305,.T.) ;
#4869=EDGE_CURVE('',#3862,#3860,#661,.T.) ;
#4870=EDGE_CURVE('',#3863,#3861,#662,.T.) ;
#4871=EDGE_CURVE('',#3864,#3865,#2306,.T.) ;
#4872=EDGE_CURVE('',#3864,#3862,#663,.T.) ;
#4873=EDGE_CURVE('',#3865,#3863,#664,.T.) ;
#4874=EDGE_CURVE('',#3866,#3867,#2307,.T.) ;
#4875=EDGE_CURVE('',#3866,#3864,#665,.T.) ;
#4876=EDGE_CURVE('',#3867,#3865,#666,.T.) ;
#4877=EDGE_CURVE('',#3868,#3869,#2308,.T.) ;
#4878=EDGE_CURVE('',#3868,#3866,#667,.T.) ;
#4879=EDGE_CURVE('',#3869,#3867,#668,.T.) ;
#4880=EDGE_CURVE('',#3870,#3871,#2309,.T.) ;
#4881=EDGE_CURVE('',#3870,#3868,#669,.T.) ;
#4882=EDGE_CURVE('',#3871,#3869,#670,.T.) ;
#4883=EDGE_CURVE('',#3872,#3873,#2310,.T.) ;
#4884=EDGE_CURVE('',#3872,#3870,#671,.T.) ;
#4885=EDGE_CURVE('',#3873,#3871,#672,.T.) ;
#4886=EDGE_CURVE('',#3874,#3875,#2311,.T.) ;
#4887=EDGE_CURVE('',#3874,#3872,#673,.T.) ;
#4888=EDGE_CURVE('',#3875,#3873,#674,.T.) ;
#4889=EDGE_CURVE('',#3876,#3877,#2312,.T.) ;
#4890=EDGE_CURVE('',#3876,#3874,#675,.T.) ;
#4891=EDGE_CURVE('',#3877,#3875,#676,.T.) ;
#4892=EDGE_CURVE('',#3878,#3879,#2313,.T.) ;
#4893=EDGE_CURVE('',#3878,#3876,#677,.T.) ;
#4894=EDGE_CURVE('',#3879,#3877,#678,.T.) ;
#4895=EDGE_CURVE('',#3854,#3851,#679,.T.) ;
#4896=EDGE_CURVE('',#3880,#3851,#3277,.T.) ;
#4897=EDGE_CURVE('',#3880,#3855,#680,.T.) ;
#4898=EDGE_CURVE('',#3850,#3880,#681,.T.) ;
#4899=EDGE_CURVE('',#3881,#3824,#682,.T.) ;
#4900=EDGE_CURVE('',#3881,#3879,#683,.T.) ;
#4901=EDGE_CURVE('',#3823,#3882,#3278,.T.) ;
#4902=EDGE_CURVE('',#3823,#3883,#684,.T.) ;
#4903=EDGE_CURVE('',#3883,#3881,#3279,.T.) ;
#4904=EDGE_CURVE('',#3882,#3824,#3280,.T.) ;
#4905=EDGE_CURVE('',#3883,#3878,#685,.T.) ;
#4906=EDGE_CURVE('',#3882,#3884,#3281,.T.) ;
#4907=EDGE_CURVE('',#3884,#3884,#3282,.T.) ;
#4908=EDGE_CURVE('',#3849,#3880,#3283,.T.) ;
#4909=EDGE_CURVE('',#3885,#3885,#3284,.T.) ;
#4910=EDGE_CURVE('',#3849,#3886,#2314,.T.) ;
#4911=EDGE_CURVE('',#3886,#3886,#3285,.T.) ;
#4912=EDGE_CURVE('',#3887,#3888,#231,.T.) ;
#4913=EDGE_CURVE('',#3887,#3889,#2315,.T.) ;
#4914=EDGE_CURVE('',#3889,#3890,#2316,.T.) ;
#4915=EDGE_CURVE('',#3888,#3890,#2317,.T.) ;
#4916=EDGE_CURVE('',#3890,#3891,#3286,.T.) ;
#4917=EDGE_CURVE('',#3891,#3889,#2318,.T.) ;
#4918=EDGE_CURVE('',#3892,#3887,#232,.T.) ;
#4919=EDGE_CURVE('',#3891,#3892,#2319,.T.) ;
#4920=EDGE_CURVE('',#3893,#3892,#3287,.T.) ;
#4921=EDGE_CURVE('',#3893,#3894,#2320,.T.) ;
#4922=EDGE_CURVE('',#3894,#3895,#3288,.T.) ;
#4923=EDGE_CURVE('',#3895,#3896,#2321,.T.) ;
#4924=EDGE_CURVE('',#3897,#3896,#3289,.T.) ;
#4925=EDGE_CURVE('',#3897,#3898,#2322,.T.) ;
#4926=EDGE_CURVE('',#3898,#3899,#3290,.T.) ;
#4927=EDGE_CURVE('',#3899,#3900,#2323,.T.) ;
#4928=EDGE_CURVE('',#3901,#3900,#3291,.T.) ;
#4929=EDGE_CURVE('',#3901,#3902,#2324,.T.) ;
#4930=EDGE_CURVE('',#3902,#3903,#3292,.T.) ;
#4931=EDGE_CURVE('',#3903,#3904,#2325,.T.) ;
#4932=EDGE_CURVE('',#3905,#3904,#3293,.T.) ;
#4933=EDGE_CURVE('',#3905,#3906,#2326,.T.) ;
#4934=EDGE_CURVE('',#3906,#3907,#3294,.T.) ;
#4935=EDGE_CURVE('',#3907,#3908,#2327,.T.) ;
#4936=EDGE_CURVE('',#3909,#3908,#3295,.T.) ;
#4937=EDGE_CURVE('',#3909,#3910,#2328,.T.) ;
#4938=EDGE_CURVE('',#3910,#3911,#3296,.T.) ;
#4939=EDGE_CURVE('',#3911,#3912,#2329,.T.) ;
#4940=EDGE_CURVE('',#3913,#3912,#3297,.T.) ;
#4941=EDGE_CURVE('',#3913,#3914,#2330,.T.) ;
#4942=EDGE_CURVE('',#3914,#3915,#3298,.T.) ;
#4943=EDGE_CURVE('',#3915,#3916,#2331,.T.) ;
#4944=EDGE_CURVE('',#3917,#3916,#3299,.T.) ;
#4945=EDGE_CURVE('',#3917,#3918,#2332,.T.) ;
#4946=EDGE_CURVE('',#3918,#3919,#3300,.T.) ;
#4947=EDGE_CURVE('',#3919,#3920,#2333,.T.) ;
#4948=EDGE_CURVE('',#3921,#3920,#3301,.T.) ;
#4949=EDGE_CURVE('',#3921,#3922,#2334,.T.) ;
#4950=EDGE_CURVE('',#3922,#3923,#3302,.T.) ;
#4951=EDGE_CURVE('',#3923,#3924,#2335,.T.) ;
#4952=EDGE_CURVE('',#3925,#3924,#3303,.T.) ;
#4953=EDGE_CURVE('',#3925,#3926,#2336,.T.) ;
#4954=EDGE_CURVE('',#3926,#3927,#3304,.T.) ;
#4955=EDGE_CURVE('',#3927,#3928,#2337,.T.) ;
#4956=EDGE_CURVE('',#3929,#3928,#3305,.T.) ;
#4957=EDGE_CURVE('',#3929,#3930,#2338,.T.) ;
#4958=EDGE_CURVE('',#3930,#3931,#3306,.T.) ;
#4959=EDGE_CURVE('',#3931,#3932,#2339,.T.) ;
#4960=EDGE_CURVE('',#3933,#3932,#3307,.T.) ;
#4961=EDGE_CURVE('',#3933,#3934,#2340,.T.) ;
#4962=EDGE_CURVE('',#3934,#3935,#3308,.T.) ;
#4963=EDGE_CURVE('',#3935,#3936,#2341,.T.) ;
#4964=EDGE_CURVE('',#3937,#3936,#3309,.T.) ;
#4965=EDGE_CURVE('',#3937,#3938,#2342,.T.) ;
#4966=EDGE_CURVE('',#3938,#3939,#3310,.T.) ;
#4967=EDGE_CURVE('',#3939,#3940,#2343,.T.) ;
#4968=EDGE_CURVE('',#3941,#3940,#3311,.T.) ;
#4969=EDGE_CURVE('',#3941,#3942,#2344,.T.) ;
#4970=EDGE_CURVE('',#3942,#3943,#3312,.T.) ;
#4971=EDGE_CURVE('',#3943,#3944,#2345,.T.) ;
#4972=EDGE_CURVE('',#3945,#3944,#3313,.T.) ;
#4973=EDGE_CURVE('',#3945,#3946,#2346,.T.) ;
#4974=EDGE_CURVE('',#3946,#3947,#3314,.T.) ;
#4975=EDGE_CURVE('',#3947,#3948,#2347,.T.) ;
#4976=EDGE_CURVE('',#3949,#3948,#3315,.T.) ;
#4977=EDGE_CURVE('',#3949,#3950,#2348,.T.) ;
#4978=EDGE_CURVE('',#3950,#3951,#3316,.T.) ;
#4979=EDGE_CURVE('',#3951,#3952,#2349,.T.) ;
#4980=EDGE_CURVE('',#3953,#3952,#3317,.T.) ;
#4981=EDGE_CURVE('',#3953,#3954,#2350,.T.) ;
#4982=EDGE_CURVE('',#3954,#3955,#3318,.T.) ;
#4983=EDGE_CURVE('',#3955,#3956,#2351,.T.) ;
#4984=EDGE_CURVE('',#3957,#3956,#3319,.T.) ;
#4985=EDGE_CURVE('',#3957,#3958,#2352,.T.) ;
#4986=EDGE_CURVE('',#3958,#3959,#3320,.T.) ;
#4987=EDGE_CURVE('',#3959,#3960,#2353,.T.) ;
#4988=EDGE_CURVE('',#3961,#3960,#3321,.T.) ;
#4989=EDGE_CURVE('',#3961,#3962,#2354,.T.) ;
#4990=EDGE_CURVE('',#3962,#3963,#3322,.T.) ;
#4991=EDGE_CURVE('',#3963,#3964,#2355,.T.) ;
#4992=EDGE_CURVE('',#3965,#3964,#3323,.T.) ;
#4993=EDGE_CURVE('',#3965,#3966,#2356,.T.) ;
#4994=EDGE_CURVE('',#3966,#3967,#3324,.T.) ;
#4995=EDGE_CURVE('',#3967,#3968,#2357,.T.) ;
#4996=EDGE_CURVE('',#3969,#3968,#3325,.T.) ;
#4997=EDGE_CURVE('',#3969,#3970,#2358,.T.) ;
#4998=EDGE_CURVE('',#3970,#3971,#3326,.T.) ;
#4999=EDGE_CURVE('',#3971,#3972,#2359,.T.) ;
#5000=EDGE_CURVE('',#3973,#3972,#3327,.T.) ;
#5001=EDGE_CURVE('',#3973,#3974,#2360,.T.) ;
#5002=EDGE_CURVE('',#3974,#3975,#3328,.T.) ;
#5003=EDGE_CURVE('',#3975,#3976,#2361,.T.) ;
#5004=EDGE_CURVE('',#3977,#3976,#3329,.T.) ;
#5005=EDGE_CURVE('',#3977,#3978,#2362,.T.) ;
#5006=EDGE_CURVE('',#3978,#3979,#3330,.T.) ;
#5007=EDGE_CURVE('',#3979,#3980,#2363,.T.) ;
#5008=EDGE_CURVE('',#3981,#3980,#3331,.T.) ;
#5009=EDGE_CURVE('',#3981,#3982,#2364,.T.) ;
#5010=EDGE_CURVE('',#3982,#3983,#3332,.T.) ;
#5011=EDGE_CURVE('',#3983,#3984,#2365,.T.) ;
#5012=EDGE_CURVE('',#3985,#3984,#3333,.T.) ;
#5013=EDGE_CURVE('',#3985,#3986,#2366,.T.) ;
#5014=EDGE_CURVE('',#3986,#3987,#3334,.T.) ;
#5015=EDGE_CURVE('',#3987,#3988,#2367,.T.) ;
#5016=EDGE_CURVE('',#3989,#3988,#3335,.T.) ;
#5017=EDGE_CURVE('',#3989,#3990,#2368,.T.) ;
#5018=EDGE_CURVE('',#3990,#3991,#3336,.T.) ;
#5019=EDGE_CURVE('',#3991,#3992,#2369,.T.) ;
#5020=EDGE_CURVE('',#3993,#3992,#3337,.T.) ;
#5021=EDGE_CURVE('',#3993,#3994,#2370,.T.) ;
#5022=EDGE_CURVE('',#3994,#3995,#3338,.T.) ;
#5023=EDGE_CURVE('',#3995,#3996,#2371,.T.) ;
#5024=EDGE_CURVE('',#3997,#3996,#3339,.T.) ;
#5025=EDGE_CURVE('',#3997,#3998,#2372,.T.) ;
#5026=EDGE_CURVE('',#3998,#3999,#3340,.T.) ;
#5027=EDGE_CURVE('',#3999,#4000,#2373,.T.) ;
#5028=EDGE_CURVE('',#4001,#4000,#3341,.T.) ;
#5029=EDGE_CURVE('',#4001,#4002,#2374,.T.) ;
#5030=EDGE_CURVE('',#4002,#4003,#3342,.T.) ;
#5031=EDGE_CURVE('',#4003,#4004,#2375,.T.) ;
#5032=EDGE_CURVE('',#4004,#4004,#3343,.T.) ;
#5033=EDGE_CURVE('',#4003,#4005,#3344,.T.) ;
#5034=EDGE_CURVE('',#4005,#4006,#2376,.T.) ;
#5035=EDGE_CURVE('',#4007,#4006,#3345,.T.) ;
#5036=EDGE_CURVE('',#4007,#4008,#2377,.T.) ;
#5037=EDGE_CURVE('',#4008,#4009,#3346,.T.) ;
#5038=EDGE_CURVE('',#4009,#4010,#2378,.T.) ;
#5039=EDGE_CURVE('',#4011,#4010,#3347,.T.) ;
#5040=EDGE_CURVE('',#4011,#4012,#2379,.T.) ;
#5041=EDGE_CURVE('',#4012,#4013,#3348,.T.) ;
#5042=EDGE_CURVE('',#4013,#4014,#2380,.T.) ;
#5043=EDGE_CURVE('',#4015,#4014,#3349,.T.) ;
#5044=EDGE_CURVE('',#4015,#4016,#2381,.T.) ;
#5045=EDGE_CURVE('',#4016,#4017,#3350,.T.) ;
#5046=EDGE_CURVE('',#4017,#4018,#2382,.T.) ;
#5047=EDGE_CURVE('',#4019,#4018,#3351,.T.) ;
#5048=EDGE_CURVE('',#4019,#4020,#2383,.T.) ;
#5049=EDGE_CURVE('',#4020,#4021,#3352,.T.) ;
#5050=EDGE_CURVE('',#4021,#4022,#2384,.T.) ;
#5051=EDGE_CURVE('',#4023,#4022,#3353,.T.) ;
#5052=EDGE_CURVE('',#4023,#4024,#2385,.T.) ;
#5053=EDGE_CURVE('',#4024,#4025,#3354,.T.) ;
#5054=EDGE_CURVE('',#4025,#4026,#2386,.T.) ;
#5055=EDGE_CURVE('',#4027,#4026,#3355,.T.) ;
#5056=EDGE_CURVE('',#4027,#4028,#2387,.T.) ;
#5057=EDGE_CURVE('',#4028,#4029,#3356,.T.) ;
#5058=EDGE_CURVE('',#4029,#4030,#2388,.T.) ;
#5059=EDGE_CURVE('',#4031,#4030,#3357,.T.) ;
#5060=EDGE_CURVE('',#4031,#4032,#2389,.T.) ;
#5061=EDGE_CURVE('',#4032,#4033,#3358,.T.) ;
#5062=EDGE_CURVE('',#4033,#4034,#2390,.T.) ;
#5063=EDGE_CURVE('',#3888,#4034,#3359,.T.) ;
#5064=EDGE_CURVE('',#4035,#4031,#233,.T.) ;
#5065=EDGE_CURVE('',#4035,#4036,#2391,.T.) ;
#5066=EDGE_CURVE('',#4036,#4032,#2392,.T.) ;
#5067=EDGE_CURVE('',#4033,#4036,#2393,.T.) ;
#5068=EDGE_CURVE('',#4034,#4035,#234,.T.) ;
#5069=EDGE_CURVE('',#4037,#4027,#235,.T.) ;
#5070=EDGE_CURVE('',#4037,#4038,#2394,.T.) ;
#5071=EDGE_CURVE('',#4038,#4028,#2395,.T.) ;
#5072=EDGE_CURVE('',#4029,#4038,#2396,.T.) ;
#5073=EDGE_CURVE('',#4030,#4037,#236,.T.) ;
#5074=EDGE_CURVE('',#4039,#4023,#237,.T.) ;
#5075=EDGE_CURVE('',#4039,#4040,#2397,.T.) ;
#5076=EDGE_CURVE('',#4040,#4024,#2398,.T.) ;
#5077=EDGE_CURVE('',#4025,#4040,#2399,.T.) ;
#5078=EDGE_CURVE('',#4026,#4039,#238,.T.) ;
#5079=EDGE_CURVE('',#4041,#4019,#239,.T.) ;
#5080=EDGE_CURVE('',#4041,#4042,#2400,.T.) ;
#5081=EDGE_CURVE('',#4042,#4020,#2401,.T.) ;
#5082=EDGE_CURVE('',#4021,#4042,#2402,.T.) ;
#5083=EDGE_CURVE('',#4022,#4041,#240,.T.) ;
#5084=EDGE_CURVE('',#4043,#4015,#241,.T.) ;
#5085=EDGE_CURVE('',#4043,#4044,#2403,.T.) ;
#5086=EDGE_CURVE('',#4044,#4016,#2404,.T.) ;
#5087=EDGE_CURVE('',#4017,#4044,#2405,.T.) ;
#5088=EDGE_CURVE('',#4018,#4043,#242,.T.) ;
#5089=EDGE_CURVE('',#4045,#4011,#243,.T.) ;
#5090=EDGE_CURVE('',#4045,#4046,#2406,.T.) ;
#5091=EDGE_CURVE('',#4046,#4012,#2407,.T.) ;
#5092=EDGE_CURVE('',#4013,#4046,#2408,.T.) ;
#5093=EDGE_CURVE('',#4014,#4045,#244,.T.) ;
#5094=EDGE_CURVE('',#4047,#4007,#245,.T.) ;
#5095=EDGE_CURVE('',#4047,#4048,#2409,.T.) ;
#5096=EDGE_CURVE('',#4048,#4008,#2410,.T.) ;
#5097=EDGE_CURVE('',#4009,#4048,#2411,.T.) ;
#5098=EDGE_CURVE('',#4010,#4047,#246,.T.) ;
#5099=EDGE_CURVE('',#4049,#4001,#247,.T.) ;
#5100=EDGE_CURVE('',#4049,#4050,#2412,.T.) ;
#5101=EDGE_CURVE('',#4050,#4002,#2413,.T.) ;
#5102=EDGE_CURVE('',#4005,#4050,#2414,.T.) ;
#5103=EDGE_CURVE('',#4006,#4049,#248,.T.) ;
#5104=EDGE_CURVE('',#4051,#3997,#249,.T.) ;
#5105=EDGE_CURVE('',#4051,#4052,#2415,.T.) ;
#5106=EDGE_CURVE('',#4052,#3998,#2416,.T.) ;
#5107=EDGE_CURVE('',#3999,#4052,#2417,.T.) ;
#5108=EDGE_CURVE('',#4000,#4051,#250,.T.) ;
#5109=EDGE_CURVE('',#4053,#3993,#251,.T.) ;
#5110=EDGE_CURVE('',#4053,#4054,#2418,.T.) ;
#5111=EDGE_CURVE('',#4054,#3994,#2419,.T.) ;
#5112=EDGE_CURVE('',#3995,#4054,#2420,.T.) ;
#5113=EDGE_CURVE('',#3996,#4053,#252,.T.) ;
#5114=EDGE_CURVE('',#4055,#3989,#253,.T.) ;
#5115=EDGE_CURVE('',#4055,#4056,#2421,.T.) ;
#5116=EDGE_CURVE('',#4056,#3990,#2422,.T.) ;
#5117=EDGE_CURVE('',#3991,#4056,#2423,.T.) ;
#5118=EDGE_CURVE('',#3992,#4055,#254,.T.) ;
#5119=EDGE_CURVE('',#4057,#3985,#255,.T.) ;
#5120=EDGE_CURVE('',#4057,#4058,#2424,.T.) ;
#5121=EDGE_CURVE('',#4058,#3986,#2425,.T.) ;
#5122=EDGE_CURVE('',#3987,#4058,#2426,.T.) ;
#5123=EDGE_CURVE('',#3988,#4057,#256,.T.) ;
#5124=EDGE_CURVE('',#4059,#3981,#257,.T.) ;
#5125=EDGE_CURVE('',#4059,#4060,#2427,.T.) ;
#5126=EDGE_CURVE('',#4060,#3982,#2428,.T.) ;
#5127=EDGE_CURVE('',#3983,#4060,#2429,.T.) ;
#5128=EDGE_CURVE('',#3984,#4059,#258,.T.) ;
#5129=EDGE_CURVE('',#4061,#3977,#259,.T.) ;
#5130=EDGE_CURVE('',#4061,#4062,#2430,.T.) ;
#5131=EDGE_CURVE('',#4062,#3978,#2431,.T.) ;
#5132=EDGE_CURVE('',#3979,#4062,#2432,.T.) ;
#5133=EDGE_CURVE('',#3980,#4061,#260,.T.) ;
#5134=EDGE_CURVE('',#4063,#3973,#261,.T.) ;
#5135=EDGE_CURVE('',#4063,#4064,#2433,.T.) ;
#5136=EDGE_CURVE('',#4064,#3974,#2434,.T.) ;
#5137=EDGE_CURVE('',#3975,#4064,#2435,.T.) ;
#5138=EDGE_CURVE('',#3976,#4063,#262,.T.) ;
#5139=EDGE_CURVE('',#4065,#3969,#263,.T.) ;
#5140=EDGE_CURVE('',#4065,#4066,#2436,.T.) ;
#5141=EDGE_CURVE('',#4066,#3970,#2437,.T.) ;
#5142=EDGE_CURVE('',#3971,#4066,#2438,.T.) ;
#5143=EDGE_CURVE('',#3972,#4065,#264,.T.) ;
#5144=EDGE_CURVE('',#4067,#3965,#265,.T.) ;
#5145=EDGE_CURVE('',#4067,#4068,#2439,.T.) ;
#5146=EDGE_CURVE('',#4068,#3966,#2440,.T.) ;
#5147=EDGE_CURVE('',#3967,#4068,#2441,.T.) ;
#5148=EDGE_CURVE('',#3968,#4067,#266,.T.) ;
#5149=EDGE_CURVE('',#4069,#3961,#267,.T.) ;
#5150=EDGE_CURVE('',#4069,#4070,#2442,.T.) ;
#5151=EDGE_CURVE('',#4070,#3962,#2443,.T.) ;
#5152=EDGE_CURVE('',#3963,#4070,#2444,.T.) ;
#5153=EDGE_CURVE('',#3964,#4069,#268,.T.) ;
#5154=EDGE_CURVE('',#4071,#3957,#269,.T.) ;
#5155=EDGE_CURVE('',#4071,#4072,#2445,.T.) ;
#5156=EDGE_CURVE('',#4072,#3958,#2446,.T.) ;
#5157=EDGE_CURVE('',#3959,#4072,#2447,.T.) ;
#5158=EDGE_CURVE('',#3960,#4071,#270,.T.) ;
#5159=EDGE_CURVE('',#4073,#3953,#271,.T.) ;
#5160=EDGE_CURVE('',#4073,#4074,#2448,.T.) ;
#5161=EDGE_CURVE('',#4074,#3954,#2449,.T.) ;
#5162=EDGE_CURVE('',#3955,#4074,#2450,.T.) ;
#5163=EDGE_CURVE('',#3956,#4073,#272,.T.) ;
#5164=EDGE_CURVE('',#4075,#3949,#273,.T.) ;
#5165=EDGE_CURVE('',#4075,#4076,#2451,.T.) ;
#5166=EDGE_CURVE('',#4076,#3950,#2452,.T.) ;
#5167=EDGE_CURVE('',#3951,#4076,#2453,.T.) ;
#5168=EDGE_CURVE('',#3952,#4075,#274,.T.) ;
#5169=EDGE_CURVE('',#4077,#3945,#275,.T.) ;
#5170=EDGE_CURVE('',#4077,#4078,#2454,.T.) ;
#5171=EDGE_CURVE('',#4078,#3946,#2455,.T.) ;
#5172=EDGE_CURVE('',#3947,#4078,#2456,.T.) ;
#5173=EDGE_CURVE('',#3948,#4077,#276,.T.) ;
#5174=EDGE_CURVE('',#4079,#3941,#277,.T.) ;
#5175=EDGE_CURVE('',#4079,#4080,#2457,.T.) ;
#5176=EDGE_CURVE('',#4080,#3942,#2458,.T.) ;
#5177=EDGE_CURVE('',#3943,#4080,#2459,.T.) ;
#5178=EDGE_CURVE('',#3944,#4079,#278,.T.) ;
#5179=EDGE_CURVE('',#4081,#3937,#279,.T.) ;
#5180=EDGE_CURVE('',#4081,#4082,#2460,.T.) ;
#5181=EDGE_CURVE('',#4082,#3938,#2461,.T.) ;
#5182=EDGE_CURVE('',#3939,#4082,#2462,.T.) ;
#5183=EDGE_CURVE('',#3940,#4081,#280,.T.) ;
#5184=EDGE_CURVE('',#4083,#3933,#281,.T.) ;
#5185=EDGE_CURVE('',#4083,#4084,#2463,.T.) ;
#5186=EDGE_CURVE('',#4084,#3934,#2464,.T.) ;
#5187=EDGE_CURVE('',#3935,#4084,#2465,.T.) ;
#5188=EDGE_CURVE('',#3936,#4083,#282,.T.) ;
#5189=EDGE_CURVE('',#4085,#3929,#283,.T.) ;
#5190=EDGE_CURVE('',#4085,#4086,#2466,.T.) ;
#5191=EDGE_CURVE('',#4086,#3930,#2467,.T.) ;
#5192=EDGE_CURVE('',#3931,#4086,#2468,.T.) ;
#5193=EDGE_CURVE('',#3932,#4085,#284,.T.) ;
#5194=EDGE_CURVE('',#4087,#3925,#285,.T.) ;
#5195=EDGE_CURVE('',#4087,#4088,#2469,.T.) ;
#5196=EDGE_CURVE('',#4088,#3926,#2470,.T.) ;
#5197=EDGE_CURVE('',#3927,#4088,#2471,.T.) ;
#5198=EDGE_CURVE('',#3928,#4087,#286,.T.) ;
#5199=EDGE_CURVE('',#4089,#3921,#287,.T.) ;
#5200=EDGE_CURVE('',#4089,#4090,#2472,.T.) ;
#5201=EDGE_CURVE('',#4090,#3922,#2473,.T.) ;
#5202=EDGE_CURVE('',#3923,#4090,#2474,.T.) ;
#5203=EDGE_CURVE('',#3924,#4089,#288,.T.) ;
#5204=EDGE_CURVE('',#4091,#3917,#289,.T.) ;
#5205=EDGE_CURVE('',#4091,#4092,#2475,.T.) ;
#5206=EDGE_CURVE('',#4092,#3918,#2476,.T.) ;
#5207=EDGE_CURVE('',#3919,#4092,#2477,.T.) ;
#5208=EDGE_CURVE('',#3920,#4091,#290,.T.) ;
#5209=EDGE_CURVE('',#4093,#3913,#291,.T.) ;
#5210=EDGE_CURVE('',#4093,#4094,#2478,.T.) ;
#5211=EDGE_CURVE('',#4094,#3914,#2479,.T.) ;
#5212=EDGE_CURVE('',#3915,#4094,#2480,.T.) ;
#5213=EDGE_CURVE('',#3916,#4093,#292,.T.) ;
#5214=EDGE_CURVE('',#4095,#3909,#293,.T.) ;
#5215=EDGE_CURVE('',#4095,#4096,#2481,.T.) ;
#5216=EDGE_CURVE('',#4096,#3910,#2482,.T.) ;
#5217=EDGE_CURVE('',#3911,#4096,#2483,.T.) ;
#5218=EDGE_CURVE('',#3912,#4095,#294,.T.) ;
#5219=EDGE_CURVE('',#4097,#3905,#295,.T.) ;
#5220=EDGE_CURVE('',#4097,#4098,#2484,.T.) ;
#5221=EDGE_CURVE('',#4098,#3906,#2485,.T.) ;
#5222=EDGE_CURVE('',#3907,#4098,#2486,.T.) ;
#5223=EDGE_CURVE('',#3908,#4097,#296,.T.) ;
#5224=EDGE_CURVE('',#4099,#3901,#297,.T.) ;
#5225=EDGE_CURVE('',#4099,#4100,#2487,.T.) ;
#5226=EDGE_CURVE('',#4100,#3902,#2488,.T.) ;
#5227=EDGE_CURVE('',#3903,#4100,#2489,.T.) ;
#5228=EDGE_CURVE('',#3904,#4099,#298,.T.) ;
#5229=EDGE_CURVE('',#4101,#3897,#299,.T.) ;
#5230=EDGE_CURVE('',#4101,#4102,#2490,.T.) ;
#5231=EDGE_CURVE('',#4102,#3898,#2491,.T.) ;
#5232=EDGE_CURVE('',#3899,#4102,#2492,.T.) ;
#5233=EDGE_CURVE('',#3900,#4101,#300,.T.) ;
#5234=EDGE_CURVE('',#4103,#3893,#301,.T.) ;
#5235=EDGE_CURVE('',#4103,#4104,#2493,.T.) ;
#5236=EDGE_CURVE('',#4104,#3894,#2494,.T.) ;
#5237=EDGE_CURVE('',#3895,#4104,#2495,.T.) ;
#5238=EDGE_CURVE('',#3896,#4103,#302,.T.) ;
#5239=EDGE_CURVE('',#4004,#3885,#3360,.T.) ;
#5240=EDGE_CURVE('',#4105,#4105,#3361,.T.) ;
#5241=EDGE_CURVE('',#4105,#4049,#2496,.T.) ;
#5242=EDGE_CURVE('',#4106,#4106,#3362,.T.) ;
#5243=EDGE_CURVE('',#4107,#4108,#303,.T.) ;
#5244=EDGE_CURVE('',#4109,#4107,#3363,.T.) ;
#5245=EDGE_CURVE('',#4110,#4109,#304,.T.) ;
#5246=EDGE_CURVE('',#4111,#4110,#305,.T.) ;
#5247=EDGE_CURVE('',#4112,#4111,#3364,.T.) ;
#5248=EDGE_CURVE('',#4113,#4112,#306,.T.) ;
#5249=EDGE_CURVE('',#4114,#4113,#307,.T.) ;
#5250=EDGE_CURVE('',#4115,#4114,#3365,.T.) ;
#5251=EDGE_CURVE('',#4116,#4115,#308,.T.) ;
#5252=EDGE_CURVE('',#4117,#4116,#309,.T.) ;
#5253=EDGE_CURVE('',#4118,#4117,#3366,.T.) ;
#5254=EDGE_CURVE('',#4119,#4118,#310,.T.) ;
#5255=EDGE_CURVE('',#4120,#4119,#311,.T.) ;
#5256=EDGE_CURVE('',#4121,#4120,#3367,.T.) ;
#5257=EDGE_CURVE('',#4122,#4121,#312,.T.) ;
#5258=EDGE_CURVE('',#4122,#4106,#2497,.T.) ;
#5259=EDGE_CURVE('',#4123,#4122,#313,.T.) ;
#5260=EDGE_CURVE('',#4124,#4123,#3368,.T.) ;
#5261=EDGE_CURVE('',#4108,#4124,#314,.T.) ;
#5262=EDGE_CURVE('',#4118,#4125,#2498,.T.) ;
#5263=EDGE_CURVE('',#4126,#4117,#2499,.T.) ;
#5264=EDGE_CURVE('',#4125,#4126,#3369,.T.) ;
#5265=EDGE_CURVE('',#4127,#4114,#2500,.T.) ;
#5266=EDGE_CURVE('',#4128,#4127,#3370,.T.) ;
#5267=EDGE_CURVE('',#4115,#4128,#2501,.T.) ;
#5268=EDGE_CURVE('',#4121,#4129,#2502,.T.) ;
#5269=EDGE_CURVE('',#4130,#4120,#2503,.T.) ;
#5270=EDGE_CURVE('',#4129,#4130,#3371,.T.) ;
#5271=EDGE_CURVE('',#4131,#4111,#2504,.T.) ;
#5272=EDGE_CURVE('',#4132,#4131,#3372,.T.) ;
#5273=EDGE_CURVE('',#4112,#4132,#2505,.T.) ;
#5274=EDGE_CURVE('',#4124,#4133,#2506,.T.) ;
#5275=EDGE_CURVE('',#4134,#4123,#2507,.T.) ;
#5276=EDGE_CURVE('',#4133,#4134,#3373,.T.) ;
#5277=EDGE_CURVE('',#4135,#4107,#2508,.T.) ;
#5278=EDGE_CURVE('',#4136,#4135,#3374,.T.) ;
#5279=EDGE_CURVE('',#4109,#4136,#2509,.T.) ;
#5280=EDGE_CURVE('',#4134,#4133,#2510,.T.) ;
#5281=EDGE_CURVE('',#4122,#4137,#2511,.T.) ;
#5282=EDGE_CURVE('',#4137,#4138,#2512,.T.) ;
#5283=EDGE_CURVE('',#4108,#4138,#2513,.T.) ;
#5284=EDGE_CURVE('',#4130,#4129,#2514,.T.) ;
#5285=EDGE_CURVE('',#4119,#4139,#2515,.T.) ;
#5286=EDGE_CURVE('',#4139,#4137,#2516,.T.) ;
#5287=EDGE_CURVE('',#4126,#4125,#2517,.T.) ;
#5288=EDGE_CURVE('',#4116,#4140,#2518,.T.) ;
#5289=EDGE_CURVE('',#4140,#4139,#2519,.T.) ;
#5290=EDGE_CURVE('',#4127,#4128,#2520,.T.) ;
#5291=EDGE_CURVE('',#4131,#4132,#2521,.T.) ;
#5292=EDGE_CURVE('',#4135,#4136,#2522,.T.) ;
#5293=EDGE_CURVE('',#4141,#4142,#2523,.T.) ;
#5294=EDGE_CURVE('',#4142,#4141,#3375,.T.) ;
#5295=EDGE_CURVE('',#4142,#4140,#2524,.T.) ;
#5296=EDGE_CURVE('',#4140,#4142,#3376,.T.) ;
#5297=EDGE_CURVE('',#4139,#4140,#3377,.T.) ;
#5298=EDGE_CURVE('',#4137,#4139,#3378,.T.) ;
#5299=EDGE_CURVE('',#4138,#4137,#3379,.T.) ;
#5300=EDGE_CURVE('',#4138,#4141,#2525,.T.) ;
#5301=EDGE_CURVE('',#4141,#4138,#3380,.T.) ;
#5302=EDGE_CURVE('',#4143,#4137,#2526,.T.) ;
#5303=EDGE_CURVE('',#4110,#4141,#2527,.T.) ;
#5304=EDGE_CURVE('',#4113,#4142,#2528,.T.) ;
#6627=ORIENTED_EDGE('',*,*,#4811,.F.) ;
#6628=ORIENTED_EDGE('',*,*,#4812,.T.) ;
#6629=ORIENTED_EDGE('',*,*,#4813,.F.) ;
#6630=ORIENTED_EDGE('',*,*,#4814,.T.) ;
#6631=ORIENTED_EDGE('',*,*,#4815,.F.) ;
#6632=ORIENTED_EDGE('',*,*,#4816,.T.) ;
#6633=ORIENTED_EDGE('',*,*,#4811,.T.) ;
#6634=ORIENTED_EDGE('',*,*,#4817,.T.) ;
#6635=ORIENTED_EDGE('',*,*,#4818,.F.) ;
#6636=ORIENTED_EDGE('',*,*,#4819,.T.) ;
#6637=ORIENTED_EDGE('',*,*,#4815,.T.) ;
#6638=ORIENTED_EDGE('',*,*,#4820,.T.) ;
#6639=ORIENTED_EDGE('',*,*,#4821,.F.) ;
#6640=ORIENTED_EDGE('',*,*,#4822,.T.) ;
#6641=ORIENTED_EDGE('',*,*,#4818,.T.) ;
#6642=ORIENTED_EDGE('',*,*,#4823,.T.) ;
#6643=ORIENTED_EDGE('',*,*,#4824,.F.) ;
#6644=ORIENTED_EDGE('',*,*,#4825,.T.) ;
#6645=ORIENTED_EDGE('',*,*,#4821,.T.) ;
#6646=ORIENTED_EDGE('',*,*,#4826,.T.) ;
#6647=ORIENTED_EDGE('',*,*,#4827,.F.) ;
#6648=ORIENTED_EDGE('',*,*,#4828,.T.) ;
#6649=ORIENTED_EDGE('',*,*,#4824,.T.) ;
#6650=ORIENTED_EDGE('',*,*,#4829,.T.) ;
#6651=ORIENTED_EDGE('',*,*,#4830,.F.) ;
#6652=ORIENTED_EDGE('',*,*,#4831,.T.) ;
#6653=ORIENTED_EDGE('',*,*,#4827,.T.) ;
#6654=ORIENTED_EDGE('',*,*,#4832,.T.) ;
#6655=ORIENTED_EDGE('',*,*,#4833,.F.) ;
#6656=ORIENTED_EDGE('',*,*,#4834,.T.) ;
#6657=ORIENTED_EDGE('',*,*,#4830,.T.) ;
#6658=ORIENTED_EDGE('',*,*,#4835,.T.) ;
#6659=ORIENTED_EDGE('',*,*,#4836,.F.) ;
#6660=ORIENTED_EDGE('',*,*,#4837,.T.) ;
#6661=ORIENTED_EDGE('',*,*,#4833,.T.) ;
#6662=ORIENTED_EDGE('',*,*,#4838,.T.) ;
#6663=ORIENTED_EDGE('',*,*,#4839,.F.) ;
#6664=ORIENTED_EDGE('',*,*,#4840,.T.) ;
#6665=ORIENTED_EDGE('',*,*,#4836,.T.) ;
#6666=ORIENTED_EDGE('',*,*,#4841,.T.) ;
#6667=ORIENTED_EDGE('',*,*,#4842,.F.) ;
#6668=ORIENTED_EDGE('',*,*,#4843,.T.) ;
#6669=ORIENTED_EDGE('',*,*,#4839,.T.) ;
#6670=ORIENTED_EDGE('',*,*,#4844,.T.) ;
#6671=ORIENTED_EDGE('',*,*,#4845,.F.) ;
#6672=ORIENTED_EDGE('',*,*,#4846,.T.) ;
#6673=ORIENTED_EDGE('',*,*,#4842,.T.) ;
#6674=ORIENTED_EDGE('',*,*,#4847,.T.) ;
#6675=ORIENTED_EDGE('',*,*,#4848,.F.) ;
#6676=ORIENTED_EDGE('',*,*,#4849,.T.) ;
#6677=ORIENTED_EDGE('',*,*,#4845,.T.) ;
#6678=ORIENTED_EDGE('',*,*,#4850,.T.) ;
#6679=ORIENTED_EDGE('',*,*,#4851,.F.) ;
#6680=ORIENTED_EDGE('',*,*,#4852,.F.) ;
#6681=ORIENTED_EDGE('',*,*,#4853,.T.) ;
#6682=ORIENTED_EDGE('',*,*,#4848,.T.) ;
#6683=ORIENTED_EDGE('',*,*,#4854,.T.) ;
#6684=ORIENTED_EDGE('',*,*,#4855,.F.) ;
#6685=ORIENTED_EDGE('',*,*,#4856,.T.) ;
#6686=ORIENTED_EDGE('',*,*,#4857,.F.) ;
#6687=ORIENTED_EDGE('',*,*,#4858,.F.) ;
#6688=ORIENTED_EDGE('',*,*,#4859,.F.) ;
#6689=ORIENTED_EDGE('',*,*,#4860,.T.) ;
#6690=ORIENTED_EDGE('',*,*,#4855,.T.) ;
#6691=ORIENTED_EDGE('',*,*,#4861,.F.) ;
#6692=ORIENTED_EDGE('',*,*,#4862,.F.) ;
#6693=ORIENTED_EDGE('',*,*,#4863,.T.) ;
#6694=ORIENTED_EDGE('',*,*,#4859,.T.) ;
#6695=ORIENTED_EDGE('',*,*,#4864,.F.) ;
#6696=ORIENTED_EDGE('',*,*,#4865,.F.) ;
#6697=ORIENTED_EDGE('',*,*,#4866,.T.) ;
#6698=ORIENTED_EDGE('',*,*,#4862,.T.) ;
#6699=ORIENTED_EDGE('',*,*,#4867,.F.) ;
#6700=ORIENTED_EDGE('',*,*,#4868,.F.) ;
#6701=ORIENTED_EDGE('',*,*,#4869,.T.) ;
#6702=ORIENTED_EDGE('',*,*,#4865,.T.) ;
#6703=ORIENTED_EDGE('',*,*,#4870,.F.) ;
#6704=ORIENTED_EDGE('',*,*,#4871,.F.) ;
#6705=ORIENTED_EDGE('',*,*,#4872,.T.) ;
#6706=ORIENTED_EDGE('',*,*,#4868,.T.) ;
#6707=ORIENTED_EDGE('',*,*,#4873,.F.) ;
#6708=ORIENTED_EDGE('',*,*,#4874,.F.) ;
#6709=ORIENTED_EDGE('',*,*,#4875,.T.) ;
#6710=ORIENTED_EDGE('',*,*,#4871,.T.) ;
#6711=ORIENTED_EDGE('',*,*,#4876,.F.) ;
#6712=ORIENTED_EDGE('',*,*,#4877,.F.) ;
#6713=ORIENTED_EDGE('',*,*,#4878,.T.) ;
#6714=ORIENTED_EDGE('',*,*,#4874,.T.) ;
#6715=ORIENTED_EDGE('',*,*,#4879,.F.) ;
#6716=ORIENTED_EDGE('',*,*,#4880,.F.) ;
#6717=ORIENTED_EDGE('',*,*,#4881,.T.) ;
#6718=ORIENTED_EDGE('',*,*,#4877,.T.) ;
#6719=ORIENTED_EDGE('',*,*,#4882,.F.) ;
#6720=ORIENTED_EDGE('',*,*,#4883,.F.) ;
#6721=ORIENTED_EDGE('',*,*,#4884,.T.) ;
#6722=ORIENTED_EDGE('',*,*,#4880,.T.) ;
#6723=ORIENTED_EDGE('',*,*,#4885,.F.) ;
#6724=ORIENTED_EDGE('',*,*,#4886,.F.) ;
#6725=ORIENTED_EDGE('',*,*,#4887,.T.) ;
#6726=ORIENTED_EDGE('',*,*,#4883,.T.) ;
#6727=ORIENTED_EDGE('',*,*,#4888,.F.) ;
#6728=ORIENTED_EDGE('',*,*,#4889,.F.) ;
#6729=ORIENTED_EDGE('',*,*,#4890,.T.) ;
#6730=ORIENTED_EDGE('',*,*,#4886,.T.) ;
#6731=ORIENTED_EDGE('',*,*,#4891,.F.) ;
#6732=ORIENTED_EDGE('',*,*,#4892,.F.) ;
#6733=ORIENTED_EDGE('',*,*,#4893,.T.) ;
#6734=ORIENTED_EDGE('',*,*,#4889,.T.) ;
#6735=ORIENTED_EDGE('',*,*,#4894,.F.) ;
#6736=ORIENTED_EDGE('',*,*,#4857,.T.) ;
#6737=ORIENTED_EDGE('',*,*,#4895,.T.) ;
#6738=ORIENTED_EDGE('',*,*,#4896,.F.) ;
#6739=ORIENTED_EDGE('',*,*,#4897,.T.) ;
#6740=ORIENTED_EDGE('',*,*,#4897,.F.) ;
#6741=ORIENTED_EDGE('',*,*,#4898,.F.) ;
#6742=ORIENTED_EDGE('',*,*,#4854,.F.) ;
#6743=ORIENTED_EDGE('',*,*,#4850,.F.) ;
#6744=ORIENTED_EDGE('',*,*,#4847,.F.) ;
#6745=ORIENTED_EDGE('',*,*,#4844,.F.) ;
#6746=ORIENTED_EDGE('',*,*,#4841,.F.) ;
#6747=ORIENTED_EDGE('',*,*,#4838,.F.) ;
#6748=ORIENTED_EDGE('',*,*,#4835,.F.) ;
#6749=ORIENTED_EDGE('',*,*,#4832,.F.) ;
#6750=ORIENTED_EDGE('',*,*,#4829,.F.) ;
#6751=ORIENTED_EDGE('',*,*,#4826,.F.) ;
#6752=ORIENTED_EDGE('',*,*,#4823,.F.) ;
#6753=ORIENTED_EDGE('',*,*,#4820,.F.) ;
#6754=ORIENTED_EDGE('',*,*,#4817,.F.) ;
#6755=ORIENTED_EDGE('',*,*,#4814,.F.) ;
#6756=ORIENTED_EDGE('',*,*,#4899,.F.) ;
#6757=ORIENTED_EDGE('',*,*,#4900,.T.) ;
#6758=ORIENTED_EDGE('',*,*,#4894,.T.) ;
#6759=ORIENTED_EDGE('',*,*,#4891,.T.) ;
#6760=ORIENTED_EDGE('',*,*,#4888,.T.) ;
#6761=ORIENTED_EDGE('',*,*,#4885,.T.) ;
#6762=ORIENTED_EDGE('',*,*,#4882,.T.) ;
#6763=ORIENTED_EDGE('',*,*,#4879,.T.) ;
#6764=ORIENTED_EDGE('',*,*,#4876,.T.) ;
#6765=ORIENTED_EDGE('',*,*,#4873,.T.) ;
#6766=ORIENTED_EDGE('',*,*,#4870,.T.) ;
#6767=ORIENTED_EDGE('',*,*,#4867,.T.) ;
#6768=ORIENTED_EDGE('',*,*,#4864,.T.) ;
#6769=ORIENTED_EDGE('',*,*,#4861,.T.) ;
#6770=ORIENTED_EDGE('',*,*,#4858,.T.) ;
#6771=ORIENTED_EDGE('',*,*,#4901,.F.) ;
#6772=ORIENTED_EDGE('',*,*,#4902,.T.) ;
#6773=ORIENTED_EDGE('',*,*,#4903,.T.) ;
#6774=ORIENTED_EDGE('',*,*,#4899,.T.) ;
#6775=ORIENTED_EDGE('',*,*,#4904,.F.) ;
#6776=ORIENTED_EDGE('',*,*,#4892,.T.) ;
#6777=ORIENTED_EDGE('',*,*,#4900,.F.) ;
#6778=ORIENTED_EDGE('',*,*,#4903,.F.) ;
#6779=ORIENTED_EDGE('',*,*,#4905,.T.) ;
#6780=ORIENTED_EDGE('',*,*,#4895,.F.) ;
#6781=ORIENTED_EDGE('',*,*,#4856,.F.) ;
#6782=ORIENTED_EDGE('',*,*,#4860,.F.) ;
#6783=ORIENTED_EDGE('',*,*,#4863,.F.) ;
#6784=ORIENTED_EDGE('',*,*,#4866,.F.) ;
#6785=ORIENTED_EDGE('',*,*,#4869,.F.) ;
#6786=ORIENTED_EDGE('',*,*,#4872,.F.) ;
#6787=ORIENTED_EDGE('',*,*,#4875,.F.) ;
#6788=ORIENTED_EDGE('',*,*,#4878,.F.) ;
#6789=ORIENTED_EDGE('',*,*,#4881,.F.) ;
#6790=ORIENTED_EDGE('',*,*,#4884,.F.) ;
#6791=ORIENTED_EDGE('',*,*,#4887,.F.) ;
#6792=ORIENTED_EDGE('',*,*,#4890,.F.) ;
#6793=ORIENTED_EDGE('',*,*,#4893,.F.) ;
#6794=ORIENTED_EDGE('',*,*,#4905,.F.) ;
#6795=ORIENTED_EDGE('',*,*,#4902,.F.) ;
#6796=ORIENTED_EDGE('',*,*,#4812,.F.) ;
#6797=ORIENTED_EDGE('',*,*,#4816,.F.) ;
#6798=ORIENTED_EDGE('',*,*,#4819,.F.) ;
#6799=ORIENTED_EDGE('',*,*,#4822,.F.) ;
#6800=ORIENTED_EDGE('',*,*,#4825,.F.) ;
#6801=ORIENTED_EDGE('',*,*,#4828,.F.) ;
#6802=ORIENTED_EDGE('',*,*,#4831,.F.) ;
#6803=ORIENTED_EDGE('',*,*,#4834,.F.) ;
#6804=ORIENTED_EDGE('',*,*,#4837,.F.) ;
#6805=ORIENTED_EDGE('',*,*,#4840,.F.) ;
#6806=ORIENTED_EDGE('',*,*,#4843,.F.) ;
#6807=ORIENTED_EDGE('',*,*,#4846,.F.) ;
#6808=ORIENTED_EDGE('',*,*,#4849,.F.) ;
#6809=ORIENTED_EDGE('',*,*,#4853,.F.) ;
#6810=ORIENTED_EDGE('',*,*,#4901,.T.) ;
#6811=ORIENTED_EDGE('',*,*,#4906,.T.) ;
#6812=ORIENTED_EDGE('',*,*,#4907,.T.) ;
#6813=ORIENTED_EDGE('',*,*,#4906,.F.) ;
#6814=ORIENTED_EDGE('',*,*,#4904,.T.) ;
#6815=ORIENTED_EDGE('',*,*,#4813,.T.) ;
#6816=ORIENTED_EDGE('',*,*,#4851,.T.) ;
#6817=ORIENTED_EDGE('',*,*,#4898,.T.) ;
#6818=ORIENTED_EDGE('',*,*,#4908,.F.) ;
#6819=ORIENTED_EDGE('',*,*,#4909,.F.) ;
#6820=ORIENTED_EDGE('',*,*,#4907,.F.) ;
#6821=ORIENTED_EDGE('',*,*,#4852,.T.) ;
#6822=ORIENTED_EDGE('',*,*,#4910,.T.) ;
#6823=ORIENTED_EDGE('',*,*,#4911,.T.) ;
#6824=ORIENTED_EDGE('',*,*,#4910,.F.) ;
#6825=ORIENTED_EDGE('',*,*,#4908,.T.) ;
#6826=ORIENTED_EDGE('',*,*,#4896,.T.) ;
#6827=ORIENTED_EDGE('',*,*,#4911,.F.) ;
#6828=ORIENTED_EDGE('',*,*,#4912,.F.) ;
#6829=ORIENTED_EDGE('',*,*,#4913,.T.) ;
#6830=ORIENTED_EDGE('',*,*,#4914,.T.) ;
#6831=ORIENTED_EDGE('',*,*,#4915,.F.) ;
#6832=ORIENTED_EDGE('',*,*,#4916,.F.) ;
#6833=ORIENTED_EDGE('',*,*,#4914,.F.) ;
#6834=ORIENTED_EDGE('',*,*,#4917,.F.) ;
#6835=ORIENTED_EDGE('',*,*,#4918,.F.) ;
#6836=ORIENTED_EDGE('',*,*,#4919,.F.) ;
#6837=ORIENTED_EDGE('',*,*,#4917,.T.) ;
#6838=ORIENTED_EDGE('',*,*,#4913,.F.) ;
#6839=ORIENTED_EDGE('',*,*,#4915,.T.) ;
#6840=ORIENTED_EDGE('',*,*,#4916,.T.) ;
#6841=ORIENTED_EDGE('',*,*,#4919,.T.) ;
#6842=ORIENTED_EDGE('',*,*,#4920,.F.) ;
#6843=ORIENTED_EDGE('',*,*,#4921,.T.) ;
#6844=ORIENTED_EDGE('',*,*,#4922,.T.) ;
#6845=ORIENTED_EDGE('',*,*,#4923,.T.) ;
#6846=ORIENTED_EDGE('',*,*,#4924,.F.) ;
#6847=ORIENTED_EDGE('',*,*,#4925,.T.) ;
#6848=ORIENTED_EDGE('',*,*,#4926,.T.) ;
#6849=ORIENTED_EDGE('',*,*,#4927,.T.) ;
#6850=ORIENTED_EDGE('',*,*,#4928,.F.) ;
#6851=ORIENTED_EDGE('',*,*,#4929,.T.) ;
#6852=ORIENTED_EDGE('',*,*,#4930,.T.) ;
#6853=ORIENTED_EDGE('',*,*,#4931,.T.) ;
#6854=ORIENTED_EDGE('',*,*,#4932,.F.) ;
#6855=ORIENTED_EDGE('',*,*,#4933,.T.) ;
#6856=ORIENTED_EDGE('',*,*,#4934,.T.) ;
#6857=ORIENTED_EDGE('',*,*,#4935,.T.) ;
#6858=ORIENTED_EDGE('',*,*,#4936,.F.) ;
#6859=ORIENTED_EDGE('',*,*,#4937,.T.) ;
#6860=ORIENTED_EDGE('',*,*,#4938,.T.) ;
#6861=ORIENTED_EDGE('',*,*,#4939,.T.) ;
#6862=ORIENTED_EDGE('',*,*,#4940,.F.) ;
#6863=ORIENTED_EDGE('',*,*,#4941,.T.) ;
#6864=ORIENTED_EDGE('',*,*,#4942,.T.) ;
#6865=ORIENTED_EDGE('',*,*,#4943,.T.) ;
#6866=ORIENTED_EDGE('',*,*,#4944,.F.) ;
#6867=ORIENTED_EDGE('',*,*,#4945,.T.) ;
#6868=ORIENTED_EDGE('',*,*,#4946,.T.) ;
#6869=ORIENTED_EDGE('',*,*,#4947,.T.) ;
#6870=ORIENTED_EDGE('',*,*,#4948,.F.) ;
#6871=ORIENTED_EDGE('',*,*,#4949,.T.) ;
#6872=ORIENTED_EDGE('',*,*,#4950,.T.) ;
#6873=ORIENTED_EDGE('',*,*,#4951,.T.) ;
#6874=ORIENTED_EDGE('',*,*,#4952,.F.) ;
#6875=ORIENTED_EDGE('',*,*,#4953,.T.) ;
#6876=ORIENTED_EDGE('',*,*,#4954,.T.) ;
#6877=ORIENTED_EDGE('',*,*,#4955,.T.) ;
#6878=ORIENTED_EDGE('',*,*,#4956,.F.) ;
#6879=ORIENTED_EDGE('',*,*,#4957,.T.) ;
#6880=ORIENTED_EDGE('',*,*,#4958,.T.) ;
#6881=ORIENTED_EDGE('',*,*,#4959,.T.) ;
#6882=ORIENTED_EDGE('',*,*,#4960,.F.) ;
#6883=ORIENTED_EDGE('',*,*,#4961,.T.) ;
#6884=ORIENTED_EDGE('',*,*,#4962,.T.) ;
#6885=ORIENTED_EDGE('',*,*,#4963,.T.) ;
#6886=ORIENTED_EDGE('',*,*,#4964,.F.) ;
#6887=ORIENTED_EDGE('',*,*,#4965,.T.) ;
#6888=ORIENTED_EDGE('',*,*,#4966,.T.) ;
#6889=ORIENTED_EDGE('',*,*,#4967,.T.) ;
#6890=ORIENTED_EDGE('',*,*,#4968,.F.) ;
#6891=ORIENTED_EDGE('',*,*,#4969,.T.) ;
#6892=ORIENTED_EDGE('',*,*,#4970,.T.) ;
#6893=ORIENTED_EDGE('',*,*,#4971,.T.) ;
#6894=ORIENTED_EDGE('',*,*,#4972,.F.) ;
#6895=ORIENTED_EDGE('',*,*,#4973,.T.) ;
#6896=ORIENTED_EDGE('',*,*,#4974,.T.) ;
#6897=ORIENTED_EDGE('',*,*,#4975,.T.) ;
#6898=ORIENTED_EDGE('',*,*,#4976,.F.) ;
#6899=ORIENTED_EDGE('',*,*,#4977,.T.) ;
#6900=ORIENTED_EDGE('',*,*,#4978,.T.) ;
#6901=ORIENTED_EDGE('',*,*,#4979,.T.) ;
#6902=ORIENTED_EDGE('',*,*,#4980,.F.) ;
#6903=ORIENTED_EDGE('',*,*,#4981,.T.) ;
#6904=ORIENTED_EDGE('',*,*,#4982,.T.) ;
#6905=ORIENTED_EDGE('',*,*,#4983,.T.) ;
#6906=ORIENTED_EDGE('',*,*,#4984,.F.) ;
#6907=ORIENTED_EDGE('',*,*,#4985,.T.) ;
#6908=ORIENTED_EDGE('',*,*,#4986,.T.) ;
#6909=ORIENTED_EDGE('',*,*,#4987,.T.) ;
#6910=ORIENTED_EDGE('',*,*,#4988,.F.) ;
#6911=ORIENTED_EDGE('',*,*,#4989,.T.) ;
#6912=ORIENTED_EDGE('',*,*,#4990,.T.) ;
#6913=ORIENTED_EDGE('',*,*,#4991,.T.) ;
#6914=ORIENTED_EDGE('',*,*,#4992,.F.) ;
#6915=ORIENTED_EDGE('',*,*,#4993,.T.) ;
#6916=ORIENTED_EDGE('',*,*,#4994,.T.) ;
#6917=ORIENTED_EDGE('',*,*,#4995,.T.) ;
#6918=ORIENTED_EDGE('',*,*,#4996,.F.) ;
#6919=ORIENTED_EDGE('',*,*,#4997,.T.) ;
#6920=ORIENTED_EDGE('',*,*,#4998,.T.) ;
#6921=ORIENTED_EDGE('',*,*,#4999,.T.) ;
#6922=ORIENTED_EDGE('',*,*,#5000,.F.) ;
#6923=ORIENTED_EDGE('',*,*,#5001,.T.) ;
#6924=ORIENTED_EDGE('',*,*,#5002,.T.) ;
#6925=ORIENTED_EDGE('',*,*,#5003,.T.) ;
#6926=ORIENTED_EDGE('',*,*,#5004,.F.) ;
#6927=ORIENTED_EDGE('',*,*,#5005,.T.) ;
#6928=ORIENTED_EDGE('',*,*,#5006,.T.) ;
#6929=ORIENTED_EDGE('',*,*,#5007,.T.) ;
#6930=ORIENTED_EDGE('',*,*,#5008,.F.) ;
#6931=ORIENTED_EDGE('',*,*,#5009,.T.) ;
#6932=ORIENTED_EDGE('',*,*,#5010,.T.) ;
#6933=ORIENTED_EDGE('',*,*,#5011,.T.) ;
#6934=ORIENTED_EDGE('',*,*,#5012,.F.) ;
#6935=ORIENTED_EDGE('',*,*,#5013,.T.) ;
#6936=ORIENTED_EDGE('',*,*,#5014,.T.) ;
#6937=ORIENTED_EDGE('',*,*,#5015,.T.) ;
#6938=ORIENTED_EDGE('',*,*,#5016,.F.) ;
#6939=ORIENTED_EDGE('',*,*,#5017,.T.) ;
#6940=ORIENTED_EDGE('',*,*,#5018,.T.) ;
#6941=ORIENTED_EDGE('',*,*,#5019,.T.) ;
#6942=ORIENTED_EDGE('',*,*,#5020,.F.) ;
#6943=ORIENTED_EDGE('',*,*,#5021,.T.) ;
#6944=ORIENTED_EDGE('',*,*,#5022,.T.) ;
#6945=ORIENTED_EDGE('',*,*,#5023,.T.) ;
#6946=ORIENTED_EDGE('',*,*,#5024,.F.) ;
#6947=ORIENTED_EDGE('',*,*,#5025,.T.) ;
#6948=ORIENTED_EDGE('',*,*,#5026,.T.) ;
#6949=ORIENTED_EDGE('',*,*,#5027,.T.) ;
#6950=ORIENTED_EDGE('',*,*,#5028,.F.) ;
#6951=ORIENTED_EDGE('',*,*,#5029,.T.) ;
#6952=ORIENTED_EDGE('',*,*,#5030,.T.) ;
#6953=ORIENTED_EDGE('',*,*,#5031,.T.) ;
#6954=ORIENTED_EDGE('',*,*,#5032,.F.) ;
#6955=ORIENTED_EDGE('',*,*,#5031,.F.) ;
#6956=ORIENTED_EDGE('',*,*,#5033,.T.) ;
#6957=ORIENTED_EDGE('',*,*,#5034,.T.) ;
#6958=ORIENTED_EDGE('',*,*,#5035,.F.) ;
#6959=ORIENTED_EDGE('',*,*,#5036,.T.) ;
#6960=ORIENTED_EDGE('',*,*,#5037,.T.) ;
#6961=ORIENTED_EDGE('',*,*,#5038,.T.) ;
#6962=ORIENTED_EDGE('',*,*,#5039,.F.) ;
#6963=ORIENTED_EDGE('',*,*,#5040,.T.) ;
#6964=ORIENTED_EDGE('',*,*,#5041,.T.) ;
#6965=ORIENTED_EDGE('',*,*,#5042,.T.) ;
#6966=ORIENTED_EDGE('',*,*,#5043,.F.) ;
#6967=ORIENTED_EDGE('',*,*,#5044,.T.) ;
#6968=ORIENTED_EDGE('',*,*,#5045,.T.) ;
#6969=ORIENTED_EDGE('',*,*,#5046,.T.) ;
#6970=ORIENTED_EDGE('',*,*,#5047,.F.) ;
#6971=ORIENTED_EDGE('',*,*,#5048,.T.) ;
#6972=ORIENTED_EDGE('',*,*,#5049,.T.) ;
#6973=ORIENTED_EDGE('',*,*,#5050,.T.) ;
#6974=ORIENTED_EDGE('',*,*,#5051,.F.) ;
#6975=ORIENTED_EDGE('',*,*,#5052,.T.) ;
#6976=ORIENTED_EDGE('',*,*,#5053,.T.) ;
#6977=ORIENTED_EDGE('',*,*,#5054,.T.) ;
#6978=ORIENTED_EDGE('',*,*,#5055,.F.) ;
#6979=ORIENTED_EDGE('',*,*,#5056,.T.) ;
#6980=ORIENTED_EDGE('',*,*,#5057,.T.) ;
#6981=ORIENTED_EDGE('',*,*,#5058,.T.) ;
#6982=ORIENTED_EDGE('',*,*,#5059,.F.) ;
#6983=ORIENTED_EDGE('',*,*,#5060,.T.) ;
#6984=ORIENTED_EDGE('',*,*,#5061,.T.) ;
#6985=ORIENTED_EDGE('',*,*,#5062,.T.) ;
#6986=ORIENTED_EDGE('',*,*,#5063,.F.) ;
#6987=ORIENTED_EDGE('',*,*,#5064,.F.) ;
#6988=ORIENTED_EDGE('',*,*,#5065,.T.) ;
#6989=ORIENTED_EDGE('',*,*,#5066,.T.) ;
#6990=ORIENTED_EDGE('',*,*,#5060,.F.) ;
#6991=ORIENTED_EDGE('',*,*,#5061,.F.) ;
#6992=ORIENTED_EDGE('',*,*,#5066,.F.) ;
#6993=ORIENTED_EDGE('',*,*,#5067,.F.) ;
#6994=ORIENTED_EDGE('',*,*,#5068,.F.) ;
#6995=ORIENTED_EDGE('',*,*,#5062,.F.) ;
#6996=ORIENTED_EDGE('',*,*,#5067,.T.) ;
#6997=ORIENTED_EDGE('',*,*,#5065,.F.) ;
#6998=ORIENTED_EDGE('',*,*,#5069,.F.) ;
#6999=ORIENTED_EDGE('',*,*,#5070,.T.) ;
#7000=ORIENTED_EDGE('',*,*,#5071,.T.) ;
#7001=ORIENTED_EDGE('',*,*,#5056,.F.) ;
#7002=ORIENTED_EDGE('',*,*,#5057,.F.) ;
#7003=ORIENTED_EDGE('',*,*,#5071,.F.) ;
#7004=ORIENTED_EDGE('',*,*,#5072,.F.) ;
#7005=ORIENTED_EDGE('',*,*,#5073,.F.) ;
#7006=ORIENTED_EDGE('',*,*,#5058,.F.) ;
#7007=ORIENTED_EDGE('',*,*,#5072,.T.) ;
#7008=ORIENTED_EDGE('',*,*,#5070,.F.) ;
#7009=ORIENTED_EDGE('',*,*,#5074,.F.) ;
#7010=ORIENTED_EDGE('',*,*,#5075,.T.) ;
#7011=ORIENTED_EDGE('',*,*,#5076,.T.) ;
#7012=ORIENTED_EDGE('',*,*,#5052,.F.) ;
#7013=ORIENTED_EDGE('',*,*,#5053,.F.) ;
#7014=ORIENTED_EDGE('',*,*,#5076,.F.) ;
#7015=ORIENTED_EDGE('',*,*,#5077,.F.) ;
#7016=ORIENTED_EDGE('',*,*,#5078,.F.) ;
#7017=ORIENTED_EDGE('',*,*,#5054,.F.) ;
#7018=ORIENTED_EDGE('',*,*,#5077,.T.) ;
#7019=ORIENTED_EDGE('',*,*,#5075,.F.) ;
#7020=ORIENTED_EDGE('',*,*,#5079,.F.) ;
#7021=ORIENTED_EDGE('',*,*,#5080,.T.) ;
#7022=ORIENTED_EDGE('',*,*,#5081,.T.) ;
#7023=ORIENTED_EDGE('',*,*,#5048,.F.) ;
#7024=ORIENTED_EDGE('',*,*,#5049,.F.) ;
#7025=ORIENTED_EDGE('',*,*,#5081,.F.) ;
#7026=ORIENTED_EDGE('',*,*,#5082,.F.) ;
#7027=ORIENTED_EDGE('',*,*,#5083,.F.) ;
#7028=ORIENTED_EDGE('',*,*,#5050,.F.) ;
#7029=ORIENTED_EDGE('',*,*,#5082,.T.) ;
#7030=ORIENTED_EDGE('',*,*,#5080,.F.) ;
#7031=ORIENTED_EDGE('',*,*,#5084,.F.) ;
#7032=ORIENTED_EDGE('',*,*,#5085,.T.) ;
#7033=ORIENTED_EDGE('',*,*,#5086,.T.) ;
#7034=ORIENTED_EDGE('',*,*,#5044,.F.) ;
#7035=ORIENTED_EDGE('',*,*,#5045,.F.) ;
#7036=ORIENTED_EDGE('',*,*,#5086,.F.) ;
#7037=ORIENTED_EDGE('',*,*,#5087,.F.) ;
#7038=ORIENTED_EDGE('',*,*,#5088,.F.) ;
#7039=ORIENTED_EDGE('',*,*,#5046,.F.) ;
#7040=ORIENTED_EDGE('',*,*,#5087,.T.) ;
#7041=ORIENTED_EDGE('',*,*,#5085,.F.) ;
#7042=ORIENTED_EDGE('',*,*,#5089,.F.) ;
#7043=ORIENTED_EDGE('',*,*,#5090,.T.) ;
#7044=ORIENTED_EDGE('',*,*,#5091,.T.) ;
#7045=ORIENTED_EDGE('',*,*,#5040,.F.) ;
#7046=ORIENTED_EDGE('',*,*,#5041,.F.) ;
#7047=ORIENTED_EDGE('',*,*,#5091,.F.) ;
#7048=ORIENTED_EDGE('',*,*,#5092,.F.) ;
#7049=ORIENTED_EDGE('',*,*,#5093,.F.) ;
#7050=ORIENTED_EDGE('',*,*,#5042,.F.) ;
#7051=ORIENTED_EDGE('',*,*,#5092,.T.) ;
#7052=ORIENTED_EDGE('',*,*,#5090,.F.) ;
#7053=ORIENTED_EDGE('',*,*,#5094,.F.) ;
#7054=ORIENTED_EDGE('',*,*,#5095,.T.) ;
#7055=ORIENTED_EDGE('',*,*,#5096,.T.) ;
#7056=ORIENTED_EDGE('',*,*,#5036,.F.) ;
#7057=ORIENTED_EDGE('',*,*,#5037,.F.) ;
#7058=ORIENTED_EDGE('',*,*,#5096,.F.) ;
#7059=ORIENTED_EDGE('',*,*,#5097,.F.) ;
#7060=ORIENTED_EDGE('',*,*,#5098,.F.) ;
#7061=ORIENTED_EDGE('',*,*,#5038,.F.) ;
#7062=ORIENTED_EDGE('',*,*,#5097,.T.) ;
#7063=ORIENTED_EDGE('',*,*,#5095,.F.) ;
#7064=ORIENTED_EDGE('',*,*,#5099,.F.) ;
#7065=ORIENTED_EDGE('',*,*,#5100,.T.) ;
#7066=ORIENTED_EDGE('',*,*,#5101,.T.) ;
#7067=ORIENTED_EDGE('',*,*,#5029,.F.) ;
#7068=ORIENTED_EDGE('',*,*,#5030,.F.) ;
#7069=ORIENTED_EDGE('',*,*,#5101,.F.) ;
#7070=ORIENTED_EDGE('',*,*,#5102,.F.) ;
#7071=ORIENTED_EDGE('',*,*,#5033,.F.) ;
#7072=ORIENTED_EDGE('',*,*,#5103,.F.) ;
#7073=ORIENTED_EDGE('',*,*,#5034,.F.) ;
#7074=ORIENTED_EDGE('',*,*,#5102,.T.) ;
#7075=ORIENTED_EDGE('',*,*,#5100,.F.) ;
#7076=ORIENTED_EDGE('',*,*,#5104,.F.) ;
#7077=ORIENTED_EDGE('',*,*,#5105,.T.) ;
#7078=ORIENTED_EDGE('',*,*,#5106,.T.) ;
#7079=ORIENTED_EDGE('',*,*,#5025,.F.) ;
#7080=ORIENTED_EDGE('',*,*,#5026,.F.) ;
#7081=ORIENTED_EDGE('',*,*,#5106,.F.) ;
#7082=ORIENTED_EDGE('',*,*,#5107,.F.) ;
#7083=ORIENTED_EDGE('',*,*,#5108,.F.) ;
#7084=ORIENTED_EDGE('',*,*,#5027,.F.) ;
#7085=ORIENTED_EDGE('',*,*,#5107,.T.) ;
#7086=ORIENTED_EDGE('',*,*,#5105,.F.) ;
#7087=ORIENTED_EDGE('',*,*,#5109,.F.) ;
#7088=ORIENTED_EDGE('',*,*,#5110,.T.) ;
#7089=ORIENTED_EDGE('',*,*,#5111,.T.) ;
#7090=ORIENTED_EDGE('',*,*,#5021,.F.) ;
#7091=ORIENTED_EDGE('',*,*,#5022,.F.) ;
#7092=ORIENTED_EDGE('',*,*,#5111,.F.) ;
#7093=ORIENTED_EDGE('',*,*,#5112,.F.) ;
#7094=ORIENTED_EDGE('',*,*,#5113,.F.) ;
#7095=ORIENTED_EDGE('',*,*,#5023,.F.) ;
#7096=ORIENTED_EDGE('',*,*,#5112,.T.) ;
#7097=ORIENTED_EDGE('',*,*,#5110,.F.) ;
#7098=ORIENTED_EDGE('',*,*,#5114,.F.) ;
#7099=ORIENTED_EDGE('',*,*,#5115,.T.) ;
#7100=ORIENTED_EDGE('',*,*,#5116,.T.) ;
#7101=ORIENTED_EDGE('',*,*,#5017,.F.) ;
#7102=ORIENTED_EDGE('',*,*,#5018,.F.) ;
#7103=ORIENTED_EDGE('',*,*,#5116,.F.) ;
#7104=ORIENTED_EDGE('',*,*,#5117,.F.) ;
#7105=ORIENTED_EDGE('',*,*,#5118,.F.) ;
#7106=ORIENTED_EDGE('',*,*,#5019,.F.) ;
#7107=ORIENTED_EDGE('',*,*,#5117,.T.) ;
#7108=ORIENTED_EDGE('',*,*,#5115,.F.) ;
#7109=ORIENTED_EDGE('',*,*,#5119,.F.) ;
#7110=ORIENTED_EDGE('',*,*,#5120,.T.) ;
#7111=ORIENTED_EDGE('',*,*,#5121,.T.) ;
#7112=ORIENTED_EDGE('',*,*,#5013,.F.) ;
#7113=ORIENTED_EDGE('',*,*,#5014,.F.) ;
#7114=ORIENTED_EDGE('',*,*,#5121,.F.) ;
#7115=ORIENTED_EDGE('',*,*,#5122,.F.) ;
#7116=ORIENTED_EDGE('',*,*,#5123,.F.) ;
#7117=ORIENTED_EDGE('',*,*,#5015,.F.) ;
#7118=ORIENTED_EDGE('',*,*,#5122,.T.) ;
#7119=ORIENTED_EDGE('',*,*,#5120,.F.) ;
#7120=ORIENTED_EDGE('',*,*,#5124,.F.) ;
#7121=ORIENTED_EDGE('',*,*,#5125,.T.) ;
#7122=ORIENTED_EDGE('',*,*,#5126,.T.) ;
#7123=ORIENTED_EDGE('',*,*,#5009,.F.) ;
#7124=ORIENTED_EDGE('',*,*,#5010,.F.) ;
#7125=ORIENTED_EDGE('',*,*,#5126,.F.) ;
#7126=ORIENTED_EDGE('',*,*,#5127,.F.) ;
#7127=ORIENTED_EDGE('',*,*,#5128,.F.) ;
#7128=ORIENTED_EDGE('',*,*,#5011,.F.) ;
#7129=ORIENTED_EDGE('',*,*,#5127,.T.) ;
#7130=ORIENTED_EDGE('',*,*,#5125,.F.) ;
#7131=ORIENTED_EDGE('',*,*,#5129,.F.) ;
#7132=ORIENTED_EDGE('',*,*,#5130,.T.) ;
#7133=ORIENTED_EDGE('',*,*,#5131,.T.) ;
#7134=ORIENTED_EDGE('',*,*,#5005,.F.) ;
#7135=ORIENTED_EDGE('',*,*,#5006,.F.) ;
#7136=ORIENTED_EDGE('',*,*,#5131,.F.) ;
#7137=ORIENTED_EDGE('',*,*,#5132,.F.) ;
#7138=ORIENTED_EDGE('',*,*,#5133,.F.) ;
#7139=ORIENTED_EDGE('',*,*,#5007,.F.) ;
#7140=ORIENTED_EDGE('',*,*,#5132,.T.) ;
#7141=ORIENTED_EDGE('',*,*,#5130,.F.) ;
#7142=ORIENTED_EDGE('',*,*,#5134,.F.) ;
#7143=ORIENTED_EDGE('',*,*,#5135,.T.) ;
#7144=ORIENTED_EDGE('',*,*,#5136,.T.) ;
#7145=ORIENTED_EDGE('',*,*,#5001,.F.) ;
#7146=ORIENTED_EDGE('',*,*,#5002,.F.) ;
#7147=ORIENTED_EDGE('',*,*,#5136,.F.) ;
#7148=ORIENTED_EDGE('',*,*,#5137,.F.) ;
#7149=ORIENTED_EDGE('',*,*,#5138,.F.) ;
#7150=ORIENTED_EDGE('',*,*,#5003,.F.) ;
#7151=ORIENTED_EDGE('',*,*,#5137,.T.) ;
#7152=ORIENTED_EDGE('',*,*,#5135,.F.) ;
#7153=ORIENTED_EDGE('',*,*,#5139,.F.) ;
#7154=ORIENTED_EDGE('',*,*,#5140,.T.) ;
#7155=ORIENTED_EDGE('',*,*,#5141,.T.) ;
#7156=ORIENTED_EDGE('',*,*,#4997,.F.) ;
#7157=ORIENTED_EDGE('',*,*,#4998,.F.) ;
#7158=ORIENTED_EDGE('',*,*,#5141,.F.) ;
#7159=ORIENTED_EDGE('',*,*,#5142,.F.) ;
#7160=ORIENTED_EDGE('',*,*,#5143,.F.) ;
#7161=ORIENTED_EDGE('',*,*,#4999,.F.) ;
#7162=ORIENTED_EDGE('',*,*,#5142,.T.) ;
#7163=ORIENTED_EDGE('',*,*,#5140,.F.) ;
#7164=ORIENTED_EDGE('',*,*,#5144,.F.) ;
#7165=ORIENTED_EDGE('',*,*,#5145,.T.) ;
#7166=ORIENTED_EDGE('',*,*,#5146,.T.) ;
#7167=ORIENTED_EDGE('',*,*,#4993,.F.) ;
#7168=ORIENTED_EDGE('',*,*,#4994,.F.) ;
#7169=ORIENTED_EDGE('',*,*,#5146,.F.) ;
#7170=ORIENTED_EDGE('',*,*,#5147,.F.) ;
#7171=ORIENTED_EDGE('',*,*,#5148,.F.) ;
#7172=ORIENTED_EDGE('',*,*,#4995,.F.) ;
#7173=ORIENTED_EDGE('',*,*,#5147,.T.) ;
#7174=ORIENTED_EDGE('',*,*,#5145,.F.) ;
#7175=ORIENTED_EDGE('',*,*,#5149,.F.) ;
#7176=ORIENTED_EDGE('',*,*,#5150,.T.) ;
#7177=ORIENTED_EDGE('',*,*,#5151,.T.) ;
#7178=ORIENTED_EDGE('',*,*,#4989,.F.) ;
#7179=ORIENTED_EDGE('',*,*,#4990,.F.) ;
#7180=ORIENTED_EDGE('',*,*,#5151,.F.) ;
#7181=ORIENTED_EDGE('',*,*,#5152,.F.) ;
#7182=ORIENTED_EDGE('',*,*,#5153,.F.) ;
#7183=ORIENTED_EDGE('',*,*,#4991,.F.) ;
#7184=ORIENTED_EDGE('',*,*,#5152,.T.) ;
#7185=ORIENTED_EDGE('',*,*,#5150,.F.) ;
#7186=ORIENTED_EDGE('',*,*,#5154,.F.) ;
#7187=ORIENTED_EDGE('',*,*,#5155,.T.) ;
#7188=ORIENTED_EDGE('',*,*,#5156,.T.) ;
#7189=ORIENTED_EDGE('',*,*,#4985,.F.) ;
#7190=ORIENTED_EDGE('',*,*,#4986,.F.) ;
#7191=ORIENTED_EDGE('',*,*,#5156,.F.) ;
#7192=ORIENTED_EDGE('',*,*,#5157,.F.) ;
#7193=ORIENTED_EDGE('',*,*,#5158,.F.) ;
#7194=ORIENTED_EDGE('',*,*,#4987,.F.) ;
#7195=ORIENTED_EDGE('',*,*,#5157,.T.) ;
#7196=ORIENTED_EDGE('',*,*,#5155,.F.) ;
#7197=ORIENTED_EDGE('',*,*,#5159,.F.) ;
#7198=ORIENTED_EDGE('',*,*,#5160,.T.) ;
#7199=ORIENTED_EDGE('',*,*,#5161,.T.) ;
#7200=ORIENTED_EDGE('',*,*,#4981,.F.) ;
#7201=ORIENTED_EDGE('',*,*,#4982,.F.) ;
#7202=ORIENTED_EDGE('',*,*,#5161,.F.) ;
#7203=ORIENTED_EDGE('',*,*,#5162,.F.) ;
#7204=ORIENTED_EDGE('',*,*,#5163,.F.) ;
#7205=ORIENTED_EDGE('',*,*,#4983,.F.) ;
#7206=ORIENTED_EDGE('',*,*,#5162,.T.) ;
#7207=ORIENTED_EDGE('',*,*,#5160,.F.) ;
#7208=ORIENTED_EDGE('',*,*,#5164,.F.) ;
#7209=ORIENTED_EDGE('',*,*,#5165,.T.) ;
#7210=ORIENTED_EDGE('',*,*,#5166,.T.) ;
#7211=ORIENTED_EDGE('',*,*,#4977,.F.) ;
#7212=ORIENTED_EDGE('',*,*,#4978,.F.) ;
#7213=ORIENTED_EDGE('',*,*,#5166,.F.) ;
#7214=ORIENTED_EDGE('',*,*,#5167,.F.) ;
#7215=ORIENTED_EDGE('',*,*,#5168,.F.) ;
#7216=ORIENTED_EDGE('',*,*,#4979,.F.) ;
#7217=ORIENTED_EDGE('',*,*,#5167,.T.) ;
#7218=ORIENTED_EDGE('',*,*,#5165,.F.) ;
#7219=ORIENTED_EDGE('',*,*,#5169,.F.) ;
#7220=ORIENTED_EDGE('',*,*,#5170,.T.) ;
#7221=ORIENTED_EDGE('',*,*,#5171,.T.) ;
#7222=ORIENTED_EDGE('',*,*,#4973,.F.) ;
#7223=ORIENTED_EDGE('',*,*,#4974,.F.) ;
#7224=ORIENTED_EDGE('',*,*,#5171,.F.) ;
#7225=ORIENTED_EDGE('',*,*,#5172,.F.) ;
#7226=ORIENTED_EDGE('',*,*,#5173,.F.) ;
#7227=ORIENTED_EDGE('',*,*,#4975,.F.) ;
#7228=ORIENTED_EDGE('',*,*,#5172,.T.) ;
#7229=ORIENTED_EDGE('',*,*,#5170,.F.) ;
#7230=ORIENTED_EDGE('',*,*,#5174,.F.) ;
#7231=ORIENTED_EDGE('',*,*,#5175,.T.) ;
#7232=ORIENTED_EDGE('',*,*,#5176,.T.) ;
#7233=ORIENTED_EDGE('',*,*,#4969,.F.) ;
#7234=ORIENTED_EDGE('',*,*,#4970,.F.) ;
#7235=ORIENTED_EDGE('',*,*,#5176,.F.) ;
#7236=ORIENTED_EDGE('',*,*,#5177,.F.) ;
#7237=ORIENTED_EDGE('',*,*,#5178,.F.) ;
#7238=ORIENTED_EDGE('',*,*,#4971,.F.) ;
#7239=ORIENTED_EDGE('',*,*,#5177,.T.) ;
#7240=ORIENTED_EDGE('',*,*,#5175,.F.) ;
#7241=ORIENTED_EDGE('',*,*,#5179,.F.) ;
#7242=ORIENTED_EDGE('',*,*,#5180,.T.) ;
#7243=ORIENTED_EDGE('',*,*,#5181,.T.) ;
#7244=ORIENTED_EDGE('',*,*,#4965,.F.) ;
#7245=ORIENTED_EDGE('',*,*,#4966,.F.) ;
#7246=ORIENTED_EDGE('',*,*,#5181,.F.) ;
#7247=ORIENTED_EDGE('',*,*,#5182,.F.) ;
#7248=ORIENTED_EDGE('',*,*,#5183,.F.) ;
#7249=ORIENTED_EDGE('',*,*,#4967,.F.) ;
#7250=ORIENTED_EDGE('',*,*,#5182,.T.) ;
#7251=ORIENTED_EDGE('',*,*,#5180,.F.) ;
#7252=ORIENTED_EDGE('',*,*,#5184,.F.) ;
#7253=ORIENTED_EDGE('',*,*,#5185,.T.) ;
#7254=ORIENTED_EDGE('',*,*,#5186,.T.) ;
#7255=ORIENTED_EDGE('',*,*,#4961,.F.) ;
#7256=ORIENTED_EDGE('',*,*,#4962,.F.) ;
#7257=ORIENTED_EDGE('',*,*,#5186,.F.) ;
#7258=ORIENTED_EDGE('',*,*,#5187,.F.) ;
#7259=ORIENTED_EDGE('',*,*,#5188,.F.) ;
#7260=ORIENTED_EDGE('',*,*,#4963,.F.) ;
#7261=ORIENTED_EDGE('',*,*,#5187,.T.) ;
#7262=ORIENTED_EDGE('',*,*,#5185,.F.) ;
#7263=ORIENTED_EDGE('',*,*,#5189,.F.) ;
#7264=ORIENTED_EDGE('',*,*,#5190,.T.) ;
#7265=ORIENTED_EDGE('',*,*,#5191,.T.) ;
#7266=ORIENTED_EDGE('',*,*,#4957,.F.) ;
#7267=ORIENTED_EDGE('',*,*,#4958,.F.) ;
#7268=ORIENTED_EDGE('',*,*,#5191,.F.) ;
#7269=ORIENTED_EDGE('',*,*,#5192,.F.) ;
#7270=ORIENTED_EDGE('',*,*,#5193,.F.) ;
#7271=ORIENTED_EDGE('',*,*,#4959,.F.) ;
#7272=ORIENTED_EDGE('',*,*,#5192,.T.) ;
#7273=ORIENTED_EDGE('',*,*,#5190,.F.) ;
#7274=ORIENTED_EDGE('',*,*,#5194,.F.) ;
#7275=ORIENTED_EDGE('',*,*,#5195,.T.) ;
#7276=ORIENTED_EDGE('',*,*,#5196,.T.) ;
#7277=ORIENTED_EDGE('',*,*,#4953,.F.) ;
#7278=ORIENTED_EDGE('',*,*,#4954,.F.) ;
#7279=ORIENTED_EDGE('',*,*,#5196,.F.) ;
#7280=ORIENTED_EDGE('',*,*,#5197,.F.) ;
#7281=ORIENTED_EDGE('',*,*,#5198,.F.) ;
#7282=ORIENTED_EDGE('',*,*,#4955,.F.) ;
#7283=ORIENTED_EDGE('',*,*,#5197,.T.) ;
#7284=ORIENTED_EDGE('',*,*,#5195,.F.) ;
#7285=ORIENTED_EDGE('',*,*,#5199,.F.) ;
#7286=ORIENTED_EDGE('',*,*,#5200,.T.) ;
#7287=ORIENTED_EDGE('',*,*,#5201,.T.) ;
#7288=ORIENTED_EDGE('',*,*,#4949,.F.) ;
#7289=ORIENTED_EDGE('',*,*,#4950,.F.) ;
#7290=ORIENTED_EDGE('',*,*,#5201,.F.) ;
#7291=ORIENTED_EDGE('',*,*,#5202,.F.) ;
#7292=ORIENTED_EDGE('',*,*,#5203,.F.) ;
#7293=ORIENTED_EDGE('',*,*,#4951,.F.) ;
#7294=ORIENTED_EDGE('',*,*,#5202,.T.) ;
#7295=ORIENTED_EDGE('',*,*,#5200,.F.) ;
#7296=ORIENTED_EDGE('',*,*,#5204,.F.) ;
#7297=ORIENTED_EDGE('',*,*,#5205,.T.) ;
#7298=ORIENTED_EDGE('',*,*,#5206,.T.) ;
#7299=ORIENTED_EDGE('',*,*,#4945,.F.) ;
#7300=ORIENTED_EDGE('',*,*,#4946,.F.) ;
#7301=ORIENTED_EDGE('',*,*,#5206,.F.) ;
#7302=ORIENTED_EDGE('',*,*,#5207,.F.) ;
#7303=ORIENTED_EDGE('',*,*,#5208,.F.) ;
#7304=ORIENTED_EDGE('',*,*,#4947,.F.) ;
#7305=ORIENTED_EDGE('',*,*,#5207,.T.) ;
#7306=ORIENTED_EDGE('',*,*,#5205,.F.) ;
#7307=ORIENTED_EDGE('',*,*,#5209,.F.) ;
#7308=ORIENTED_EDGE('',*,*,#5210,.T.) ;
#7309=ORIENTED_EDGE('',*,*,#5211,.T.) ;
#7310=ORIENTED_EDGE('',*,*,#4941,.F.) ;
#7311=ORIENTED_EDGE('',*,*,#4942,.F.) ;
#7312=ORIENTED_EDGE('',*,*,#5211,.F.) ;
#7313=ORIENTED_EDGE('',*,*,#5212,.F.) ;
#7314=ORIENTED_EDGE('',*,*,#5213,.F.) ;
#7315=ORIENTED_EDGE('',*,*,#4943,.F.) ;
#7316=ORIENTED_EDGE('',*,*,#5212,.T.) ;
#7317=ORIENTED_EDGE('',*,*,#5210,.F.) ;
#7318=ORIENTED_EDGE('',*,*,#5214,.F.) ;
#7319=ORIENTED_EDGE('',*,*,#5215,.T.) ;
#7320=ORIENTED_EDGE('',*,*,#5216,.T.) ;
#7321=ORIENTED_EDGE('',*,*,#4937,.F.) ;
#7322=ORIENTED_EDGE('',*,*,#4938,.F.) ;
#7323=ORIENTED_EDGE('',*,*,#5216,.F.) ;
#7324=ORIENTED_EDGE('',*,*,#5217,.F.) ;
#7325=ORIENTED_EDGE('',*,*,#5218,.F.) ;
#7326=ORIENTED_EDGE('',*,*,#4939,.F.) ;
#7327=ORIENTED_EDGE('',*,*,#5217,.T.) ;
#7328=ORIENTED_EDGE('',*,*,#5215,.F.) ;
#7329=ORIENTED_EDGE('',*,*,#5219,.F.) ;
#7330=ORIENTED_EDGE('',*,*,#5220,.T.) ;
#7331=ORIENTED_EDGE('',*,*,#5221,.T.) ;
#7332=ORIENTED_EDGE('',*,*,#4933,.F.) ;
#7333=ORIENTED_EDGE('',*,*,#4934,.F.) ;
#7334=ORIENTED_EDGE('',*,*,#5221,.F.) ;
#7335=ORIENTED_EDGE('',*,*,#5222,.F.) ;
#7336=ORIENTED_EDGE('',*,*,#5223,.F.) ;
#7337=ORIENTED_EDGE('',*,*,#4935,.F.) ;
#7338=ORIENTED_EDGE('',*,*,#5222,.T.) ;
#7339=ORIENTED_EDGE('',*,*,#5220,.F.) ;
#7340=ORIENTED_EDGE('',*,*,#5224,.F.) ;
#7341=ORIENTED_EDGE('',*,*,#5225,.T.) ;
#7342=ORIENTED_EDGE('',*,*,#5226,.T.) ;
#7343=ORIENTED_EDGE('',*,*,#4929,.F.) ;
#7344=ORIENTED_EDGE('',*,*,#4930,.F.) ;
#7345=ORIENTED_EDGE('',*,*,#5226,.F.) ;
#7346=ORIENTED_EDGE('',*,*,#5227,.F.) ;
#7347=ORIENTED_EDGE('',*,*,#5228,.F.) ;
#7348=ORIENTED_EDGE('',*,*,#4931,.F.) ;
#7349=ORIENTED_EDGE('',*,*,#5227,.T.) ;
#7350=ORIENTED_EDGE('',*,*,#5225,.F.) ;
#7351=ORIENTED_EDGE('',*,*,#5229,.F.) ;
#7352=ORIENTED_EDGE('',*,*,#5230,.T.) ;
#7353=ORIENTED_EDGE('',*,*,#5231,.T.) ;
#7354=ORIENTED_EDGE('',*,*,#4925,.F.) ;
#7355=ORIENTED_EDGE('',*,*,#4926,.F.) ;
#7356=ORIENTED_EDGE('',*,*,#5231,.F.) ;
#7357=ORIENTED_EDGE('',*,*,#5232,.F.) ;
#7358=ORIENTED_EDGE('',*,*,#5233,.F.) ;
#7359=ORIENTED_EDGE('',*,*,#4927,.F.) ;
#7360=ORIENTED_EDGE('',*,*,#5232,.T.) ;
#7361=ORIENTED_EDGE('',*,*,#5230,.F.) ;
#7362=ORIENTED_EDGE('',*,*,#5234,.F.) ;
#7363=ORIENTED_EDGE('',*,*,#5235,.T.) ;
#7364=ORIENTED_EDGE('',*,*,#5236,.T.) ;
#7365=ORIENTED_EDGE('',*,*,#4921,.F.) ;
#7366=ORIENTED_EDGE('',*,*,#4922,.F.) ;
#7367=ORIENTED_EDGE('',*,*,#5236,.F.) ;
#7368=ORIENTED_EDGE('',*,*,#5237,.F.) ;
#7369=ORIENTED_EDGE('',*,*,#5238,.F.) ;
#7370=ORIENTED_EDGE('',*,*,#4923,.F.) ;
#7371=ORIENTED_EDGE('',*,*,#5237,.T.) ;
#7372=ORIENTED_EDGE('',*,*,#5235,.F.) ;
#7373=ORIENTED_EDGE('',*,*,#5032,.T.) ;
#7374=ORIENTED_EDGE('',*,*,#5239,.T.) ;
#7375=ORIENTED_EDGE('',*,*,#4909,.T.) ;
#7376=ORIENTED_EDGE('',*,*,#5239,.F.) ;
#7377=ORIENTED_EDGE('',*,*,#5240,.T.) ;
#7378=ORIENTED_EDGE('',*,*,#5241,.T.) ;
#7379=ORIENTED_EDGE('',*,*,#5099,.T.) ;
#7380=ORIENTED_EDGE('',*,*,#5028,.T.) ;
#7381=ORIENTED_EDGE('',*,*,#5108,.T.) ;
#7382=ORIENTED_EDGE('',*,*,#5104,.T.) ;
#7383=ORIENTED_EDGE('',*,*,#5024,.T.) ;
#7384=ORIENTED_EDGE('',*,*,#5113,.T.) ;
#7385=ORIENTED_EDGE('',*,*,#5109,.T.) ;
#7386=ORIENTED_EDGE('',*,*,#5020,.T.) ;
#7387=ORIENTED_EDGE('',*,*,#5118,.T.) ;
#7388=ORIENTED_EDGE('',*,*,#5114,.T.) ;
#7389=ORIENTED_EDGE('',*,*,#5016,.T.) ;
#7390=ORIENTED_EDGE('',*,*,#5123,.T.) ;
#7391=ORIENTED_EDGE('',*,*,#5119,.T.) ;
#7392=ORIENTED_EDGE('',*,*,#5012,.T.) ;
#7393=ORIENTED_EDGE('',*,*,#5128,.T.) ;
#7394=ORIENTED_EDGE('',*,*,#5124,.T.) ;
#7395=ORIENTED_EDGE('',*,*,#5008,.T.) ;
#7396=ORIENTED_EDGE('',*,*,#5133,.T.) ;
#7397=ORIENTED_EDGE('',*,*,#5129,.T.) ;
#7398=ORIENTED_EDGE('',*,*,#5004,.T.) ;
#7399=ORIENTED_EDGE('',*,*,#5138,.T.) ;
#7400=ORIENTED_EDGE('',*,*,#5134,.T.) ;
#7401=ORIENTED_EDGE('',*,*,#5000,.T.) ;
#7402=ORIENTED_EDGE('',*,*,#5143,.T.) ;
#7403=ORIENTED_EDGE('',*,*,#5139,.T.) ;
#7404=ORIENTED_EDGE('',*,*,#4996,.T.) ;
#7405=ORIENTED_EDGE('',*,*,#5148,.T.) ;
#7406=ORIENTED_EDGE('',*,*,#5144,.T.) ;
#7407=ORIENTED_EDGE('',*,*,#4992,.T.) ;
#7408=ORIENTED_EDGE('',*,*,#5153,.T.) ;
#7409=ORIENTED_EDGE('',*,*,#5149,.T.) ;
#7410=ORIENTED_EDGE('',*,*,#4988,.T.) ;
#7411=ORIENTED_EDGE('',*,*,#5158,.T.) ;
#7412=ORIENTED_EDGE('',*,*,#5154,.T.) ;
#7413=ORIENTED_EDGE('',*,*,#4984,.T.) ;
#7414=ORIENTED_EDGE('',*,*,#5163,.T.) ;
#7415=ORIENTED_EDGE('',*,*,#5159,.T.) ;
#7416=ORIENTED_EDGE('',*,*,#4980,.T.) ;
#7417=ORIENTED_EDGE('',*,*,#5168,.T.) ;
#7418=ORIENTED_EDGE('',*,*,#5164,.T.) ;
#7419=ORIENTED_EDGE('',*,*,#4976,.T.) ;
#7420=ORIENTED_EDGE('',*,*,#5173,.T.) ;
#7421=ORIENTED_EDGE('',*,*,#5169,.T.) ;
#7422=ORIENTED_EDGE('',*,*,#4972,.T.) ;
#7423=ORIENTED_EDGE('',*,*,#5178,.T.) ;
#7424=ORIENTED_EDGE('',*,*,#5174,.T.) ;
#7425=ORIENTED_EDGE('',*,*,#4968,.T.) ;
#7426=ORIENTED_EDGE('',*,*,#5183,.T.) ;
#7427=ORIENTED_EDGE('',*,*,#5179,.T.) ;
#7428=ORIENTED_EDGE('',*,*,#4964,.T.) ;
#7429=ORIENTED_EDGE('',*,*,#5188,.T.) ;
#7430=ORIENTED_EDGE('',*,*,#5184,.T.) ;
#7431=ORIENTED_EDGE('',*,*,#4960,.T.) ;
#7432=ORIENTED_EDGE('',*,*,#5193,.T.) ;
#7433=ORIENTED_EDGE('',*,*,#5189,.T.) ;
#7434=ORIENTED_EDGE('',*,*,#4956,.T.) ;
#7435=ORIENTED_EDGE('',*,*,#5198,.T.) ;
#7436=ORIENTED_EDGE('',*,*,#5194,.T.) ;
#7437=ORIENTED_EDGE('',*,*,#4952,.T.) ;
#7438=ORIENTED_EDGE('',*,*,#5203,.T.) ;
#7439=ORIENTED_EDGE('',*,*,#5199,.T.) ;
#7440=ORIENTED_EDGE('',*,*,#4948,.T.) ;
#7441=ORIENTED_EDGE('',*,*,#5208,.T.) ;
#7442=ORIENTED_EDGE('',*,*,#5204,.T.) ;
#7443=ORIENTED_EDGE('',*,*,#4944,.T.) ;
#7444=ORIENTED_EDGE('',*,*,#5213,.T.) ;
#7445=ORIENTED_EDGE('',*,*,#5209,.T.) ;
#7446=ORIENTED_EDGE('',*,*,#4940,.T.) ;
#7447=ORIENTED_EDGE('',*,*,#5218,.T.) ;
#7448=ORIENTED_EDGE('',*,*,#5214,.T.) ;
#7449=ORIENTED_EDGE('',*,*,#4936,.T.) ;
#7450=ORIENTED_EDGE('',*,*,#5223,.T.) ;
#7451=ORIENTED_EDGE('',*,*,#5219,.T.) ;
#7452=ORIENTED_EDGE('',*,*,#4932,.T.) ;
#7453=ORIENTED_EDGE('',*,*,#5228,.T.) ;
#7454=ORIENTED_EDGE('',*,*,#5224,.T.) ;
#7455=ORIENTED_EDGE('',*,*,#4928,.T.) ;
#7456=ORIENTED_EDGE('',*,*,#5233,.T.) ;
#7457=ORIENTED_EDGE('',*,*,#5229,.T.) ;
#7458=ORIENTED_EDGE('',*,*,#4924,.T.) ;
#7459=ORIENTED_EDGE('',*,*,#5238,.T.) ;
#7460=ORIENTED_EDGE('',*,*,#5234,.T.) ;
#7461=ORIENTED_EDGE('',*,*,#4920,.T.) ;
#7462=ORIENTED_EDGE('',*,*,#4918,.T.) ;
#7463=ORIENTED_EDGE('',*,*,#4912,.T.) ;
#7464=ORIENTED_EDGE('',*,*,#5063,.T.) ;
#7465=ORIENTED_EDGE('',*,*,#5068,.T.) ;
#7466=ORIENTED_EDGE('',*,*,#5064,.T.) ;
#7467=ORIENTED_EDGE('',*,*,#5059,.T.) ;
#7468=ORIENTED_EDGE('',*,*,#5073,.T.) ;
#7469=ORIENTED_EDGE('',*,*,#5069,.T.) ;
#7470=ORIENTED_EDGE('',*,*,#5055,.T.) ;
#7471=ORIENTED_EDGE('',*,*,#5078,.T.) ;
#7472=ORIENTED_EDGE('',*,*,#5074,.T.) ;
#7473=ORIENTED_EDGE('',*,*,#5051,.T.) ;
#7474=ORIENTED_EDGE('',*,*,#5083,.T.) ;
#7475=ORIENTED_EDGE('',*,*,#5079,.T.) ;
#7476=ORIENTED_EDGE('',*,*,#5047,.T.) ;
#7477=ORIENTED_EDGE('',*,*,#5088,.T.) ;
#7478=ORIENTED_EDGE('',*,*,#5084,.T.) ;
#7479=ORIENTED_EDGE('',*,*,#5043,.T.) ;
#7480=ORIENTED_EDGE('',*,*,#5093,.T.) ;
#7481=ORIENTED_EDGE('',*,*,#5089,.T.) ;
#7482=ORIENTED_EDGE('',*,*,#5039,.T.) ;
#7483=ORIENTED_EDGE('',*,*,#5098,.T.) ;
#7484=ORIENTED_EDGE('',*,*,#5094,.T.) ;
#7485=ORIENTED_EDGE('',*,*,#5035,.T.) ;
#7486=ORIENTED_EDGE('',*,*,#5103,.T.) ;
#7487=ORIENTED_EDGE('',*,*,#5241,.F.) ;
#7488=ORIENTED_EDGE('',*,*,#5240,.F.) ;
#7489=ORIENTED_EDGE('',*,*,#5242,.T.) ;
#7490=ORIENTED_EDGE('',*,*,#5243,.F.) ;
#7491=ORIENTED_EDGE('',*,*,#5244,.F.) ;
#7492=ORIENTED_EDGE('',*,*,#5245,.F.) ;
#7493=ORIENTED_EDGE('',*,*,#5246,.F.) ;
#7494=ORIENTED_EDGE('',*,*,#5247,.F.) ;
#7495=ORIENTED_EDGE('',*,*,#5248,.F.) ;
#7496=ORIENTED_EDGE('',*,*,#5249,.F.) ;
#7497=ORIENTED_EDGE('',*,*,#5250,.F.) ;
#7498=ORIENTED_EDGE('',*,*,#5251,.F.) ;
#7499=ORIENTED_EDGE('',*,*,#5252,.F.) ;
#7500=ORIENTED_EDGE('',*,*,#5253,.F.) ;
#7501=ORIENTED_EDGE('',*,*,#5254,.F.) ;
#7502=ORIENTED_EDGE('',*,*,#5255,.F.) ;
#7503=ORIENTED_EDGE('',*,*,#5256,.F.) ;
#7504=ORIENTED_EDGE('',*,*,#5257,.F.) ;
#7505=ORIENTED_EDGE('',*,*,#5258,.T.) ;
#7506=ORIENTED_EDGE('',*,*,#5242,.F.) ;
#7507=ORIENTED_EDGE('',*,*,#5258,.F.) ;
#7508=ORIENTED_EDGE('',*,*,#5259,.F.) ;
#7509=ORIENTED_EDGE('',*,*,#5260,.F.) ;
#7510=ORIENTED_EDGE('',*,*,#5261,.F.) ;
#7511=ORIENTED_EDGE('',*,*,#5262,.F.) ;
#7512=ORIENTED_EDGE('',*,*,#5253,.T.) ;
#7513=ORIENTED_EDGE('',*,*,#5263,.F.) ;
#7514=ORIENTED_EDGE('',*,*,#5264,.F.) ;
#7515=ORIENTED_EDGE('',*,*,#5265,.F.) ;
#7516=ORIENTED_EDGE('',*,*,#5266,.F.) ;
#7517=ORIENTED_EDGE('',*,*,#5267,.F.) ;
#7518=ORIENTED_EDGE('',*,*,#5250,.T.) ;
#7519=ORIENTED_EDGE('',*,*,#5268,.F.) ;
#7520=ORIENTED_EDGE('',*,*,#5256,.T.) ;
#7521=ORIENTED_EDGE('',*,*,#5269,.F.) ;
#7522=ORIENTED_EDGE('',*,*,#5270,.F.) ;
#7523=ORIENTED_EDGE('',*,*,#5271,.F.) ;
#7524=ORIENTED_EDGE('',*,*,#5272,.F.) ;
#7525=ORIENTED_EDGE('',*,*,#5273,.F.) ;
#7526=ORIENTED_EDGE('',*,*,#5247,.T.) ;
#7527=ORIENTED_EDGE('',*,*,#5274,.F.) ;
#7528=ORIENTED_EDGE('',*,*,#5260,.T.) ;
#7529=ORIENTED_EDGE('',*,*,#5275,.F.) ;
#7530=ORIENTED_EDGE('',*,*,#5276,.F.) ;
#7531=ORIENTED_EDGE('',*,*,#5277,.F.) ;
#7532=ORIENTED_EDGE('',*,*,#5278,.F.) ;
#7533=ORIENTED_EDGE('',*,*,#5279,.F.) ;
#7534=ORIENTED_EDGE('',*,*,#5244,.T.) ;
#7535=ORIENTED_EDGE('',*,*,#5261,.T.) ;
#7536=ORIENTED_EDGE('',*,*,#5274,.T.) ;
#7537=ORIENTED_EDGE('',*,*,#5280,.F.) ;
#7538=ORIENTED_EDGE('',*,*,#5275,.T.) ;
#7539=ORIENTED_EDGE('',*,*,#5259,.T.) ;
#7540=ORIENTED_EDGE('',*,*,#5281,.T.) ;
#7541=ORIENTED_EDGE('',*,*,#5282,.T.) ;
#7542=ORIENTED_EDGE('',*,*,#5283,.F.) ;
#7543=ORIENTED_EDGE('',*,*,#5257,.T.) ;
#7544=ORIENTED_EDGE('',*,*,#5268,.T.) ;
#7545=ORIENTED_EDGE('',*,*,#5284,.F.) ;
#7546=ORIENTED_EDGE('',*,*,#5269,.T.) ;
#7547=ORIENTED_EDGE('',*,*,#5255,.T.) ;
#7548=ORIENTED_EDGE('',*,*,#5285,.T.) ;
#7549=ORIENTED_EDGE('',*,*,#5286,.T.) ;
#7550=ORIENTED_EDGE('',*,*,#5281,.F.) ;
#7551=ORIENTED_EDGE('',*,*,#5254,.T.) ;
#7552=ORIENTED_EDGE('',*,*,#5262,.T.) ;
#7553=ORIENTED_EDGE('',*,*,#5287,.F.) ;
#7554=ORIENTED_EDGE('',*,*,#5263,.T.) ;
#7555=ORIENTED_EDGE('',*,*,#5252,.T.) ;
#7556=ORIENTED_EDGE('',*,*,#5288,.T.) ;
#7557=ORIENTED_EDGE('',*,*,#5289,.T.) ;
#7558=ORIENTED_EDGE('',*,*,#5285,.F.) ;
#7559=ORIENTED_EDGE('',*,*,#5264,.T.) ;
#7560=ORIENTED_EDGE('',*,*,#5287,.T.) ;
#7561=ORIENTED_EDGE('',*,*,#5270,.T.) ;
#7562=ORIENTED_EDGE('',*,*,#5284,.T.) ;
#7563=ORIENTED_EDGE('',*,*,#5266,.T.) ;
#7564=ORIENTED_EDGE('',*,*,#5290,.T.) ;
#7565=ORIENTED_EDGE('',*,*,#5276,.T.) ;
#7566=ORIENTED_EDGE('',*,*,#5280,.T.) ;
#7567=ORIENTED_EDGE('',*,*,#5272,.T.) ;
#7568=ORIENTED_EDGE('',*,*,#5291,.T.) ;
#7569=ORIENTED_EDGE('',*,*,#5278,.T.) ;
#7570=ORIENTED_EDGE('',*,*,#5292,.T.) ;
#7571=ORIENTED_EDGE('',*,*,#5293,.F.) ;
#7572=ORIENTED_EDGE('',*,*,#5294,.F.) ;
#7573=ORIENTED_EDGE('',*,*,#5295,.F.) ;
#7574=ORIENTED_EDGE('',*,*,#5296,.F.) ;
#7575=ORIENTED_EDGE('',*,*,#5289,.F.) ;
#7576=ORIENTED_EDGE('',*,*,#5297,.F.) ;
#7577=ORIENTED_EDGE('',*,*,#5286,.F.) ;
#7578=ORIENTED_EDGE('',*,*,#5298,.F.) ;
#7579=ORIENTED_EDGE('',*,*,#5282,.F.) ;
#7580=ORIENTED_EDGE('',*,*,#5299,.F.) ;
#7581=ORIENTED_EDGE('',*,*,#5300,.F.) ;
#7582=ORIENTED_EDGE('',*,*,#5301,.F.) ;
#7583=ORIENTED_EDGE('',*,*,#5302,.T.) ;
#7584=ORIENTED_EDGE('',*,*,#5298,.T.) ;
#7585=ORIENTED_EDGE('',*,*,#5297,.T.) ;
#7586=ORIENTED_EDGE('',*,*,#5296,.T.) ;
#7587=ORIENTED_EDGE('',*,*,#5294,.T.) ;
#7588=ORIENTED_EDGE('',*,*,#5301,.T.) ;
#7589=ORIENTED_EDGE('',*,*,#5299,.T.) ;
#7590=ORIENTED_EDGE('',*,*,#5302,.F.) ;
#7591=ORIENTED_EDGE('',*,*,#5246,.T.) ;
#7592=ORIENTED_EDGE('',*,*,#5303,.T.) ;
#7593=ORIENTED_EDGE('',*,*,#5293,.T.) ;
#7594=ORIENTED_EDGE('',*,*,#5304,.F.) ;
#7595=ORIENTED_EDGE('',*,*,#5248,.T.) ;
#7596=ORIENTED_EDGE('',*,*,#5273,.T.) ;
#7597=ORIENTED_EDGE('',*,*,#5291,.F.) ;
#7598=ORIENTED_EDGE('',*,*,#5271,.T.) ;
#7599=ORIENTED_EDGE('',*,*,#5243,.T.) ;
#7600=ORIENTED_EDGE('',*,*,#5283,.T.) ;
#7601=ORIENTED_EDGE('',*,*,#5300,.T.) ;
#7602=ORIENTED_EDGE('',*,*,#5303,.F.) ;
#7603=ORIENTED_EDGE('',*,*,#5245,.T.) ;
#7604=ORIENTED_EDGE('',*,*,#5279,.T.) ;
#7605=ORIENTED_EDGE('',*,*,#5292,.F.) ;
#7606=ORIENTED_EDGE('',*,*,#5277,.T.) ;
#7607=ORIENTED_EDGE('',*,*,#5249,.T.) ;
#7608=ORIENTED_EDGE('',*,*,#5304,.T.) ;
#7609=ORIENTED_EDGE('',*,*,#5295,.T.) ;
#7610=ORIENTED_EDGE('',*,*,#5288,.F.) ;
#7611=ORIENTED_EDGE('',*,*,#5251,.T.) ;
#7612=ORIENTED_EDGE('',*,*,#5267,.T.) ;
#7613=ORIENTED_EDGE('',*,*,#5290,.F.) ;
#7614=ORIENTED_EDGE('',*,*,#5265,.T.) ;
#7728=CONICAL_SURFACE('',#8641,1.704,0.785398163397448) ;
#7729=CONICAL_SURFACE('',#8829,3.3,0.785398163397448) ;
#7730=CONICAL_SURFACE('',#8833,1.83205080756888,0.785398163397456) ;
#7731=CONICAL_SURFACE('',#8873,0.866025403784438,1.02974425867665) ;
#7982=ADVANCED_FACE('',(#1307),#1018,.T.) ;
#7983=ADVANCED_FACE('',(#1308),#1019,.T.) ;
#7984=ADVANCED_FACE('',(#1309),#1020,.T.) ;
#7985=ADVANCED_FACE('',(#1310),#1021,.T.) ;
#7986=ADVANCED_FACE('',(#1311),#1022,.T.) ;
#7987=ADVANCED_FACE('',(#1312),#1023,.T.) ;
#7988=ADVANCED_FACE('',(#1313),#1024,.T.) ;
#7989=ADVANCED_FACE('',(#1314),#1025,.T.) ;
#7990=ADVANCED_FACE('',(#1315),#1026,.T.) ;
#7991=ADVANCED_FACE('',(#1316),#1027,.T.) ;
#7992=ADVANCED_FACE('',(#1317),#1028,.T.) ;
#7993=ADVANCED_FACE('',(#1318),#1029,.T.) ;
#7994=ADVANCED_FACE('',(#1319),#1030,.T.) ;
#7995=ADVANCED_FACE('',(#1320),#1031,.T.) ;
#7996=ADVANCED_FACE('',(#1321),#1032,.T.) ;
#7997=ADVANCED_FACE('',(#1322),#1033,.T.) ;
#7998=ADVANCED_FACE('',(#1323),#1034,.T.) ;
#7999=ADVANCED_FACE('',(#1324),#1035,.T.) ;
#8000=ADVANCED_FACE('',(#1325),#1036,.T.) ;
#8001=ADVANCED_FACE('',(#1326),#1037,.T.) ;
#8002=ADVANCED_FACE('',(#1327),#1038,.T.) ;
#8003=ADVANCED_FACE('',(#1328),#1039,.T.) ;
#8004=ADVANCED_FACE('',(#1329),#1040,.T.) ;
#8005=ADVANCED_FACE('',(#1330),#1041,.T.) ;
#8006=ADVANCED_FACE('',(#1331),#1042,.T.) ;
#8007=ADVANCED_FACE('',(#1332),#1043,.T.) ;
#8008=ADVANCED_FACE('',(#1333),#1044,.T.) ;
#8009=ADVANCED_FACE('',(#1334),#836,.T.) ;
#8010=ADVANCED_FACE('',(#1335),#413,.F.) ;
#8011=ADVANCED_FACE('',(#1336),#837,.F.) ;
#8012=ADVANCED_FACE('',(#1337),#1045,.T.) ;
#8013=ADVANCED_FACE('',(#1338),#414,.F.) ;
#8014=ADVANCED_FACE('',(#1339),#317,.F.) ;
#8015=ADVANCED_FACE('',(#1340),#1046,.T.) ;
#8016=ADVANCED_FACE('',(#1341,#729),#838,.F.) ;
#8017=ADVANCED_FACE('',(#1342),#7728,.T.) ;
#8018=ADVANCED_FACE('',(#1343),#839,.F.) ;
#8019=ADVANCED_FACE('',(#1344),#840,.F.) ;
#8020=ADVANCED_FACE('',(#1345),#841,.F.) ;
#8021=ADVANCED_FACE('',(#1346),#842,.F.) ;
#8022=ADVANCED_FACE('',(#1347),#1047,.T.) ;
#8023=ADVANCED_FACE('',(#1348),#843,.F.) ;
#8024=ADVANCED_FACE('',(#1349),#844,.F.) ;
#8025=ADVANCED_FACE('',(#1350),#845,.F.) ;
#8026=ADVANCED_FACE('',(#1351),#846,.F.) ;
#8027=ADVANCED_FACE('',(#1352),#847,.F.) ;
#8028=ADVANCED_FACE('',(#1353),#848,.F.) ;
#8029=ADVANCED_FACE('',(#1354),#849,.F.) ;
#8030=ADVANCED_FACE('',(#1355),#850,.F.) ;
#8031=ADVANCED_FACE('',(#1356),#851,.F.) ;
#8032=ADVANCED_FACE('',(#1357),#852,.F.) ;
#8033=ADVANCED_FACE('',(#1358),#853,.F.) ;
#8034=ADVANCED_FACE('',(#1359),#854,.F.) ;
#8035=ADVANCED_FACE('',(#1360),#855,.F.) ;
#8036=ADVANCED_FACE('',(#1361),#856,.F.) ;
#8037=ADVANCED_FACE('',(#1362),#857,.F.) ;
#8038=ADVANCED_FACE('',(#1363),#858,.F.) ;
#8039=ADVANCED_FACE('',(#1364),#859,.F.) ;
#8040=ADVANCED_FACE('',(#1365),#860,.F.) ;
#8041=ADVANCED_FACE('',(#1366),#861,.F.) ;
#8042=ADVANCED_FACE('',(#1367),#862,.F.) ;
#8043=ADVANCED_FACE('',(#1368),#863,.F.) ;
#8044=ADVANCED_FACE('',(#1369),#864,.F.) ;
#8045=ADVANCED_FACE('',(#1370),#865,.F.) ;
#8046=ADVANCED_FACE('',(#1371),#866,.F.) ;
#8047=ADVANCED_FACE('',(#1372),#867,.F.) ;
#8048=ADVANCED_FACE('',(#1373),#868,.F.) ;
#8049=ADVANCED_FACE('',(#1374),#869,.F.) ;
#8050=ADVANCED_FACE('',(#1375),#870,.F.) ;
#8051=ADVANCED_FACE('',(#1376),#871,.F.) ;
#8052=ADVANCED_FACE('',(#1377),#872,.F.) ;
#8053=ADVANCED_FACE('',(#1378),#873,.F.) ;
#8054=ADVANCED_FACE('',(#1379),#874,.F.) ;
#8055=ADVANCED_FACE('',(#1380),#875,.F.) ;
#8056=ADVANCED_FACE('',(#1381),#876,.F.) ;
#8057=ADVANCED_FACE('',(#1382),#877,.F.) ;
#8058=ADVANCED_FACE('',(#1383),#878,.F.) ;
#8059=ADVANCED_FACE('',(#1384),#879,.F.) ;
#8060=ADVANCED_FACE('',(#1385),#880,.F.) ;
#8061=ADVANCED_FACE('',(#1386),#881,.F.) ;
#8062=ADVANCED_FACE('',(#1387),#882,.F.) ;
#8063=ADVANCED_FACE('',(#1388),#883,.F.) ;
#8064=ADVANCED_FACE('',(#1389),#884,.F.) ;
#8065=ADVANCED_FACE('',(#1390),#885,.F.) ;
#8066=ADVANCED_FACE('',(#1391),#886,.F.) ;
#8067=ADVANCED_FACE('',(#1392),#887,.F.) ;
#8068=ADVANCED_FACE('',(#1393),#888,.F.) ;
#8069=ADVANCED_FACE('',(#1394),#889,.F.) ;
#8070=ADVANCED_FACE('',(#1395),#890,.F.) ;
#8071=ADVANCED_FACE('',(#1396),#891,.F.) ;
#8072=ADVANCED_FACE('',(#1397),#892,.F.) ;
#8073=ADVANCED_FACE('',(#1398),#893,.F.) ;
#8074=ADVANCED_FACE('',(#1399),#894,.F.) ;
#8075=ADVANCED_FACE('',(#1400),#895,.F.) ;
#8076=ADVANCED_FACE('',(#1401),#896,.F.) ;
#8077=ADVANCED_FACE('',(#1402),#897,.F.) ;
#8078=ADVANCED_FACE('',(#1403),#898,.F.) ;
#8079=ADVANCED_FACE('',(#1404),#899,.F.) ;
#8080=ADVANCED_FACE('',(#1405),#900,.F.) ;
#8081=ADVANCED_FACE('',(#1406),#901,.F.) ;
#8082=ADVANCED_FACE('',(#1407),#902,.F.) ;
#8083=ADVANCED_FACE('',(#1408),#903,.F.) ;
#8084=ADVANCED_FACE('',(#1409),#904,.F.) ;
#8085=ADVANCED_FACE('',(#1410),#905,.F.) ;
#8086=ADVANCED_FACE('',(#1411),#906,.F.) ;
#8087=ADVANCED_FACE('',(#1412),#907,.F.) ;
#8088=ADVANCED_FACE('',(#1413),#908,.F.) ;
#8089=ADVANCED_FACE('',(#1414),#909,.F.) ;
#8090=ADVANCED_FACE('',(#1415),#910,.F.) ;
#8091=ADVANCED_FACE('',(#1416),#911,.F.) ;
#8092=ADVANCED_FACE('',(#1417),#912,.F.) ;
#8093=ADVANCED_FACE('',(#1418),#913,.F.) ;
#8094=ADVANCED_FACE('',(#1419),#914,.F.) ;
#8095=ADVANCED_FACE('',(#1420),#915,.F.) ;
#8096=ADVANCED_FACE('',(#1421),#916,.F.) ;
#8097=ADVANCED_FACE('',(#1422),#917,.F.) ;
#8098=ADVANCED_FACE('',(#1423),#918,.F.) ;
#8099=ADVANCED_FACE('',(#1424),#919,.F.) ;
#8100=ADVANCED_FACE('',(#1425),#920,.F.) ;
#8101=ADVANCED_FACE('',(#1426),#921,.F.) ;
#8102=ADVANCED_FACE('',(#1427),#922,.F.) ;
#8103=ADVANCED_FACE('',(#1428),#923,.F.) ;
#8104=ADVANCED_FACE('',(#1429),#924,.F.) ;
#8105=ADVANCED_FACE('',(#1430),#925,.F.) ;
#8106=ADVANCED_FACE('',(#1431),#926,.F.) ;
#8107=ADVANCED_FACE('',(#1432),#927,.F.) ;
#8108=ADVANCED_FACE('',(#1433),#928,.F.) ;
#8109=ADVANCED_FACE('',(#1434),#929,.F.) ;
#8110=ADVANCED_FACE('',(#1435),#930,.F.) ;
#8111=ADVANCED_FACE('',(#1436),#931,.F.) ;
#8112=ADVANCED_FACE('',(#1437),#932,.F.) ;
#8113=ADVANCED_FACE('',(#1438),#933,.F.) ;
#8114=ADVANCED_FACE('',(#1439),#934,.F.) ;
#8115=ADVANCED_FACE('',(#1440),#935,.F.) ;
#8116=ADVANCED_FACE('',(#1441),#936,.F.) ;
#8117=ADVANCED_FACE('',(#1442),#937,.F.) ;
#8118=ADVANCED_FACE('',(#1443),#938,.F.) ;
#8119=ADVANCED_FACE('',(#1444),#939,.F.) ;
#8120=ADVANCED_FACE('',(#1445),#940,.F.) ;
#8121=ADVANCED_FACE('',(#1446),#941,.F.) ;
#8122=ADVANCED_FACE('',(#1447),#942,.F.) ;
#8123=ADVANCED_FACE('',(#1448),#943,.F.) ;
#8124=ADVANCED_FACE('',(#1449),#944,.F.) ;
#8125=ADVANCED_FACE('',(#1450),#945,.F.) ;
#8126=ADVANCED_FACE('',(#1451),#946,.F.) ;
#8127=ADVANCED_FACE('',(#1452),#947,.F.) ;
#8128=ADVANCED_FACE('',(#1453),#318,.T.) ;
#8129=ADVANCED_FACE('',(#1454),#7729,.T.) ;
#8130=ADVANCED_FACE('',(#1455,#730),#948,.T.) ;
#8131=ADVANCED_FACE('',(#1456),#7730,.F.) ;
#8132=ADVANCED_FACE('',(#1457),#1048,.T.) ;
#8133=ADVANCED_FACE('',(#1458),#1049,.T.) ;
#8134=ADVANCED_FACE('',(#1459),#1050,.T.) ;
#8135=ADVANCED_FACE('',(#1460),#1051,.T.) ;
#8136=ADVANCED_FACE('',(#1461),#1052,.T.) ;
#8137=ADVANCED_FACE('',(#1462),#1053,.T.) ;
#8138=ADVANCED_FACE('',(#1463),#949,.F.) ;
#8139=ADVANCED_FACE('',(#1464),#950,.F.) ;
#8140=ADVANCED_FACE('',(#1465),#951,.F.) ;
#8141=ADVANCED_FACE('',(#1466),#952,.T.) ;
#8142=ADVANCED_FACE('',(#1467),#953,.T.) ;
#8143=ADVANCED_FACE('',(#1468),#954,.T.) ;
#8144=ADVANCED_FACE('',(#1469),#955,.T.) ;
#8145=ADVANCED_FACE('',(#1470),#956,.T.) ;
#8146=ADVANCED_FACE('',(#1471),#957,.T.) ;
#8147=ADVANCED_FACE('',(#1472),#958,.F.) ;
#8148=ADVANCED_FACE('',(#1473),#959,.F.) ;
#8149=ADVANCED_FACE('',(#1474),#960,.F.) ;
#8150=ADVANCED_FACE('',(#1475),#961,.F.) ;
#8151=ADVANCED_FACE('',(#1476),#962,.F.) ;
#8152=ADVANCED_FACE('',(#1477),#963,.F.) ;
#8153=ADVANCED_FACE('',(#1478),#7731,.F.) ;
#8154=ADVANCED_FACE('',(#1479),#964,.F.) ;
#8155=ADVANCED_FACE('',(#1480),#965,.F.) ;
#8156=ADVANCED_FACE('',(#1481),#966,.F.) ;
#8182=CLOSED_SHELL('',(#7982,#7983,#7984,#7985,#7986,#7987,#7988,#7989,
#7990,#7991,#7992,#7993,#7994,#7995,#7996,#7997,#7998,#7999,#8000,#8001,
#8002,#8003,#8004,#8005,#8006,#8007,#8008,#8009,#8010,#8011,#8012,#8013,
#8014,#8015,#8016,#8017,#8018,#8019,#8020,#8021,#8022,#8023,#8024,#8025,
#8026,#8027,#8028,#8029,#8030,#8031,#8032,#8033,#8034,#8035,#8036,#8037,
#8038,#8039,#8040,#8041,#8042,#8043,#8044,#8045,#8046,#8047,#8048,#8049,
#8050,#8051,#8052,#8053,#8054,#8055,#8056,#8057,#8058,#8059,#8060,#8061,
#8062,#8063,#8064,#8065,#8066,#8067,#8068,#8069,#8070,#8071,#8072,#8073,
#8074,#8075,#8076,#8077,#8078,#8079,#8080,#8081,#8082,#8083,#8084,#8085,
#8086,#8087,#8088,#8089,#8090,#8091,#8092,#8093,#8094,#8095,#8096,#8097,
#8098,#8099,#8100,#8101,#8102,#8103,#8104,#8105,#8106,#8107,#8108,#8109,
#8110,#8111,#8112,#8113,#8114,#8115,#8116,#8117,#8118,#8119,#8120,#8121,
#8122,#8123,#8124,#8125,#8126,#8127,#8128,#8129,#8130,#8131,#8132,#8133,
#8134,#8135,#8136,#8137,#8138,#8139,#8140,#8141,#8142,#8143,#8144,#8145,
#8146,#8147,#8148,#8149,#8150,#8151,#8152,#8153,#8154,#8155,#8156)) ;
#8596=AXIS2_PLACEMENT_3D('',#13718,#9929,#9930) ;
#8597=AXIS2_PLACEMENT_3D('',#13719,#9931,#9932) ;
#8598=AXIS2_PLACEMENT_3D('',#13735,#9934,#9935) ;
#8599=AXIS2_PLACEMENT_3D('',#13743,#9936,#9937) ;
#8600=AXIS2_PLACEMENT_3D('',#13791,#9939,#9940) ;
#8601=AXIS2_PLACEMENT_3D('',#13839,#9942,#9943) ;
#8602=AXIS2_PLACEMENT_3D('',#13893,#9945,#9946) ;
#8603=AXIS2_PLACEMENT_3D('',#13941,#9948,#9949) ;
#8604=AXIS2_PLACEMENT_3D('',#13989,#9951,#9952) ;
#8605=AXIS2_PLACEMENT_3D('',#14043,#9954,#9955) ;
#8606=AXIS2_PLACEMENT_3D('',#14091,#9957,#9958) ;
#8607=AXIS2_PLACEMENT_3D('',#14139,#9960,#9961) ;
#8608=AXIS2_PLACEMENT_3D('',#14187,#9963,#9964) ;
#8609=AXIS2_PLACEMENT_3D('',#14241,#9966,#9967) ;
#8610=AXIS2_PLACEMENT_3D('',#14289,#9969,#9970) ;
#8611=AXIS2_PLACEMENT_3D('',#14337,#9972,#9973) ;
#8612=AXIS2_PLACEMENT_3D('',#14342,#9975,#9976) ;
#8613=AXIS2_PLACEMENT_3D('',#14390,#9977,#9978) ;
#8614=AXIS2_PLACEMENT_3D('',#14404,#9980,#9981) ;
#8615=AXIS2_PLACEMENT_3D('',#14411,#9982,#9983) ;
#8616=AXIS2_PLACEMENT_3D('',#14436,#9985,#9986) ;
#8617=AXIS2_PLACEMENT_3D('',#14460,#9988,#9989) ;
#8618=AXIS2_PLACEMENT_3D('',#14485,#9991,#9992) ;
#8619=AXIS2_PLACEMENT_3D('',#14510,#9994,#9995) ;
#8620=AXIS2_PLACEMENT_3D('',#14534,#9997,#9998) ;
#8621=AXIS2_PLACEMENT_3D('',#14558,#10000,#10001) ;
#8622=AXIS2_PLACEMENT_3D('',#14583,#10003,#10004) ;
#8623=AXIS2_PLACEMENT_3D('',#14608,#10006,#10007) ;
#8624=AXIS2_PLACEMENT_3D('',#14632,#10009,#10010) ;
#8625=AXIS2_PLACEMENT_3D('',#14657,#10012,#10013) ;
#8626=AXIS2_PLACEMENT_3D('',#14682,#10015,#10016) ;
#8627=AXIS2_PLACEMENT_3D('',#14706,#10018,#10019) ;
#8628=AXIS2_PLACEMENT_3D('',#14796,#10020,#10021) ;
#8629=AXIS2_PLACEMENT_3D('',#15343,#10022,#10023) ;
#8630=AXIS2_PLACEMENT_3D('',#15345,#10024,#10025) ;
#8631=AXIS2_PLACEMENT_3D('',#15435,#10026,#10027) ;
#8632=AXIS2_PLACEMENT_3D('',#15436,#10028,#10029) ;
#8633=AXIS2_PLACEMENT_3D('',#15437,#10030,#10031) ;
#8634=AXIS2_PLACEMENT_3D('',#15802,#10032,#10033) ;
#8635=AXIS2_PLACEMENT_3D('',#15804,#10034,#10035) ;
#8636=AXIS2_PLACEMENT_3D('',#15805,#10036,#10037) ;
#8637=AXIS2_PLACEMENT_3D('',#15806,#10038,#10039) ;
#8638=AXIS2_PLACEMENT_3D('',#15807,#10040,#10041) ;
#8639=AXIS2_PLACEMENT_3D('',#15808,#10042,#10043) ;
#8640=AXIS2_PLACEMENT_3D('',#15810,#10044,#10045) ;
#8641=AXIS2_PLACEMENT_3D('',#15811,#10046,#10047) ;
#8642=AXIS2_PLACEMENT_3D('',#15814,#10049,#10050) ;
#8643=AXIS2_PLACEMENT_3D('',#15815,#10051,#10052) ;
#8644=AXIS2_PLACEMENT_3D('',#15816,#10053,#10054) ;
#8645=AXIS2_PLACEMENT_3D('',#15827,#10058,#10059) ;
#8646=AXIS2_PLACEMENT_3D('',#15829,#10060,#10061) ;
#8647=AXIS2_PLACEMENT_3D('',#15831,#10063,#10064) ;
#8648=AXIS2_PLACEMENT_3D('',#15837,#10066,#10067) ;
#8649=AXIS2_PLACEMENT_3D('',#15839,#10068,#10069) ;
#8650=AXIS2_PLACEMENT_3D('',#15843,#10071,#10072) ;
#8651=AXIS2_PLACEMENT_3D('',#15847,#10074,#10075) ;
#8652=AXIS2_PLACEMENT_3D('',#15851,#10077,#10078) ;
#8653=AXIS2_PLACEMENT_3D('',#15855,#10080,#10081) ;
#8654=AXIS2_PLACEMENT_3D('',#15859,#10083,#10084) ;
#8655=AXIS2_PLACEMENT_3D('',#15863,#10086,#10087) ;
#8656=AXIS2_PLACEMENT_3D('',#15867,#10089,#10090) ;
#8657=AXIS2_PLACEMENT_3D('',#15871,#10092,#10093) ;
#8658=AXIS2_PLACEMENT_3D('',#15875,#10095,#10096) ;
#8659=AXIS2_PLACEMENT_3D('',#15879,#10098,#10099) ;
#8660=AXIS2_PLACEMENT_3D('',#15883,#10101,#10102) ;
#8661=AXIS2_PLACEMENT_3D('',#15887,#10104,#10105) ;
#8662=AXIS2_PLACEMENT_3D('',#15891,#10107,#10108) ;
#8663=AXIS2_PLACEMENT_3D('',#15895,#10110,#10111) ;
#8664=AXIS2_PLACEMENT_3D('',#15899,#10113,#10114) ;
#8665=AXIS2_PLACEMENT_3D('',#15903,#10116,#10117) ;
#8666=AXIS2_PLACEMENT_3D('',#15907,#10119,#10120) ;
#8667=AXIS2_PLACEMENT_3D('',#15911,#10122,#10123) ;
#8668=AXIS2_PLACEMENT_3D('',#15915,#10125,#10126) ;
#8669=AXIS2_PLACEMENT_3D('',#15919,#10128,#10129) ;
#8670=AXIS2_PLACEMENT_3D('',#15923,#10131,#10132) ;
#8671=AXIS2_PLACEMENT_3D('',#15927,#10134,#10135) ;
#8672=AXIS2_PLACEMENT_3D('',#15931,#10137,#10138) ;
#8673=AXIS2_PLACEMENT_3D('',#15935,#10140,#10141) ;
#8674=AXIS2_PLACEMENT_3D('',#15939,#10143,#10144) ;
#8675=AXIS2_PLACEMENT_3D('',#15943,#10146,#10147) ;
#8676=AXIS2_PLACEMENT_3D('',#15947,#10149,#10150) ;
#8677=AXIS2_PLACEMENT_3D('',#15951,#10152,#10153) ;
#8678=AXIS2_PLACEMENT_3D('',#15955,#10155,#10156) ;
#8679=AXIS2_PLACEMENT_3D('',#15959,#10158,#10159) ;
#8680=AXIS2_PLACEMENT_3D('',#15963,#10161,#10162) ;
#8681=AXIS2_PLACEMENT_3D('',#15967,#10164,#10165) ;
#8682=AXIS2_PLACEMENT_3D('',#15971,#10167,#10168) ;
#8683=AXIS2_PLACEMENT_3D('',#15975,#10170,#10171) ;
#8684=AXIS2_PLACEMENT_3D('',#15979,#10173,#10174) ;
#8685=AXIS2_PLACEMENT_3D('',#15983,#10176,#10177) ;
#8686=AXIS2_PLACEMENT_3D('',#15987,#10179,#10180) ;
#8687=AXIS2_PLACEMENT_3D('',#15991,#10182,#10183) ;
#8688=AXIS2_PLACEMENT_3D('',#15995,#10185,#10186) ;
#8689=AXIS2_PLACEMENT_3D('',#15999,#10188,#10189) ;
#8690=AXIS2_PLACEMENT_3D('',#16003,#10191,#10192) ;
#8691=AXIS2_PLACEMENT_3D('',#16007,#10194,#10195) ;
#8692=AXIS2_PLACEMENT_3D('',#16011,#10197,#10198) ;
#8693=AXIS2_PLACEMENT_3D('',#16015,#10200,#10201) ;
#8694=AXIS2_PLACEMENT_3D('',#16019,#10203,#10204) ;
#8695=AXIS2_PLACEMENT_3D('',#16023,#10206,#10207) ;
#8696=AXIS2_PLACEMENT_3D('',#16027,#10209,#10210) ;
#8697=AXIS2_PLACEMENT_3D('',#16031,#10212,#10213) ;
#8698=AXIS2_PLACEMENT_3D('',#16035,#10215,#10216) ;
#8699=AXIS2_PLACEMENT_3D('',#16039,#10218,#10219) ;
#8700=AXIS2_PLACEMENT_3D('',#16043,#10221,#10222) ;
#8701=AXIS2_PLACEMENT_3D('',#16047,#10224,#10225) ;
#8702=AXIS2_PLACEMENT_3D('',#16051,#10227,#10228) ;
#8703=AXIS2_PLACEMENT_3D('',#16055,#10230,#10231) ;
#8704=AXIS2_PLACEMENT_3D('',#16059,#10233,#10234) ;
#8705=AXIS2_PLACEMENT_3D('',#16062,#10236,#10237) ;
#8706=AXIS2_PLACEMENT_3D('',#16064,#10238,#10239) ;
#8707=AXIS2_PLACEMENT_3D('',#16068,#10241,#10242) ;
#8708=AXIS2_PLACEMENT_3D('',#16072,#10244,#10245) ;
#8709=AXIS2_PLACEMENT_3D('',#16076,#10247,#10248) ;
#8710=AXIS2_PLACEMENT_3D('',#16080,#10250,#10251) ;
#8711=AXIS2_PLACEMENT_3D('',#16084,#10253,#10254) ;
#8712=AXIS2_PLACEMENT_3D('',#16088,#10256,#10257) ;
#8713=AXIS2_PLACEMENT_3D('',#16092,#10259,#10260) ;
#8714=AXIS2_PLACEMENT_3D('',#16096,#10262,#10263) ;
#8715=AXIS2_PLACEMENT_3D('',#16100,#10265,#10266) ;
#8716=AXIS2_PLACEMENT_3D('',#16104,#10268,#10269) ;
#8717=AXIS2_PLACEMENT_3D('',#16108,#10271,#10272) ;
#8718=AXIS2_PLACEMENT_3D('',#16112,#10274,#10275) ;
#8719=AXIS2_PLACEMENT_3D('',#16116,#10277,#10278) ;
#8720=AXIS2_PLACEMENT_3D('',#16120,#10280,#10281) ;
#8721=AXIS2_PLACEMENT_3D('',#16123,#10283,#10284) ;
#8722=AXIS2_PLACEMENT_3D('',#16124,#10285,#10286) ;
#8723=AXIS2_PLACEMENT_3D('',#16132,#10289,#10290) ;
#8724=AXIS2_PLACEMENT_3D('',#16134,#10292,#10293) ;
#8725=AXIS2_PLACEMENT_3D('',#16138,#10294,#10295) ;
#8726=AXIS2_PLACEMENT_3D('',#16146,#10298,#10299) ;
#8727=AXIS2_PLACEMENT_3D('',#16148,#10301,#10302) ;
#8728=AXIS2_PLACEMENT_3D('',#16152,#10303,#10304) ;
#8729=AXIS2_PLACEMENT_3D('',#16160,#10307,#10308) ;
#8730=AXIS2_PLACEMENT_3D('',#16162,#10310,#10311) ;
#8731=AXIS2_PLACEMENT_3D('',#16166,#10312,#10313) ;
#8732=AXIS2_PLACEMENT_3D('',#16174,#10316,#10317) ;
#8733=AXIS2_PLACEMENT_3D('',#16176,#10319,#10320) ;
#8734=AXIS2_PLACEMENT_3D('',#16180,#10321,#10322) ;
#8735=AXIS2_PLACEMENT_3D('',#16188,#10325,#10326) ;
#8736=AXIS2_PLACEMENT_3D('',#16190,#10328,#10329) ;
#8737=AXIS2_PLACEMENT_3D('',#16194,#10330,#10331) ;
#8738=AXIS2_PLACEMENT_3D('',#16202,#10334,#10335) ;
#8739=AXIS2_PLACEMENT_3D('',#16204,#10337,#10338) ;
#8740=AXIS2_PLACEMENT_3D('',#16208,#10339,#10340) ;
#8741=AXIS2_PLACEMENT_3D('',#16216,#10343,#10344) ;
#8742=AXIS2_PLACEMENT_3D('',#16218,#10346,#10347) ;
#8743=AXIS2_PLACEMENT_3D('',#16222,#10348,#10349) ;
#8744=AXIS2_PLACEMENT_3D('',#16230,#10352,#10353) ;
#8745=AXIS2_PLACEMENT_3D('',#16232,#10355,#10356) ;
#8746=AXIS2_PLACEMENT_3D('',#16236,#10357,#10358) ;
#8747=AXIS2_PLACEMENT_3D('',#16244,#10361,#10362) ;
#8748=AXIS2_PLACEMENT_3D('',#16246,#10364,#10365) ;
#8749=AXIS2_PLACEMENT_3D('',#16250,#10366,#10367) ;
#8750=AXIS2_PLACEMENT_3D('',#16258,#10370,#10371) ;
#8751=AXIS2_PLACEMENT_3D('',#16260,#10373,#10374) ;
#8752=AXIS2_PLACEMENT_3D('',#16264,#10375,#10376) ;
#8753=AXIS2_PLACEMENT_3D('',#16272,#10379,#10380) ;
#8754=AXIS2_PLACEMENT_3D('',#16274,#10382,#10383) ;
#8755=AXIS2_PLACEMENT_3D('',#16278,#10384,#10385) ;
#8756=AXIS2_PLACEMENT_3D('',#16286,#10388,#10389) ;
#8757=AXIS2_PLACEMENT_3D('',#16288,#10391,#10392) ;
#8758=AXIS2_PLACEMENT_3D('',#16292,#10393,#10394) ;
#8759=AXIS2_PLACEMENT_3D('',#16300,#10397,#10398) ;
#8760=AXIS2_PLACEMENT_3D('',#16302,#10400,#10401) ;
#8761=AXIS2_PLACEMENT_3D('',#16306,#10402,#10403) ;
#8762=AXIS2_PLACEMENT_3D('',#16314,#10406,#10407) ;
#8763=AXIS2_PLACEMENT_3D('',#16316,#10409,#10410) ;
#8764=AXIS2_PLACEMENT_3D('',#16320,#10411,#10412) ;
#8765=AXIS2_PLACEMENT_3D('',#16328,#10415,#10416) ;
#8766=AXIS2_PLACEMENT_3D('',#16330,#10418,#10419) ;
#8767=AXIS2_PLACEMENT_3D('',#16334,#10420,#10421) ;
#8768=AXIS2_PLACEMENT_3D('',#16342,#10424,#10425) ;
#8769=AXIS2_PLACEMENT_3D('',#16344,#10427,#10428) ;
#8770=AXIS2_PLACEMENT_3D('',#16348,#10429,#10430) ;
#8771=AXIS2_PLACEMENT_3D('',#16356,#10433,#10434) ;
#8772=AXIS2_PLACEMENT_3D('',#16358,#10436,#10437) ;
#8773=AXIS2_PLACEMENT_3D('',#16362,#10438,#10439) ;
#8774=AXIS2_PLACEMENT_3D('',#16370,#10442,#10443) ;
#8775=AXIS2_PLACEMENT_3D('',#16372,#10445,#10446) ;
#8776=AXIS2_PLACEMENT_3D('',#16376,#10447,#10448) ;
#8777=AXIS2_PLACEMENT_3D('',#16384,#10451,#10452) ;
#8778=AXIS2_PLACEMENT_3D('',#16386,#10454,#10455) ;
#8779=AXIS2_PLACEMENT_3D('',#16390,#10456,#10457) ;
#8780=AXIS2_PLACEMENT_3D('',#16398,#10460,#10461) ;
#8781=AXIS2_PLACEMENT_3D('',#16400,#10463,#10464) ;
#8782=AXIS2_PLACEMENT_3D('',#16404,#10465,#10466) ;
#8783=AXIS2_PLACEMENT_3D('',#16412,#10469,#10470) ;
#8784=AXIS2_PLACEMENT_3D('',#16414,#10472,#10473) ;
#8785=AXIS2_PLACEMENT_3D('',#16418,#10474,#10475) ;
#8786=AXIS2_PLACEMENT_3D('',#16426,#10478,#10479) ;
#8787=AXIS2_PLACEMENT_3D('',#16428,#10481,#10482) ;
#8788=AXIS2_PLACEMENT_3D('',#16432,#10483,#10484) ;
#8789=AXIS2_PLACEMENT_3D('',#16440,#10487,#10488) ;
#8790=AXIS2_PLACEMENT_3D('',#16442,#10490,#10491) ;
#8791=AXIS2_PLACEMENT_3D('',#16446,#10492,#10493) ;
#8792=AXIS2_PLACEMENT_3D('',#16454,#10496,#10497) ;
#8793=AXIS2_PLACEMENT_3D('',#16456,#10499,#10500) ;
#8794=AXIS2_PLACEMENT_3D('',#16460,#10501,#10502) ;
#8795=AXIS2_PLACEMENT_3D('',#16468,#10505,#10506) ;
#8796=AXIS2_PLACEMENT_3D('',#16470,#10508,#10509) ;
#8797=AXIS2_PLACEMENT_3D('',#16474,#10510,#10511) ;
#8798=AXIS2_PLACEMENT_3D('',#16482,#10514,#10515) ;
#8799=AXIS2_PLACEMENT_3D('',#16484,#10517,#10518) ;
#8800=AXIS2_PLACEMENT_3D('',#16488,#10519,#10520) ;
#8801=AXIS2_PLACEMENT_3D('',#16496,#10523,#10524) ;
#8802=AXIS2_PLACEMENT_3D('',#16498,#10526,#10527) ;
#8803=AXIS2_PLACEMENT_3D('',#16502,#10528,#10529) ;
#8804=AXIS2_PLACEMENT_3D('',#16510,#10532,#10533) ;
#8805=AXIS2_PLACEMENT_3D('',#16512,#10535,#10536) ;
#8806=AXIS2_PLACEMENT_3D('',#16516,#10537,#10538) ;
#8807=AXIS2_PLACEMENT_3D('',#16524,#10541,#10542) ;
#8808=AXIS2_PLACEMENT_3D('',#16526,#10544,#10545) ;
#8809=AXIS2_PLACEMENT_3D('',#16530,#10546,#10547) ;
#8810=AXIS2_PLACEMENT_3D('',#16538,#10550,#10551) ;
#8811=AXIS2_PLACEMENT_3D('',#16540,#10553,#10554) ;
#8812=AXIS2_PLACEMENT_3D('',#16544,#10555,#10556) ;
#8813=AXIS2_PLACEMENT_3D('',#16552,#10559,#10560) ;
#8814=AXIS2_PLACEMENT_3D('',#16554,#10562,#10563) ;
#8815=AXIS2_PLACEMENT_3D('',#16558,#10564,#10565) ;
#8816=AXIS2_PLACEMENT_3D('',#16566,#10568,#10569) ;
#8817=AXIS2_PLACEMENT_3D('',#16568,#10571,#10572) ;
#8818=AXIS2_PLACEMENT_3D('',#16572,#10573,#10574) ;
#8819=AXIS2_PLACEMENT_3D('',#16580,#10577,#10578) ;
#8820=AXIS2_PLACEMENT_3D('',#16582,#10580,#10581) ;
#8821=AXIS2_PLACEMENT_3D('',#16586,#10582,#10583) ;
#8822=AXIS2_PLACEMENT_3D('',#16594,#10586,#10587) ;
#8823=AXIS2_PLACEMENT_3D('',#16596,#10589,#10590) ;
#8824=AXIS2_PLACEMENT_3D('',#16600,#10591,#10592) ;
#8825=AXIS2_PLACEMENT_3D('',#16608,#10595,#10596) ;
#8826=AXIS2_PLACEMENT_3D('',#16610,#10598,#10599) ;
#8827=AXIS2_PLACEMENT_3D('',#16614,#10600,#10601) ;
#8828=AXIS2_PLACEMENT_3D('',#16615,#10602,#10603) ;
#8829=AXIS2_PLACEMENT_3D('',#16616,#10604,#10605) ;
#8830=AXIS2_PLACEMENT_3D('',#16618,#10606,#10607) ;
#8831=AXIS2_PLACEMENT_3D('',#16620,#10609,#10610) ;
#8832=AXIS2_PLACEMENT_3D('',#16622,#10611,#10612) ;
#8833=AXIS2_PLACEMENT_3D('',#16623,#10613,#10614) ;
#8834=AXIS2_PLACEMENT_3D('',#16630,#10615,#10616) ;
#8835=AXIS2_PLACEMENT_3D('',#16640,#10617,#10618) ;
#8836=AXIS2_PLACEMENT_3D('',#16650,#10619,#10620) ;
#8837=AXIS2_PLACEMENT_3D('',#16660,#10621,#10622) ;
#8838=AXIS2_PLACEMENT_3D('',#16670,#10623,#10624) ;
#8839=AXIS2_PLACEMENT_3D('',#16681,#10626,#10627) ;
#8840=AXIS2_PLACEMENT_3D('',#16685,#10628,#10629) ;
#8841=AXIS2_PLACEMENT_3D('',#16690,#10632,#10633) ;
#8842=AXIS2_PLACEMENT_3D('',#16691,#10634,#10635) ;
#8843=AXIS2_PLACEMENT_3D('',#16695,#10637,#10638) ;
#8844=AXIS2_PLACEMENT_3D('',#16697,#10640,#10641) ;
#8845=AXIS2_PLACEMENT_3D('',#16702,#10644,#10645) ;
#8846=AXIS2_PLACEMENT_3D('',#16703,#10646,#10647) ;
#8847=AXIS2_PLACEMENT_3D('',#16707,#10649,#10650) ;
#8848=AXIS2_PLACEMENT_3D('',#16709,#10652,#10653) ;
#8849=AXIS2_PLACEMENT_3D('',#16714,#10656,#10657) ;
#8850=AXIS2_PLACEMENT_3D('',#16715,#10658,#10659) ;
#8851=AXIS2_PLACEMENT_3D('',#16719,#10661,#10662) ;
#8852=AXIS2_PLACEMENT_3D('',#16721,#10664,#10665) ;
#8853=AXIS2_PLACEMENT_3D('',#16728,#10670,#10671) ;
#8854=AXIS2_PLACEMENT_3D('',#16733,#10675,#10676) ;
#8855=AXIS2_PLACEMENT_3D('',#16738,#10680,#10681) ;
#8856=AXIS2_PLACEMENT_3D('',#16739,#10682,#10683) ;
#8857=AXIS2_PLACEMENT_3D('',#16740,#10684,#10685) ;
#8858=AXIS2_PLACEMENT_3D('',#16742,#10687,#10688) ;
#8859=AXIS2_PLACEMENT_3D('',#16743,#10689,#10690) ;
#8860=AXIS2_PLACEMENT_3D('',#16745,#10692,#10693) ;
#8861=AXIS2_PLACEMENT_3D('',#16747,#10695,#10696) ;
#8862=AXIS2_PLACEMENT_3D('',#16751,#10698,#10699) ;
#8863=AXIS2_PLACEMENT_3D('',#16752,#10700,#10701) ;
#8864=AXIS2_PLACEMENT_3D('',#16754,#10703,#10704) ;
#8865=AXIS2_PLACEMENT_3D('',#16755,#10705,#10706) ;
#8866=AXIS2_PLACEMENT_3D('',#16756,#10707,#10708) ;
#8867=AXIS2_PLACEMENT_3D('',#16757,#10709,#10710) ;
#8868=AXIS2_PLACEMENT_3D('',#16758,#10711,#10712) ;
#8869=AXIS2_PLACEMENT_3D('',#16759,#10713,#10714) ;
#8870=AXIS2_PLACEMENT_3D('',#16760,#10715,#10716) ;
#8871=AXIS2_PLACEMENT_3D('',#16761,#10717,#10718) ;
#8872=AXIS2_PLACEMENT_3D('',#16763,#10720,#10721) ;
#8873=AXIS2_PLACEMENT_3D('',#16764,#10722,#10723) ;
#8874=AXIS2_PLACEMENT_3D('',#16767,#10725,#10726) ;
#8875=AXIS2_PLACEMENT_3D('',#16770,#10729,#10730) ;
#8876=AXIS2_PLACEMENT_3D('',#16771,#10731,#10732) ;
#9929=DIRECTION('axis',(0.,0.,1.)) ;
#9930=DIRECTION('refdir',(1.,0.,0.)) ;
#9931=DIRECTION('center_axis',(-1.,0.,0.)) ;
#9932=DIRECTION('ref_axis',(0.,0.,-1.)) ;
#9933=DIRECTION('',(1.,0.,0.)) ;
#9934=DIRECTION('center_axis',(1.,0.,0.)) ;
#9935=DIRECTION('ref_axis',(0.,0.,-1.)) ;
#9936=DIRECTION('center_axis',(-1.,0.,0.)) ;
#9937=DIRECTION('ref_axis',(0.,0.,-1.)) ;
#9938=DIRECTION('',(1.,0.,0.)) ;
#9939=DIRECTION('center_axis',(-1.,0.,0.)) ;
#9940=DIRECTION('ref_axis',(0.,0.,-1.)) ;
#9941=DIRECTION('',(1.,0.,0.)) ;
#9942=DIRECTION('center_axis',(-1.,0.,0.)) ;
#9943=DIRECTION('ref_axis',(0.,0.,-1.)) ;
#9944=DIRECTION('',(1.,0.,0.)) ;
#9945=DIRECTION('center_axis',(-1.,0.,0.)) ;
#9946=DIRECTION('ref_axis',(0.,0.,-1.)) ;
#9947=DIRECTION('',(1.,0.,0.)) ;
#9948=DIRECTION('center_axis',(-1.,0.,0.)) ;
#9949=DIRECTION('ref_axis',(0.,0.,-1.)) ;
#9950=DIRECTION('',(1.,0.,0.)) ;
#9951=DIRECTION('center_axis',(-1.,0.,0.)) ;
#9952=DIRECTION('ref_axis',(0.,0.,-1.)) ;
#9953=DIRECTION('',(1.,0.,0.)) ;
#9954=DIRECTION('center_axis',(-1.,0.,0.)) ;
#9955=DIRECTION('ref_axis',(0.,0.,-1.)) ;
#9956=DIRECTION('',(1.,0.,0.)) ;
#9957=DIRECTION('center_axis',(-1.,0.,0.)) ;
#9958=DIRECTION('ref_axis',(0.,0.,-1.)) ;
#9959=DIRECTION('',(1.,0.,0.)) ;
#9960=DIRECTION('center_axis',(-1.,0.,0.)) ;
#9961=DIRECTION('ref_axis',(0.,0.,-1.)) ;
#9962=DIRECTION('',(1.,0.,0.)) ;
#9963=DIRECTION('center_axis',(-1.,0.,0.)) ;
#9964=DIRECTION('ref_axis',(0.,0.,-1.)) ;
#9965=DIRECTION('',(1.,0.,0.)) ;
#9966=DIRECTION('center_axis',(-1.,0.,0.)) ;
#9967=DIRECTION('ref_axis',(0.,0.,-1.)) ;
#9968=DIRECTION('',(1.,0.,0.)) ;
#9969=DIRECTION('center_axis',(-1.,0.,0.)) ;
#9970=DIRECTION('ref_axis',(0.,0.,-1.)) ;
#9971=DIRECTION('',(1.,0.,0.)) ;
#9972=DIRECTION('center_axis',(-1.,0.,0.)) ;
#9973=DIRECTION('ref_axis',(0.,0.,-1.)) ;
#9974=DIRECTION('',(1.,0.,0.)) ;
#9975=DIRECTION('center_axis',(-1.,0.,0.)) ;
#9976=DIRECTION('ref_axis',(0.,0.,-1.)) ;
#9977=DIRECTION('center_axis',(-1.,0.,0.)) ;
#9978=DIRECTION('ref_axis',(0.,0.912319398217867,-0.409479322598088)) ;
#9979=DIRECTION('',(-1.,0.,0.)) ;
#9980=DIRECTION('center_axis',(-1.,0.,0.)) ;
#9981=DIRECTION('ref_axis',(0.,-7.70839515651023E-14,-1.)) ;
#9982=DIRECTION('center_axis',(-1.,0.,0.)) ;
#9983=DIRECTION('ref_axis',(0.,-7.70839515651023E-14,-1.)) ;
#9984=DIRECTION('',(-1.,0.,0.)) ;
#9985=DIRECTION('center_axis',(-1.,0.,0.)) ;
#9986=DIRECTION('ref_axis',(0.,-7.70839515651023E-14,-1.)) ;
#9987=DIRECTION('',(-1.,0.,0.)) ;
#9988=DIRECTION('center_axis',(-1.,0.,0.)) ;
#9989=DIRECTION('ref_axis',(0.,-7.70839515651023E-14,-1.)) ;
#9990=DIRECTION('',(-1.,0.,0.)) ;
#9991=DIRECTION('center_axis',(-1.,0.,0.)) ;
#9992=DIRECTION('ref_axis',(0.,-7.70839515651023E-14,-1.)) ;
#9993=DIRECTION('',(-1.,0.,0.)) ;
#9994=DIRECTION('center_axis',(-1.,0.,0.)) ;
#9995=DIRECTION('ref_axis',(0.,-7.70839515651023E-14,-1.)) ;
#9996=DIRECTION('',(-1.,0.,0.)) ;
#9997=DIRECTION('center_axis',(-1.,0.,0.)) ;
#9998=DIRECTION('ref_axis',(0.,-7.70839515651023E-14,-1.)) ;
#9999=DIRECTION('',(-1.,0.,0.)) ;
#10000=DIRECTION('center_axis',(-1.,0.,0.)) ;
#10001=DIRECTION('ref_axis',(0.,-7.70839515651023E-14,-1.)) ;
#10002=DIRECTION('',(-1.,0.,0.)) ;
#10003=DIRECTION('center_axis',(-1.,0.,0.)) ;
#10004=DIRECTION('ref_axis',(0.,-7.70839515651023E-14,-1.)) ;
#10005=DIRECTION('',(-1.,0.,0.)) ;
#10006=DIRECTION('center_axis',(-1.,0.,0.)) ;
#10007=DIRECTION('ref_axis',(0.,-7.70839515651023E-14,-1.)) ;
#10008=DIRECTION('',(-1.,0.,0.)) ;
#10009=DIRECTION('center_axis',(-1.,0.,0.)) ;
#10010=DIRECTION('ref_axis',(0.,-7.70839515651023E-14,-1.)) ;
#10011=DIRECTION('',(-1.,0.,0.)) ;
#10012=DIRECTION('center_axis',(-1.,0.,0.)) ;
#10013=DIRECTION('ref_axis',(0.,-7.70839515651023E-14,-1.)) ;
#10014=DIRECTION('',(-1.,0.,0.)) ;
#10015=DIRECTION('center_axis',(-1.,0.,0.)) ;
#10016=DIRECTION('ref_axis',(0.,-7.70839515651023E-14,-1.)) ;
#10017=DIRECTION('',(-1.,0.,0.)) ;
#10018=DIRECTION('center_axis',(1.,0.,0.)) ;
#10019=DIRECTION('ref_axis',(0.,0.,-1.)) ;
#10020=DIRECTION('center_axis',(-1.,0.,0.)) ;
#10021=DIRECTION('ref_axis',(0.,0.,-1.)) ;
#10022=DIRECTION('center_axis',(1.,0.,0.)) ;
#10023=DIRECTION('ref_axis',(0.,0.,-1.)) ;
#10024=DIRECTION('center_axis',(1.,0.,0.)) ;
#10025=DIRECTION('ref_axis',(0.,0.,-1.)) ;
#10026=DIRECTION('center_axis',(1.,0.,0.)) ;
#10027=DIRECTION('ref_axis',(0.,-7.70839515651023E-14,-1.)) ;
#10028=DIRECTION('center_axis',(1.,0.,0.)) ;
#10029=DIRECTION('ref_axis',(0.,0.,-1.)) ;
#10030=DIRECTION('center_axis',(-1.,0.,0.)) ;
#10031=DIRECTION('ref_axis',(0.,-7.70839515651023E-14,-1.)) ;
#10032=DIRECTION('center_axis',(1.,0.,0.)) ;
#10033=DIRECTION('ref_axis',(0.,0.,-1.)) ;
#10034=DIRECTION('center_axis',(0.,-1.,0.)) ;
#10035=DIRECTION('ref_axis',(0.,0.,1.)) ;
#10036=DIRECTION('center_axis',(-1.,0.,0.)) ;
#10037=DIRECTION('ref_axis',(0.,0.,-1.)) ;
#10038=DIRECTION('center_axis',(-1.,0.,0.)) ;
#10039=DIRECTION('ref_axis',(0.,0.33373437595002,0.942667155633021)) ;
#10040=DIRECTION('center_axis',(-1.,0.,0.)) ;
#10041=DIRECTION('ref_axis',(0.,0.,-1.)) ;
#10042=DIRECTION('center_axis',(1.,0.,0.)) ;
#10043=DIRECTION('ref_axis',(0.,0.,-1.)) ;
#10044=DIRECTION('center_axis',(1.,0.,0.)) ;
#10045=DIRECTION('ref_axis',(0.,0.,-1.)) ;
#10046=DIRECTION('center_axis',(1.,0.,0.)) ;
#10047=DIRECTION('ref_axis',(0.,0.,-1.)) ;
#10048=DIRECTION('',(-0.707106781186548,8.65956056235493E-17,-0.707106781186548)) ;
#10049=DIRECTION('center_axis',(1.,0.,0.)) ;
#10050=DIRECTION('ref_axis',(0.,0.,-1.)) ;
#10051=DIRECTION('center_axis',(1.,0.,0.)) ;
#10052=DIRECTION('ref_axis',(0.,0.,-1.)) ;
#10053=DIRECTION('center_axis',(0.,-0.588540350318076,0.808467844782634)) ;
#10054=DIRECTION('ref_axis',(0.,0.808467844782634,0.588540350318076)) ;
#10055=DIRECTION('',(-1.,0.,0.)) ;
#10056=DIRECTION('',(0.,0.808467844782634,0.588540350318076)) ;
#10057=DIRECTION('',(-1.,0.,0.)) ;
#10058=DIRECTION('center_axis',(-1.,0.,0.)) ;
#10059=DIRECTION('ref_axis',(0.,-0.17364817766693,0.984807753012208)) ;
#10060=DIRECTION('center_axis',(-1.,0.,0.)) ;
#10061=DIRECTION('ref_axis',(0.,0.,-1.)) ;
#10062=DIRECTION('',(0.,-0.961003922853656,0.276534736081898)) ;
#10063=DIRECTION('center_axis',(0.,-0.276534736081898,-0.961003922853656)) ;
#10064=DIRECTION('ref_axis',(0.,-0.961003922853656,0.276534736081898)) ;
#10065=DIRECTION('',(1.,0.,0.)) ;
#10066=DIRECTION('center_axis',(1.,0.,0.)) ;
#10067=DIRECTION('ref_axis',(0.,0.,-1.)) ;
#10068=DIRECTION('center_axis',(1.,0.,0.)) ;
#10069=DIRECTION('ref_axis',(0.,0.,-1.)) ;
#10070=DIRECTION('',(-1.,0.,0.)) ;
#10071=DIRECTION('center_axis',(-1.,0.,0.)) ;
#10072=DIRECTION('ref_axis',(0.,0.,-1.)) ;
#10073=DIRECTION('',(1.,0.,0.)) ;
#10074=DIRECTION('center_axis',(1.,0.,0.)) ;
#10075=DIRECTION('ref_axis',(0.,0.,-1.)) ;
#10076=DIRECTION('',(-1.,0.,0.)) ;
#10077=DIRECTION('center_axis',(-1.,0.,0.)) ;
#10078=DIRECTION('ref_axis',(0.,0.,-1.)) ;
#10079=DIRECTION('',(1.,0.,0.)) ;
#10080=DIRECTION('center_axis',(1.,0.,0.)) ;
#10081=DIRECTION('ref_axis',(0.,0.,-1.)) ;
#10082=DIRECTION('',(-1.,0.,0.)) ;
#10083=DIRECTION('center_axis',(-1.,0.,0.)) ;
#10084=DIRECTION('ref_axis',(0.,0.,-1.)) ;
#10085=DIRECTION('',(1.,0.,0.)) ;
#10086=DIRECTION('center_axis',(1.,0.,0.)) ;
#10087=DIRECTION('ref_axis',(0.,0.,-1.)) ;
#10088=DIRECTION('',(-1.,0.,0.)) ;
#10089=DIRECTION('center_axis',(-1.,0.,0.)) ;
#10090=DIRECTION('ref_axis',(0.,0.,-1.)) ;
#10091=DIRECTION('',(1.,0.,0.)) ;
#10092=DIRECTION('center_axis',(1.,0.,0.)) ;
#10093=DIRECTION('ref_axis',(0.,0.,-1.)) ;
#10094=DIRECTION('',(-1.,0.,0.)) ;
#10095=DIRECTION('center_axis',(-1.,0.,0.)) ;
#10096=DIRECTION('ref_axis',(0.,0.,-1.)) ;
#10097=DIRECTION('',(1.,0.,0.)) ;
#10098=DIRECTION('center_axis',(1.,0.,0.)) ;
#10099=DIRECTION('ref_axis',(0.,0.,-1.)) ;
#10100=DIRECTION('',(-1.,0.,0.)) ;
#10101=DIRECTION('center_axis',(-1.,0.,0.)) ;
#10102=DIRECTION('ref_axis',(0.,0.,-1.)) ;
#10103=DIRECTION('',(1.,0.,0.)) ;
#10104=DIRECTION('center_axis',(1.,0.,0.)) ;
#10105=DIRECTION('ref_axis',(0.,0.,-1.)) ;
#10106=DIRECTION('',(-1.,0.,0.)) ;
#10107=DIRECTION('center_axis',(-1.,0.,0.)) ;
#10108=DIRECTION('ref_axis',(0.,0.,-1.)) ;
#10109=DIRECTION('',(1.,0.,0.)) ;
#10110=DIRECTION('center_axis',(1.,0.,0.)) ;
#10111=DIRECTION('ref_axis',(0.,0.,-1.)) ;
#10112=DIRECTION('',(-1.,0.,0.)) ;
#10113=DIRECTION('center_axis',(-1.,0.,0.)) ;
#10114=DIRECTION('ref_axis',(0.,0.,-1.)) ;
#10115=DIRECTION('',(1.,0.,0.)) ;
#10116=DIRECTION('center_axis',(1.,0.,0.)) ;
#10117=DIRECTION('ref_axis',(0.,0.,-1.)) ;
#10118=DIRECTION('',(-1.,0.,0.)) ;
#10119=DIRECTION('center_axis',(-1.,0.,0.)) ;
#10120=DIRECTION('ref_axis',(0.,0.,-1.)) ;
#10121=DIRECTION('',(1.,0.,0.)) ;
#10122=DIRECTION('center_axis',(1.,0.,0.)) ;
#10123=DIRECTION('ref_axis',(0.,0.,-1.)) ;
#10124=DIRECTION('',(-1.,0.,0.)) ;
#10125=DIRECTION('center_axis',(-1.,0.,0.)) ;
#10126=DIRECTION('ref_axis',(0.,0.,-1.)) ;
#10127=DIRECTION('',(1.,0.,0.)) ;
#10128=DIRECTION('center_axis',(1.,0.,0.)) ;
#10129=DIRECTION('ref_axis',(0.,0.,-1.)) ;
#10130=DIRECTION('',(-1.,0.,0.)) ;
#10131=DIRECTION('center_axis',(-1.,0.,0.)) ;
#10132=DIRECTION('ref_axis',(0.,0.,-1.)) ;
#10133=DIRECTION('',(1.,0.,0.)) ;
#10134=DIRECTION('center_axis',(1.,0.,0.)) ;
#10135=DIRECTION('ref_axis',(0.,0.,-1.)) ;
#10136=DIRECTION('',(-1.,0.,0.)) ;
#10137=DIRECTION('center_axis',(-1.,0.,0.)) ;
#10138=DIRECTION('ref_axis',(0.,0.,-1.)) ;
#10139=DIRECTION('',(1.,0.,0.)) ;
#10140=DIRECTION('center_axis',(1.,0.,0.)) ;
#10141=DIRECTION('ref_axis',(0.,0.,-1.)) ;
#10142=DIRECTION('',(-1.,0.,0.)) ;
#10143=DIRECTION('center_axis',(-1.,0.,0.)) ;
#10144=DIRECTION('ref_axis',(0.,0.,-1.)) ;
#10145=DIRECTION('',(1.,0.,0.)) ;
#10146=DIRECTION('center_axis',(1.,0.,0.)) ;
#10147=DIRECTION('ref_axis',(0.,0.,-1.)) ;
#10148=DIRECTION('',(-1.,0.,0.)) ;
#10149=DIRECTION('center_axis',(-1.,0.,0.)) ;
#10150=DIRECTION('ref_axis',(0.,0.,-1.)) ;
#10151=DIRECTION('',(1.,0.,0.)) ;
#10152=DIRECTION('center_axis',(1.,0.,0.)) ;
#10153=DIRECTION('ref_axis',(0.,0.,-1.)) ;
#10154=DIRECTION('',(-1.,0.,0.)) ;
#10155=DIRECTION('center_axis',(-1.,0.,0.)) ;
#10156=DIRECTION('ref_axis',(0.,0.,-1.)) ;
#10157=DIRECTION('',(1.,0.,0.)) ;
#10158=DIRECTION('center_axis',(1.,0.,0.)) ;
#10159=DIRECTION('ref_axis',(0.,0.,-1.)) ;
#10160=DIRECTION('',(-1.,0.,0.)) ;
#10161=DIRECTION('center_axis',(-1.,0.,0.)) ;
#10162=DIRECTION('ref_axis',(0.,0.,-1.)) ;
#10163=DIRECTION('',(1.,0.,0.)) ;
#10164=DIRECTION('center_axis',(1.,0.,0.)) ;
#10165=DIRECTION('ref_axis',(0.,0.,-1.)) ;
#10166=DIRECTION('',(-1.,0.,0.)) ;
#10167=DIRECTION('center_axis',(-1.,0.,0.)) ;
#10168=DIRECTION('ref_axis',(0.,0.,-1.)) ;
#10169=DIRECTION('',(1.,0.,0.)) ;
#10170=DIRECTION('center_axis',(1.,0.,0.)) ;
#10171=DIRECTION('ref_axis',(0.,0.,-1.)) ;
#10172=DIRECTION('',(-1.,0.,0.)) ;
#10173=DIRECTION('center_axis',(-1.,0.,0.)) ;
#10174=DIRECTION('ref_axis',(0.,0.,-1.)) ;
#10175=DIRECTION('',(1.,0.,0.)) ;
#10176=DIRECTION('center_axis',(1.,0.,0.)) ;
#10177=DIRECTION('ref_axis',(0.,0.,-1.)) ;
#10178=DIRECTION('',(-1.,0.,0.)) ;
#10179=DIRECTION('center_axis',(-1.,0.,0.)) ;
#10180=DIRECTION('ref_axis',(0.,0.,-1.)) ;
#10181=DIRECTION('',(1.,0.,0.)) ;
#10182=DIRECTION('center_axis',(1.,0.,0.)) ;
#10183=DIRECTION('ref_axis',(0.,0.,-1.)) ;
#10184=DIRECTION('',(-1.,0.,0.)) ;
#10185=DIRECTION('center_axis',(-1.,0.,0.)) ;
#10186=DIRECTION('ref_axis',(0.,0.,-1.)) ;
#10187=DIRECTION('',(1.,0.,0.)) ;
#10188=DIRECTION('center_axis',(1.,0.,0.)) ;
#10189=DIRECTION('ref_axis',(0.,0.,-1.)) ;
#10190=DIRECTION('',(-1.,0.,0.)) ;
#10191=DIRECTION('center_axis',(-1.,0.,0.)) ;
#10192=DIRECTION('ref_axis',(0.,0.,-1.)) ;
#10193=DIRECTION('',(1.,0.,0.)) ;
#10194=DIRECTION('center_axis',(1.,0.,0.)) ;
#10195=DIRECTION('ref_axis',(0.,0.,-1.)) ;
#10196=DIRECTION('',(-1.,0.,0.)) ;
#10197=DIRECTION('center_axis',(-1.,0.,0.)) ;
#10198=DIRECTION('ref_axis',(0.,0.,-1.)) ;
#10199=DIRECTION('',(1.,0.,0.)) ;
#10200=DIRECTION('center_axis',(1.,0.,0.)) ;
#10201=DIRECTION('ref_axis',(0.,0.,-1.)) ;
#10202=DIRECTION('',(-1.,0.,0.)) ;
#10203=DIRECTION('center_axis',(-1.,0.,0.)) ;
#10204=DIRECTION('ref_axis',(0.,0.,-1.)) ;
#10205=DIRECTION('',(1.,0.,0.)) ;
#10206=DIRECTION('center_axis',(1.,0.,0.)) ;
#10207=DIRECTION('ref_axis',(0.,0.,-1.)) ;
#10208=DIRECTION('',(-1.,0.,0.)) ;
#10209=DIRECTION('center_axis',(-1.,0.,0.)) ;
#10210=DIRECTION('ref_axis',(0.,0.,-1.)) ;
#10211=DIRECTION('',(1.,0.,0.)) ;
#10212=DIRECTION('center_axis',(1.,0.,0.)) ;
#10213=DIRECTION('ref_axis',(0.,0.,-1.)) ;
#10214=DIRECTION('',(-1.,0.,0.)) ;
#10215=DIRECTION('center_axis',(-1.,0.,0.)) ;
#10216=DIRECTION('ref_axis',(0.,0.,-1.)) ;
#10217=DIRECTION('',(1.,0.,0.)) ;
#10218=DIRECTION('center_axis',(1.,0.,0.)) ;
#10219=DIRECTION('ref_axis',(0.,0.,-1.)) ;
#10220=DIRECTION('',(-1.,0.,0.)) ;
#10221=DIRECTION('center_axis',(-1.,0.,0.)) ;
#10222=DIRECTION('ref_axis',(0.,0.,-1.)) ;
#10223=DIRECTION('',(1.,0.,0.)) ;
#10224=DIRECTION('center_axis',(1.,0.,0.)) ;
#10225=DIRECTION('ref_axis',(0.,0.,-1.)) ;
#10226=DIRECTION('',(-1.,0.,0.)) ;
#10227=DIRECTION('center_axis',(-1.,0.,0.)) ;
#10228=DIRECTION('ref_axis',(0.,0.,-1.)) ;
#10229=DIRECTION('',(1.,0.,0.)) ;
#10230=DIRECTION('center_axis',(1.,0.,0.)) ;
#10231=DIRECTION('ref_axis',(0.,0.,-1.)) ;
#10232=DIRECTION('',(-1.,0.,0.)) ;
#10233=DIRECTION('center_axis',(-1.,0.,0.)) ;
#10234=DIRECTION('ref_axis',(0.,0.,-1.)) ;
#10235=DIRECTION('',(-1.,0.,0.)) ;
#10236=DIRECTION('center_axis',(-1.,0.,0.)) ;
#10237=DIRECTION('ref_axis',(0.,0.,-1.)) ;
#10238=DIRECTION('center_axis',(-1.,0.,0.)) ;
#10239=DIRECTION('ref_axis',(0.,0.,-1.)) ;
#10240=DIRECTION('',(1.,0.,0.)) ;
#10241=DIRECTION('center_axis',(1.,0.,0.)) ;
#10242=DIRECTION('ref_axis',(0.,0.,-1.)) ;
#10243=DIRECTION('',(-1.,0.,0.)) ;
#10244=DIRECTION('center_axis',(-1.,0.,0.)) ;
#10245=DIRECTION('ref_axis',(0.,0.,-1.)) ;
#10246=DIRECTION('',(1.,0.,0.)) ;
#10247=DIRECTION('center_axis',(1.,0.,0.)) ;
#10248=DIRECTION('ref_axis',(0.,0.,-1.)) ;
#10249=DIRECTION('',(-1.,0.,0.)) ;
#10250=DIRECTION('center_axis',(-1.,0.,0.)) ;
#10251=DIRECTION('ref_axis',(0.,0.,-1.)) ;
#10252=DIRECTION('',(1.,0.,0.)) ;
#10253=DIRECTION('center_axis',(1.,0.,0.)) ;
#10254=DIRECTION('ref_axis',(0.,0.,-1.)) ;
#10255=DIRECTION('',(-1.,0.,0.)) ;
#10256=DIRECTION('center_axis',(-1.,0.,0.)) ;
#10257=DIRECTION('ref_axis',(0.,0.,-1.)) ;
#10258=DIRECTION('',(1.,0.,0.)) ;
#10259=DIRECTION('center_axis',(1.,0.,0.)) ;
#10260=DIRECTION('ref_axis',(0.,0.,-1.)) ;
#10261=DIRECTION('',(-1.,0.,0.)) ;
#10262=DIRECTION('center_axis',(-1.,0.,0.)) ;
#10263=DIRECTION('ref_axis',(0.,0.,-1.)) ;
#10264=DIRECTION('',(1.,0.,0.)) ;
#10265=DIRECTION('center_axis',(1.,0.,0.)) ;
#10266=DIRECTION('ref_axis',(0.,0.,-1.)) ;
#10267=DIRECTION('',(-1.,0.,0.)) ;
#10268=DIRECTION('center_axis',(-1.,0.,0.)) ;
#10269=DIRECTION('ref_axis',(0.,0.,-1.)) ;
#10270=DIRECTION('',(1.,0.,0.)) ;
#10271=DIRECTION('center_axis',(1.,0.,0.)) ;
#10272=DIRECTION('ref_axis',(0.,0.,-1.)) ;
#10273=DIRECTION('',(-1.,0.,0.)) ;
#10274=DIRECTION('center_axis',(-1.,0.,0.)) ;
#10275=DIRECTION('ref_axis',(0.,0.,-1.)) ;
#10276=DIRECTION('',(1.,0.,0.)) ;
#10277=DIRECTION('center_axis',(1.,0.,0.)) ;
#10278=DIRECTION('ref_axis',(0.,0.,-1.)) ;
#10279=DIRECTION('',(-1.,0.,0.)) ;
#10280=DIRECTION('center_axis',(-1.,0.,0.)) ;
#10281=DIRECTION('ref_axis',(0.,0.,-1.)) ;
#10282=DIRECTION('',(1.,0.,0.)) ;
#10283=DIRECTION('center_axis',(1.,0.,0.)) ;
#10284=DIRECTION('ref_axis',(0.,0.,-1.)) ;
#10285=DIRECTION('center_axis',(0.,-0.719988067902578,0.693986442286817)) ;
#10286=DIRECTION('ref_axis',(0.,0.693986442286817,0.719988067902578)) ;
#10287=DIRECTION('',(-1.,0.,0.)) ;
#10288=DIRECTION('',(0.,0.693986442286817,0.719988067902578)) ;
#10289=DIRECTION('center_axis',(-1.,0.,0.)) ;
#10290=DIRECTION('ref_axis',(0.,-0.342020143325669,0.939692620785908)) ;
#10291=DIRECTION('',(0.,-0.994423866883653,0.105456972136329)) ;
#10292=DIRECTION('center_axis',(0.,-0.105456972136329,-0.994423866883653)) ;
#10293=DIRECTION('ref_axis',(0.,-0.994423866883653,0.105456972136329)) ;
#10294=DIRECTION('center_axis',(0.,-0.8295593123754,0.5584186129162)) ;
#10295=DIRECTION('ref_axis',(0.,0.5584186129162,0.8295593123754)) ;
#10296=DIRECTION('',(-1.,0.,0.)) ;
#10297=DIRECTION('',(0.,0.5584186129162,0.8295593123754)) ;
#10298=DIRECTION('center_axis',(-1.,0.,0.)) ;
#10299=DIRECTION('ref_axis',(0.,-0.5,0.866025403784438)) ;
#10300=DIRECTION('',(0.,-0.997628744921147,-0.0688250485437991)) ;
#10301=DIRECTION('center_axis',(0.,0.0688250485437991,-0.997628744921147)) ;
#10302=DIRECTION('ref_axis',(0.,-0.997628744921147,-0.0688250485437991)) ;
#10303=DIRECTION('center_axis',(0.,-0.913924816918964,0.405883516565577)) ;
#10304=DIRECTION('ref_axis',(0.,0.405883516565577,0.913924816918964)) ;
#10305=DIRECTION('',(-1.,0.,0.)) ;
#10306=DIRECTION('',(0.,0.405883516565577,0.913924816918964)) ;
#10307=DIRECTION('center_axis',(-1.,0.,0.)) ;
#10308=DIRECTION('ref_axis',(0.,-0.64278760968654,0.766044443118978)) ;
#10309=DIRECTION('',(0.,-0.970521178368716,-0.241015854951079)) ;
#10310=DIRECTION('center_axis',(0.,0.241015854951079,-0.970521178368716)) ;
#10311=DIRECTION('ref_axis',(0.,-0.970521178368716,-0.241015854951079)) ;
#10312=DIRECTION('center_axis',(0.,-0.970521178368716,0.241015854951078)) ;
#10313=DIRECTION('ref_axis',(0.,0.241015854951078,0.970521178368716)) ;
#10314=DIRECTION('',(-1.,0.,0.)) ;
#10315=DIRECTION('',(0.,0.241015854951078,0.970521178368716)) ;
#10316=DIRECTION('center_axis',(-1.,0.,0.)) ;
#10317=DIRECTION('ref_axis',(0.,-0.766044443118978,0.642787609686539)) ;
#10318=DIRECTION('',(0.,-0.913924816918963,-0.405883516565577)) ;
#10319=DIRECTION('center_axis',(0.,0.405883516565577,-0.913924816918963)) ;
#10320=DIRECTION('ref_axis',(0.,-0.913924816918963,-0.405883516565577)) ;
#10321=DIRECTION('center_axis',(0.,-0.997628744921148,0.0688250485437987)) ;
#10322=DIRECTION('ref_axis',(0.,0.0688250485437987,0.997628744921147)) ;
#10323=DIRECTION('',(-1.,0.,0.)) ;
#10324=DIRECTION('',(0.,0.0688250485437987,0.997628744921147)) ;
#10325=DIRECTION('center_axis',(-1.,0.,0.)) ;
#10326=DIRECTION('ref_axis',(0.,-0.866025403784439,0.5)) ;
#10327=DIRECTION('',(0.,-0.8295593123754,-0.5584186129162)) ;
#10328=DIRECTION('center_axis',(0.,0.5584186129162,-0.8295593123754)) ;
#10329=DIRECTION('ref_axis',(0.,-0.8295593123754,-0.5584186129162)) ;
#10330=DIRECTION('center_axis',(0.,-0.994423866883653,-0.10545697213633)) ;
#10331=DIRECTION('ref_axis',(0.,-0.10545697213633,0.994423866883653)) ;
#10332=DIRECTION('',(-1.,0.,0.)) ;
#10333=DIRECTION('',(0.,-0.10545697213633,0.994423866883653)) ;
#10334=DIRECTION('center_axis',(-1.,0.,0.)) ;
#10335=DIRECTION('ref_axis',(0.,-0.939692620785909,0.342020143325668)) ;
#10336=DIRECTION('',(0.,-0.719988067902577,-0.693986442286818)) ;
#10337=DIRECTION('center_axis',(0.,0.693986442286818,-0.719988067902577)) ;
#10338=DIRECTION('ref_axis',(0.,-0.719988067902577,-0.693986442286818)) ;
#10339=DIRECTION('center_axis',(0.,-0.961003922853655,-0.276534736081899)) ;
#10340=DIRECTION('ref_axis',(0.,-0.276534736081899,0.961003922853655)) ;
#10341=DIRECTION('',(-1.,0.,0.)) ;
#10342=DIRECTION('',(0.,-0.276534736081899,0.961003922853655)) ;
#10343=DIRECTION('center_axis',(-1.,0.,0.)) ;
#10344=DIRECTION('ref_axis',(0.,-0.984807753012208,0.17364817766693)) ;
#10345=DIRECTION('',(0.,-0.588540350318076,-0.808467844782634)) ;
#10346=DIRECTION('center_axis',(0.,0.808467844782634,-0.588540350318076)) ;
#10347=DIRECTION('ref_axis',(0.,-0.588540350318076,-0.808467844782634)) ;
#10348=DIRECTION('center_axis',(0.,-0.898384360919199,-0.439210132004947)) ;
#10349=DIRECTION('ref_axis',(0.,-0.439210132004947,0.898384360919199)) ;
#10350=DIRECTION('',(-1.,0.,0.)) ;
#10351=DIRECTION('',(0.,-0.439210132004947,0.898384360919199)) ;
#10352=DIRECTION('center_axis',(-1.,0.,0.)) ;
#10353=DIRECTION('ref_axis',(0.,-1.,-1.83697019872103E-16)) ;
#10354=DIRECTION('',(0.,-0.439210132004947,-0.898384360919199)) ;
#10355=DIRECTION('center_axis',(0.,0.898384360919199,-0.439210132004947)) ;
#10356=DIRECTION('ref_axis',(0.,-0.439210132004947,-0.898384360919199)) ;
#10357=DIRECTION('center_axis',(0.,-0.808467844782634,-0.588540350318076)) ;
#10358=DIRECTION('ref_axis',(0.,-0.588540350318076,0.808467844782634)) ;
#10359=DIRECTION('',(-1.,0.,0.)) ;
#10360=DIRECTION('',(0.,-0.588540350318076,0.808467844782634)) ;
#10361=DIRECTION('center_axis',(-1.,0.,0.)) ;
#10362=DIRECTION('ref_axis',(0.,-0.984807753012208,-0.17364817766693)) ;
#10363=DIRECTION('',(0.,-0.276534736081898,-0.961003922853656)) ;
#10364=DIRECTION('center_axis',(0.,0.961003922853656,-0.276534736081898)) ;
#10365=DIRECTION('ref_axis',(0.,-0.276534736081898,-0.961003922853656)) ;
#10366=DIRECTION('center_axis',(0.,-0.693986442286817,-0.719988067902578)) ;
#10367=DIRECTION('ref_axis',(0.,-0.719988067902578,0.693986442286817)) ;
#10368=DIRECTION('',(-1.,0.,0.)) ;
#10369=DIRECTION('',(0.,-0.719988067902578,0.693986442286817)) ;
#10370=DIRECTION('center_axis',(-1.,0.,0.)) ;
#10371=DIRECTION('ref_axis',(0.,-0.939692620785908,-0.342020143325669)) ;
#10372=DIRECTION('',(0.,-0.105456972136329,-0.994423866883653)) ;
#10373=DIRECTION('center_axis',(0.,0.994423866883653,-0.105456972136329)) ;
#10374=DIRECTION('ref_axis',(0.,-0.105456972136329,-0.994423866883653)) ;
#10375=DIRECTION('center_axis',(0.,-0.5584186129162,-0.8295593123754)) ;
#10376=DIRECTION('ref_axis',(0.,-0.8295593123754,0.5584186129162)) ;
#10377=DIRECTION('',(-1.,0.,0.)) ;
#10378=DIRECTION('',(0.,-0.8295593123754,0.5584186129162)) ;
#10379=DIRECTION('center_axis',(-1.,0.,0.)) ;
#10380=DIRECTION('ref_axis',(0.,-0.866025403784438,-0.5)) ;
#10381=DIRECTION('',(0.,0.0688250485437991,-0.997628744921147)) ;
#10382=DIRECTION('center_axis',(0.,0.997628744921147,0.0688250485437991)) ;
#10383=DIRECTION('ref_axis',(0.,0.0688250485437991,-0.997628744921147)) ;
#10384=DIRECTION('center_axis',(0.,-0.405883516565577,-0.913924816918964)) ;
#10385=DIRECTION('ref_axis',(0.,-0.913924816918964,0.405883516565577)) ;
#10386=DIRECTION('',(-1.,0.,0.)) ;
#10387=DIRECTION('',(0.,-0.913924816918964,0.405883516565577)) ;
#10388=DIRECTION('center_axis',(-1.,0.,0.)) ;
#10389=DIRECTION('ref_axis',(0.,-0.766044443118978,-0.642787609686539)) ;
#10390=DIRECTION('',(0.,0.241015854951079,-0.970521178368716)) ;
#10391=DIRECTION('center_axis',(0.,0.970521178368716,0.241015854951079)) ;
#10392=DIRECTION('ref_axis',(0.,0.241015854951079,-0.970521178368716)) ;
#10393=DIRECTION('center_axis',(0.,-0.241015854951079,-0.970521178368716)) ;
#10394=DIRECTION('ref_axis',(0.,-0.970521178368716,0.241015854951079)) ;
#10395=DIRECTION('',(-1.,0.,0.)) ;
#10396=DIRECTION('',(0.,-0.970521178368716,0.241015854951079)) ;
#10397=DIRECTION('center_axis',(-1.,0.,0.)) ;
#10398=DIRECTION('ref_axis',(0.,-0.642787609686539,-0.766044443118978)) ;
#10399=DIRECTION('',(0.,0.405883516565577,-0.913924816918963)) ;
#10400=DIRECTION('center_axis',(0.,0.913924816918963,0.405883516565577)) ;
#10401=DIRECTION('ref_axis',(0.,0.405883516565577,-0.913924816918963)) ;
#10402=DIRECTION('center_axis',(0.,-0.0688250485437983,-0.997628744921147)) ;
#10403=DIRECTION('ref_axis',(0.,-0.997628744921147,0.0688250485437983)) ;
#10404=DIRECTION('',(-1.,0.,0.)) ;
#10405=DIRECTION('',(0.,-0.997628744921147,0.0688250485437983)) ;
#10406=DIRECTION('center_axis',(-1.,0.,0.)) ;
#10407=DIRECTION('ref_axis',(0.,-0.5,-0.866025403784439)) ;
#10408=DIRECTION('',(0.,0.558418612916201,-0.8295593123754)) ;
#10409=DIRECTION('center_axis',(0.,0.8295593123754,0.558418612916201)) ;
#10410=DIRECTION('ref_axis',(0.,0.558418612916201,-0.8295593123754)) ;
#10411=DIRECTION('center_axis',(0.,0.10545697213633,-0.994423866883653)) ;
#10412=DIRECTION('ref_axis',(0.,-0.994423866883653,-0.10545697213633)) ;
#10413=DIRECTION('',(-1.,0.,0.)) ;
#10414=DIRECTION('',(0.,-0.994423866883653,-0.10545697213633)) ;
#10415=DIRECTION('center_axis',(-1.,0.,0.)) ;
#10416=DIRECTION('ref_axis',(0.,-0.342020143325669,-0.939692620785909)) ;
#10417=DIRECTION('',(0.,0.693986442286818,-0.719988067902577)) ;
#10418=DIRECTION('center_axis',(0.,0.719988067902577,0.693986442286818)) ;
#10419=DIRECTION('ref_axis',(0.,0.693986442286818,-0.719988067902577)) ;
#10420=DIRECTION('center_axis',(0.,0.276534736081899,-0.961003922853656)) ;
#10421=DIRECTION('ref_axis',(0.,-0.961003922853656,-0.276534736081899)) ;
#10422=DIRECTION('',(-1.,0.,0.)) ;
#10423=DIRECTION('',(0.,-0.961003922853655,-0.276534736081899)) ;
#10424=DIRECTION('center_axis',(-1.,0.,0.)) ;
#10425=DIRECTION('ref_axis',(0.,-0.17364817766693,-0.984807753012208)) ;
#10426=DIRECTION('',(0.,0.808467844782634,-0.588540350318076)) ;
#10427=DIRECTION('center_axis',(0.,0.588540350318076,0.808467844782634)) ;
#10428=DIRECTION('ref_axis',(0.,0.808467844782634,-0.588540350318076)) ;
#10429=DIRECTION('center_axis',(0.,0.439210132004947,-0.898384360919199)) ;
#10430=DIRECTION('ref_axis',(0.,-0.898384360919199,-0.439210132004947)) ;
#10431=DIRECTION('',(-1.,0.,0.)) ;
#10432=DIRECTION('',(0.,-0.898384360919199,-0.439210132004947)) ;
#10433=DIRECTION('center_axis',(-1.,0.,0.)) ;
#10434=DIRECTION('ref_axis',(0.,1.22464679914735E-16,-1.)) ;
#10435=DIRECTION('',(0.,0.898384360919199,-0.439210132004947)) ;
#10436=DIRECTION('center_axis',(0.,0.439210132004947,0.898384360919199)) ;
#10437=DIRECTION('ref_axis',(0.,0.898384360919199,-0.439210132004947)) ;
#10438=DIRECTION('center_axis',(0.,0.588540350318076,-0.808467844782634)) ;
#10439=DIRECTION('ref_axis',(0.,-0.808467844782633,-0.588540350318076)) ;
#10440=DIRECTION('',(-1.,0.,0.)) ;
#10441=DIRECTION('',(0.,-0.808467844782633,-0.588540350318076)) ;
#10442=DIRECTION('center_axis',(-1.,0.,0.)) ;
#10443=DIRECTION('ref_axis',(0.,0.173648177666931,-0.984807753012208)) ;
#10444=DIRECTION('',(0.,0.961003922853656,-0.276534736081898)) ;
#10445=DIRECTION('center_axis',(0.,0.276534736081898,0.961003922853656)) ;
#10446=DIRECTION('ref_axis',(0.,0.961003922853656,-0.276534736081898)) ;
#10447=DIRECTION('center_axis',(0.,0.719988067902577,-0.693986442286817)) ;
#10448=DIRECTION('ref_axis',(0.,-0.693986442286817,-0.719988067902577)) ;
#10449=DIRECTION('',(-1.,0.,0.)) ;
#10450=DIRECTION('',(0.,-0.693986442286817,-0.719988067902577)) ;
#10451=DIRECTION('center_axis',(-1.,0.,0.)) ;
#10452=DIRECTION('ref_axis',(0.,0.342020143325669,-0.939692620785908)) ;
#10453=DIRECTION('',(0.,0.994423866883653,-0.10545697213633)) ;
#10454=DIRECTION('center_axis',(0.,0.10545697213633,0.994423866883653)) ;
#10455=DIRECTION('ref_axis',(0.,0.994423866883653,-0.10545697213633)) ;
#10456=DIRECTION('center_axis',(0.,0.8295593123754,-0.558418612916201)) ;
#10457=DIRECTION('ref_axis',(0.,-0.558418612916201,-0.8295593123754)) ;
#10458=DIRECTION('',(-1.,0.,0.)) ;
#10459=DIRECTION('',(0.,-0.558418612916201,-0.8295593123754)) ;
#10460=DIRECTION('center_axis',(-1.,0.,0.)) ;
#10461=DIRECTION('ref_axis',(0.,0.5,-0.866025403784439)) ;
#10462=DIRECTION('',(0.,0.997628744921147,0.0688250485437986)) ;
#10463=DIRECTION('center_axis',(0.,-0.0688250485437986,0.997628744921148)) ;
#10464=DIRECTION('ref_axis',(0.,0.997628744921147,0.0688250485437986)) ;
#10465=DIRECTION('center_axis',(0.,0.913924816918964,-0.405883516565577)) ;
#10466=DIRECTION('ref_axis',(0.,-0.405883516565577,-0.913924816918964)) ;
#10467=DIRECTION('',(-1.,0.,0.)) ;
#10468=DIRECTION('',(0.,-0.405883516565577,-0.913924816918964)) ;
#10469=DIRECTION('center_axis',(-1.,0.,0.)) ;
#10470=DIRECTION('ref_axis',(0.,0.642787609686539,-0.766044443118978)) ;
#10471=DIRECTION('',(0.,0.970521178368716,0.241015854951079)) ;
#10472=DIRECTION('center_axis',(0.,-0.241015854951079,0.970521178368716)) ;
#10473=DIRECTION('ref_axis',(0.,0.970521178368716,0.241015854951079)) ;
#10474=DIRECTION('center_axis',(0.,0.970521178368716,-0.241015854951079)) ;
#10475=DIRECTION('ref_axis',(0.,-0.241015854951079,-0.970521178368716)) ;
#10476=DIRECTION('',(-1.,0.,0.)) ;
#10477=DIRECTION('',(0.,-0.241015854951079,-0.970521178368716)) ;
#10478=DIRECTION('center_axis',(-1.,0.,0.)) ;
#10479=DIRECTION('ref_axis',(0.,0.766044443118978,-0.642787609686539)) ;
#10480=DIRECTION('',(0.,0.913924816918963,0.405883516565577)) ;
#10481=DIRECTION('center_axis',(0.,-0.405883516565577,0.913924816918964)) ;
#10482=DIRECTION('ref_axis',(0.,0.913924816918963,0.405883516565577)) ;
#10483=DIRECTION('center_axis',(0.,0.997628744921147,-0.0688250485437984)) ;
#10484=DIRECTION('ref_axis',(0.,-0.0688250485437984,-0.997628744921147)) ;
#10485=DIRECTION('',(-1.,0.,0.)) ;
#10486=DIRECTION('',(0.,-0.0688250485437984,-0.997628744921147)) ;
#10487=DIRECTION('center_axis',(-1.,0.,0.)) ;
#10488=DIRECTION('ref_axis',(0.,0.866025403784439,-0.5)) ;
#10489=DIRECTION('',(0.,0.8295593123754,0.558418612916201)) ;
#10490=DIRECTION('center_axis',(0.,-0.558418612916201,0.8295593123754)) ;
#10491=DIRECTION('ref_axis',(0.,0.8295593123754,0.558418612916201)) ;
#10492=DIRECTION('center_axis',(0.,0.994423866883653,0.10545697213633)) ;
#10493=DIRECTION('ref_axis',(0.,0.10545697213633,-0.994423866883653)) ;
#10494=DIRECTION('',(-1.,0.,0.)) ;
#10495=DIRECTION('',(0.,0.10545697213633,-0.994423866883653)) ;
#10496=DIRECTION('center_axis',(-1.,0.,0.)) ;
#10497=DIRECTION('ref_axis',(0.,0.939692620785908,-0.342020143325669)) ;
#10498=DIRECTION('',(0.,0.719988067902577,0.693986442286817)) ;
#10499=DIRECTION('center_axis',(0.,-0.693986442286817,0.719988067902577)) ;
#10500=DIRECTION('ref_axis',(0.,0.719988067902577,0.693986442286817)) ;
#10501=DIRECTION('center_axis',(0.,0.961003922853656,0.276534736081898)) ;
#10502=DIRECTION('ref_axis',(0.,0.276534736081898,-0.961003922853656)) ;
#10503=DIRECTION('',(-1.,0.,0.)) ;
#10504=DIRECTION('',(0.,0.276534736081898,-0.961003922853656)) ;
#10505=DIRECTION('center_axis',(-1.,0.,0.)) ;
#10506=DIRECTION('ref_axis',(0.,0.984807753012208,-0.17364817766693)) ;
#10507=DIRECTION('',(0.,0.588540350318076,0.808467844782634)) ;
#10508=DIRECTION('center_axis',(0.,-0.808467844782634,0.588540350318076)) ;
#10509=DIRECTION('ref_axis',(0.,0.588540350318076,0.808467844782634)) ;
#10510=DIRECTION('center_axis',(0.,0.898384360919199,0.439210132004947)) ;
#10511=DIRECTION('ref_axis',(0.,0.439210132004947,-0.898384360919199)) ;
#10512=DIRECTION('',(-1.,0.,0.)) ;
#10513=DIRECTION('',(0.,0.439210132004947,-0.898384360919199)) ;
#10514=DIRECTION('center_axis',(-1.,0.,0.)) ;
#10515=DIRECTION('ref_axis',(0.,1.,6.12323399573677E-17)) ;
#10516=DIRECTION('',(0.,0.439210132004947,0.898384360919199)) ;
#10517=DIRECTION('center_axis',(0.,-0.898384360919199,0.439210132004947)) ;
#10518=DIRECTION('ref_axis',(0.,0.439210132004947,0.898384360919199)) ;
#10519=DIRECTION('center_axis',(0.,0.808467844782634,0.588540350318076)) ;
#10520=DIRECTION('ref_axis',(0.,0.588540350318076,-0.808467844782634)) ;
#10521=DIRECTION('',(-1.,0.,0.)) ;
#10522=DIRECTION('',(0.,0.588540350318076,-0.808467844782634)) ;
#10523=DIRECTION('center_axis',(-1.,0.,0.)) ;
#10524=DIRECTION('ref_axis',(0.,0.984807753012208,0.17364817766693)) ;
#10525=DIRECTION('',(0.,0.276534736081898,0.961003922853656)) ;
#10526=DIRECTION('center_axis',(0.,-0.961003922853656,0.276534736081898)) ;
#10527=DIRECTION('ref_axis',(0.,0.276534736081898,0.961003922853656)) ;
#10528=DIRECTION('center_axis',(0.,0.693986442286817,0.719988067902577)) ;
#10529=DIRECTION('ref_axis',(0.,0.719988067902577,-0.693986442286817)) ;
#10530=DIRECTION('',(-1.,0.,0.)) ;
#10531=DIRECTION('',(0.,0.719988067902577,-0.693986442286817)) ;
#10532=DIRECTION('center_axis',(-1.,0.,0.)) ;
#10533=DIRECTION('ref_axis',(0.,0.939692620785908,0.342020143325669)) ;
#10534=DIRECTION('',(0.,0.10545697213633,0.994423866883653)) ;
#10535=DIRECTION('center_axis',(0.,-0.994423866883653,0.10545697213633)) ;
#10536=DIRECTION('ref_axis',(0.,0.10545697213633,0.994423866883653)) ;
#10537=DIRECTION('center_axis',(0.,0.5584186129162,0.8295593123754)) ;
#10538=DIRECTION('ref_axis',(0.,0.8295593123754,-0.5584186129162)) ;
#10539=DIRECTION('',(-1.,0.,0.)) ;
#10540=DIRECTION('',(0.,0.8295593123754,-0.5584186129162)) ;
#10541=DIRECTION('center_axis',(-1.,0.,0.)) ;
#10542=DIRECTION('ref_axis',(0.,0.866025403784439,0.5)) ;
#10543=DIRECTION('',(0.,-0.0688250485437987,0.997628744921147)) ;
#10544=DIRECTION('center_axis',(0.,-0.997628744921148,-0.0688250485437987)) ;
#10545=DIRECTION('ref_axis',(0.,-0.0688250485437987,0.997628744921147)) ;
#10546=DIRECTION('center_axis',(0.,0.405883516565577,0.913924816918964)) ;
#10547=DIRECTION('ref_axis',(0.,0.913924816918963,-0.405883516565577)) ;
#10548=DIRECTION('',(-1.,0.,0.)) ;
#10549=DIRECTION('',(0.,0.913924816918963,-0.405883516565577)) ;
#10550=DIRECTION('center_axis',(-1.,0.,0.)) ;
#10551=DIRECTION('ref_axis',(0.,0.766044443118978,0.642787609686539)) ;
#10552=DIRECTION('',(0.,-0.241015854951079,0.970521178368716)) ;
#10553=DIRECTION('center_axis',(0.,-0.970521178368716,-0.241015854951079)) ;
#10554=DIRECTION('ref_axis',(0.,-0.241015854951079,0.970521178368716)) ;
#10555=DIRECTION('center_axis',(0.,0.241015854951079,0.970521178368716)) ;
#10556=DIRECTION('ref_axis',(0.,0.970521178368716,-0.241015854951079)) ;
#10557=DIRECTION('',(-1.,0.,0.)) ;
#10558=DIRECTION('',(0.,0.970521178368716,-0.241015854951079)) ;
#10559=DIRECTION('center_axis',(-1.,0.,0.)) ;
#10560=DIRECTION('ref_axis',(0.,0.642787609686539,0.766044443118978)) ;
#10561=DIRECTION('',(0.,-0.405883516565577,0.913924816918963)) ;
#10562=DIRECTION('center_axis',(0.,-0.913924816918963,-0.405883516565577)) ;
#10563=DIRECTION('ref_axis',(0.,-0.405883516565577,0.913924816918963)) ;
#10564=DIRECTION('center_axis',(0.,0.0688250485437986,0.997628744921148)) ;
#10565=DIRECTION('ref_axis',(0.,0.997628744921147,-0.0688250485437986)) ;
#10566=DIRECTION('',(-1.,0.,0.)) ;
#10567=DIRECTION('',(0.,0.997628744921147,-0.0688250485437986)) ;
#10568=DIRECTION('center_axis',(-1.,0.,0.)) ;
#10569=DIRECTION('ref_axis',(0.,0.5,0.866025403784439)) ;
#10570=DIRECTION('',(0.,-0.558418612916201,0.8295593123754)) ;
#10571=DIRECTION('center_axis',(0.,-0.8295593123754,-0.558418612916201)) ;
#10572=DIRECTION('ref_axis',(0.,-0.558418612916201,0.8295593123754)) ;
#10573=DIRECTION('center_axis',(0.,-0.10545697213633,0.994423866883653)) ;
#10574=DIRECTION('ref_axis',(0.,0.994423866883653,0.10545697213633)) ;
#10575=DIRECTION('',(-1.,0.,0.)) ;
#10576=DIRECTION('',(0.,0.994423866883653,0.10545697213633)) ;
#10577=DIRECTION('center_axis',(-1.,0.,0.)) ;
#10578=DIRECTION('ref_axis',(0.,0.342020143325669,0.939692620785908)) ;
#10579=DIRECTION('',(0.,-0.693986442286817,0.719988067902577)) ;
#10580=DIRECTION('center_axis',(0.,-0.719988067902577,-0.693986442286817)) ;
#10581=DIRECTION('ref_axis',(0.,-0.693986442286817,0.719988067902577)) ;
#10582=DIRECTION('center_axis',(0.,-0.276534736081898,0.961003922853656)) ;
#10583=DIRECTION('ref_axis',(0.,0.961003922853656,0.276534736081898)) ;
#10584=DIRECTION('',(-1.,0.,0.)) ;
#10585=DIRECTION('',(0.,0.961003922853656,0.276534736081898)) ;
#10586=DIRECTION('center_axis',(-1.,0.,0.)) ;
#10587=DIRECTION('ref_axis',(0.,0.17364817766693,0.984807753012208)) ;
#10588=DIRECTION('',(0.,-0.808467844782634,0.588540350318076)) ;
#10589=DIRECTION('center_axis',(0.,-0.588540350318076,-0.808467844782634)) ;
#10590=DIRECTION('ref_axis',(0.,-0.808467844782634,0.588540350318076)) ;
#10591=DIRECTION('center_axis',(0.,-0.439210132004947,0.898384360919199)) ;
#10592=DIRECTION('ref_axis',(0.,0.898384360919199,0.439210132004947)) ;
#10593=DIRECTION('',(-1.,0.,0.)) ;
#10594=DIRECTION('',(0.,0.898384360919199,0.439210132004947)) ;
#10595=DIRECTION('center_axis',(-1.,0.,0.)) ;
#10596=DIRECTION('ref_axis',(0.,0.,1.)) ;
#10597=DIRECTION('',(0.,-0.898384360919199,0.439210132004947)) ;
#10598=DIRECTION('center_axis',(0.,-0.439210132004947,-0.898384360919199)) ;
#10599=DIRECTION('ref_axis',(0.,-0.898384360919199,0.439210132004947)) ;
#10600=DIRECTION('center_axis',(1.,0.,0.)) ;
#10601=DIRECTION('ref_axis',(0.,0.,-1.)) ;
#10602=DIRECTION('center_axis',(0.,-1.,0.)) ;
#10603=DIRECTION('ref_axis',(0.,0.,1.)) ;
#10604=DIRECTION('center_axis',(-1.,0.,0.)) ;
#10605=DIRECTION('ref_axis',(0.,0.,-1.)) ;
#10606=DIRECTION('center_axis',(-1.,0.,0.)) ;
#10607=DIRECTION('ref_axis',(0.,0.,-1.)) ;
#10608=DIRECTION('',(-0.707106781186548,-8.65956056235494E-17,0.707106781186548)) ;
#10609=DIRECTION('center_axis',(1.,0.,0.)) ;
#10610=DIRECTION('ref_axis',(0.,0.,-1.)) ;
#10611=DIRECTION('center_axis',(-1.,0.,0.)) ;
#10612=DIRECTION('ref_axis',(0.,1.,0.)) ;
#10613=DIRECTION('center_axis',(1.,0.,0.)) ;
#10614=DIRECTION('ref_axis',(0.,1.,0.)) ;
#10615=DIRECTION('center_axis',(1.,0.,0.)) ;
#10616=DIRECTION('ref_axis',(0.,0.,-1.)) ;
#10617=DIRECTION('center_axis',(1.,0.,0.)) ;
#10618=DIRECTION('ref_axis',(0.,0.,-1.)) ;
#10619=DIRECTION('center_axis',(1.,0.,0.)) ;
#10620=DIRECTION('ref_axis',(0.,0.,-1.)) ;
#10621=DIRECTION('center_axis',(1.,0.,0.)) ;
#10622=DIRECTION('ref_axis',(0.,0.,-1.)) ;
#10623=DIRECTION('center_axis',(1.,0.,0.)) ;
#10624=DIRECTION('ref_axis',(0.,0.,-1.)) ;
#10625=DIRECTION('',(0.707106781186542,-0.707106781186553,-8.659560562355E-17)) ;
#10626=DIRECTION('center_axis',(1.,0.,0.)) ;
#10627=DIRECTION('ref_axis',(0.,0.,-1.)) ;
#10628=DIRECTION('center_axis',(1.,0.,0.)) ;
#10629=DIRECTION('ref_axis',(0.,1.,0.)) ;
#10630=DIRECTION('',(1.,0.,0.)) ;
#10631=DIRECTION('',(-1.,0.,0.)) ;
#10632=DIRECTION('center_axis',(1.,0.,0.)) ;
#10633=DIRECTION('ref_axis',(0.,1.,0.)) ;
#10634=DIRECTION('center_axis',(1.,0.,0.)) ;
#10635=DIRECTION('ref_axis',(0.,1.,0.)) ;
#10636=DIRECTION('',(-1.,0.,0.)) ;
#10637=DIRECTION('center_axis',(1.,0.,0.)) ;
#10638=DIRECTION('ref_axis',(0.,1.,0.)) ;
#10639=DIRECTION('',(1.,0.,0.)) ;
#10640=DIRECTION('center_axis',(1.,0.,0.)) ;
#10641=DIRECTION('ref_axis',(0.,1.,0.)) ;
#10642=DIRECTION('',(1.,0.,0.)) ;
#10643=DIRECTION('',(-1.,0.,0.)) ;
#10644=DIRECTION('center_axis',(1.,0.,0.)) ;
#10645=DIRECTION('ref_axis',(0.,1.,0.)) ;
#10646=DIRECTION('center_axis',(1.,0.,0.)) ;
#10647=DIRECTION('ref_axis',(0.,1.,0.)) ;
#10648=DIRECTION('',(-1.,0.,0.)) ;
#10649=DIRECTION('center_axis',(1.,0.,0.)) ;
#10650=DIRECTION('ref_axis',(0.,1.,0.)) ;
#10651=DIRECTION('',(1.,0.,0.)) ;
#10652=DIRECTION('center_axis',(1.,0.,0.)) ;
#10653=DIRECTION('ref_axis',(0.,1.,0.)) ;
#10654=DIRECTION('',(1.,0.,0.)) ;
#10655=DIRECTION('',(-1.,0.,0.)) ;
#10656=DIRECTION('center_axis',(1.,0.,0.)) ;
#10657=DIRECTION('ref_axis',(0.,1.,0.)) ;
#10658=DIRECTION('center_axis',(1.,0.,0.)) ;
#10659=DIRECTION('ref_axis',(0.,1.,0.)) ;
#10660=DIRECTION('',(-1.,0.,0.)) ;
#10661=DIRECTION('center_axis',(1.,0.,0.)) ;
#10662=DIRECTION('ref_axis',(0.,1.,0.)) ;
#10663=DIRECTION('',(1.,0.,0.)) ;
#10664=DIRECTION('center_axis',(0.,-0.86602540378444,0.499999999999998)) ;
#10665=DIRECTION('ref_axis',(0.,0.499999999999998,0.86602540378444)) ;
#10666=DIRECTION('',(0.,0.499999999999998,0.86602540378444)) ;
#10667=DIRECTION('',(-1.,0.,0.)) ;
#10668=DIRECTION('',(0.,0.499999999999998,0.86602540378444)) ;
#10669=DIRECTION('',(-1.,0.,0.)) ;
#10670=DIRECTION('center_axis',(0.,-0.86602540378444,-0.499999999999998)) ;
#10671=DIRECTION('ref_axis',(0.,-0.499999999999998,0.86602540378444)) ;
#10672=DIRECTION('',(0.,-0.499999999999998,0.86602540378444)) ;
#10673=DIRECTION('',(-1.,0.,0.)) ;
#10674=DIRECTION('',(0.,-0.499999999999998,0.86602540378444)) ;
#10675=DIRECTION('center_axis',(0.,0.,-1.)) ;
#10676=DIRECTION('ref_axis',(0.,-1.,0.)) ;
#10677=DIRECTION('',(0.,-1.,0.)) ;
#10678=DIRECTION('',(-1.,0.,0.)) ;
#10679=DIRECTION('',(0.,-1.,0.)) ;
#10680=DIRECTION('center_axis',(1.,0.,0.)) ;
#10681=DIRECTION('ref_axis',(0.,0.,-1.)) ;
#10682=DIRECTION('center_axis',(1.,0.,0.)) ;
#10683=DIRECTION('ref_axis',(0.,0.,-1.)) ;
#10684=DIRECTION('center_axis',(1.,0.,0.)) ;
#10685=DIRECTION('ref_axis',(0.,0.,-1.)) ;
#10686=DIRECTION('',(0.,-0.499999999999998,-0.86602540378444)) ;
#10687=DIRECTION('center_axis',(1.,0.,0.)) ;
#10688=DIRECTION('ref_axis',(0.,0.,-1.)) ;
#10689=DIRECTION('center_axis',(1.,0.,0.)) ;
#10690=DIRECTION('ref_axis',(0.,0.,-1.)) ;
#10691=DIRECTION('',(0.,0.499999999999998,-0.86602540378444)) ;
#10692=DIRECTION('center_axis',(1.,0.,0.)) ;
#10693=DIRECTION('ref_axis',(0.,0.,-1.)) ;
#10694=DIRECTION('',(0.,1.,0.)) ;
#10695=DIRECTION('center_axis',(1.,0.,0.)) ;
#10696=DIRECTION('ref_axis',(0.,0.,-1.)) ;
#10697=DIRECTION('',(0.,0.499999999999998,-0.86602540378444)) ;
#10698=DIRECTION('center_axis',(1.,0.,0.)) ;
#10699=DIRECTION('ref_axis',(0.,0.,-1.)) ;
#10700=DIRECTION('center_axis',(1.,0.,0.)) ;
#10701=DIRECTION('ref_axis',(0.,0.,-1.)) ;
#10702=DIRECTION('',(0.,-0.499999999999998,-0.86602540378444)) ;
#10703=DIRECTION('center_axis',(1.,0.,0.)) ;
#10704=DIRECTION('ref_axis',(0.,0.,-1.)) ;
#10705=DIRECTION('center_axis',(1.,0.,0.)) ;
#10706=DIRECTION('ref_axis',(0.,0.,-1.)) ;
#10707=DIRECTION('center_axis',(1.,0.,0.)) ;
#10708=DIRECTION('ref_axis',(0.,0.,-1.)) ;
#10709=DIRECTION('center_axis',(1.,0.,0.)) ;
#10710=DIRECTION('ref_axis',(0.,0.,-1.)) ;
#10711=DIRECTION('center_axis',(1.,0.,0.)) ;
#10712=DIRECTION('ref_axis',(0.,0.,-1.)) ;
#10713=DIRECTION('center_axis',(1.,0.,0.)) ;
#10714=DIRECTION('ref_axis',(0.,0.,-1.)) ;
#10715=DIRECTION('center_axis',(1.,0.,0.)) ;
#10716=DIRECTION('ref_axis',(0.,0.,-1.)) ;
#10717=DIRECTION('center_axis',(1.,0.,0.)) ;
#10718=DIRECTION('ref_axis',(0.,0.,-1.)) ;
#10719=DIRECTION('',(0.,1.,0.)) ;
#10720=DIRECTION('center_axis',(1.,0.,0.)) ;
#10721=DIRECTION('ref_axis',(0.,0.,-1.)) ;
#10722=DIRECTION('center_axis',(1.,0.,0.)) ;
#10723=DIRECTION('ref_axis',(0.,1.,0.)) ;
#10724=DIRECTION('',(0.515038074910055,-0.857167300702112,-1.04972719113862E-16)) ;
#10725=DIRECTION('center_axis',(0.,0.86602540378444,0.499999999999998)) ;
#10726=DIRECTION('ref_axis',(0.,0.499999999999998,-0.86602540378444)) ;
#10727=DIRECTION('',(-1.,0.,0.)) ;
#10728=DIRECTION('',(-1.,0.,0.)) ;
#10729=DIRECTION('center_axis',(0.,0.,1.)) ;
#10730=DIRECTION('ref_axis',(0.,1.,0.)) ;
#10731=DIRECTION('center_axis',(0.,0.86602540378444,-0.499999999999998)) ;
#10732=DIRECTION('ref_axis',(0.,-0.499999999999998,-0.86602540378444)) ;
#13718=CARTESIAN_POINT('',(0.,0.,0.)) ;
#13719=CARTESIAN_POINT('Origin',(29.6,39.642135623731,39.642135623731)) ;
#13720=CARTESIAN_POINT('',(29.1741303078758,39.6408187757763,41.5983047332171)) ;
#13721=CARTESIAN_POINT('',(29.2758696921242,39.6403302138731,41.5978361791329)) ;
#13722=CARTESIAN_POINT('',(29.6,39.642135623731,41.596135623731)) ;
#13723=CARTESIAN_POINT('',(29.4,37.887097212946,38.7795589530206)) ;
#13724=CARTESIAN_POINT('Ctrl Pts',(29.1741303078758,39.6408187757763,41.5983047332171)) ;
#13725=CARTESIAN_POINT('Ctrl Pts',(29.178358479461,39.5668972107545,41.5988463683251)) ;
#13726=CARTESIAN_POINT('Ctrl Pts',(29.1825866510463,39.4930348242883,41.5950187173956)) ;
#13727=CARTESIAN_POINT('Ctrl Pts',(29.1868148226315,39.4196968033455,41.5866345034286)) ;
#13728=CARTESIAN_POINT('Ctrl Pts',(29.2237530942682,38.7789991201355,41.5133880973328)) ;
#13729=CARTESIAN_POINT('Ctrl Pts',(29.260691365905,38.1783218958328,41.0923771345517)) ;
#13730=CARTESIAN_POINT('Ctrl Pts',(29.2976296375417,37.8905206264674,40.5150612002977)) ;
#13731=CARTESIAN_POINT('Ctrl Pts',(29.3317530916944,37.6246507580315,39.9817386342627)) ;
#13732=CARTESIAN_POINT('Ctrl Pts',(29.3658765458472,37.6257893479619,39.3150253464114)) ;
#13733=CARTESIAN_POINT('Ctrl Pts',(29.4,37.8858801137886,38.7785081419809)) ;
#13734=CARTESIAN_POINT('',(29.4,37.8883143121033,40.5036614834013)) ;
#13735=CARTESIAN_POINT('Origin',(29.4,39.642135623731,39.642135623731)) ;
#13736=CARTESIAN_POINT('Ctrl Pts',(29.4,37.8883143121033,40.5036614834013)) ;
#13737=CARTESIAN_POINT('Ctrl Pts',(29.3630617283633,38.1739593715505,41.0851534806482)) ;
#13738=CARTESIAN_POINT('Ctrl Pts',(29.3261234567266,38.7692045105899,41.5084274781235)) ;
#13739=CARTESIAN_POINT('Ctrl Pts',(29.2891851850899,39.4085096414219,41.5850281011346)) ;
#13740=CARTESIAN_POINT('Ctrl Pts',(29.2847466874347,39.4853284582867,41.5942324214928)) ;
#13741=CARTESIAN_POINT('Ctrl Pts',(29.2803081897794,39.5627834306131,41.5984313355494)) ;
#13742=CARTESIAN_POINT('Ctrl Pts',(29.2758696921242,39.6403302138731,41.5978361791329)) ;
#13743=CARTESIAN_POINT('Origin',(29.6,39.642135623731,39.642135623731)) ;
#13744=CARTESIAN_POINT('',(28.4741303078758,39.6414297915345,41.5932509341168)) ;
#13745=CARTESIAN_POINT('',(28.5758696921242,39.6414773978913,41.5932079635623)) ;
#13746=CARTESIAN_POINT('',(29.6,39.642135623731,41.596135623731)) ;
#13747=CARTESIAN_POINT('Ctrl Pts',(28.4741303078758,39.6414297915345,41.5932509341168)) ;
#13748=CARTESIAN_POINT('Ctrl Pts',(28.4900621829741,39.3610188002016,41.5941645620992)) ;
#13749=CARTESIAN_POINT('Ctrl Pts',(28.5059940580724,39.0809590371883,41.5376795052535)) ;
#13750=CARTESIAN_POINT('Ctrl Pts',(28.5219259331707,38.8279927600939,41.4219659840985)) ;
#13751=CARTESIAN_POINT('Ctrl Pts',(28.5588642048074,38.241486965855,41.1536825930919)) ;
#13752=CARTESIAN_POINT('Ctrl Pts',(28.5958024764441,37.8006223692225,40.5670162335662)) ;
#13753=CARTESIAN_POINT('Ctrl Pts',(28.6327407480808,37.7060808628922,39.9290270322568)) ;
#13754=CARTESIAN_POINT('Ctrl Pts',(28.6696790197175,37.611539356562,39.2910378309475)) ;
#13755=CARTESIAN_POINT('Ctrl Pts',(28.7066172913542,37.8633209405341,38.6017257878545)) ;
#13756=CARTESIAN_POINT('Ctrl Pts',(28.7435555629909,38.3468275454814,38.1748867110876)) ;
#13757=CARTESIAN_POINT('Ctrl Pts',(28.7804938346277,38.8303341504287,37.7480476343208)) ;
#13758=CARTESIAN_POINT('Ctrl Pts',(28.8174321062644,39.5455657763513,37.58368152388)) ;
#13759=CARTESIAN_POINT('Ctrl Pts',(28.8543703779011,40.16689692944,37.7565991948941)) ;
#13760=CARTESIAN_POINT('Ctrl Pts',(28.8913086495378,40.7882280825286,37.9295168659081)) ;
#13761=CARTESIAN_POINT('Ctrl Pts',(28.9282469211745,41.3156587627833,38.4397183183768)) ;
#13762=CARTESIAN_POINT('Ctrl Pts',(28.9651851928112,41.5091643242028,39.0549731841945)) ;
#13763=CARTESIAN_POINT('Ctrl Pts',(29.002123464448,41.7026698856222,39.6702280500122)) ;
#13764=CARTESIAN_POINT('Ctrl Pts',(29.0390617360846,41.5622503282064,40.3905363291788)) ;
#13765=CARTESIAN_POINT('Ctrl Pts',(29.0760000077214,41.1516814784397,40.8879495440568)) ;
#13766=CARTESIAN_POINT('Ctrl Pts',(29.1087101077728,40.7881087513245,41.3284259200389)) ;
#13767=CARTESIAN_POINT('Ctrl Pts',(29.1414202078243,40.212692868176,41.5941145204462)) ;
#13768=CARTESIAN_POINT('Ctrl Pts',(29.1741303078758,39.6408187757763,41.5983047332171)) ;
#13769=CARTESIAN_POINT('Ctrl Pts',(29.2758696921242,39.6403302138731,41.5978361791329)) ;
#13770=CARTESIAN_POINT('Ctrl Pts',(29.2433699181427,40.2081468772396,41.5934782971368)) ;
#13771=CARTESIAN_POINT('Ctrl Pts',(29.2108701441612,40.7808860108025,41.3320849172391)) ;
#13772=CARTESIAN_POINT('Ctrl Pts',(29.1783703701797,41.1448464448315,40.8966231887847)) ;
#13773=CARTESIAN_POINT('Ctrl Pts',(29.141432098543,41.5585129947845,40.4016904048769)) ;
#13774=CARTESIAN_POINT('Ctrl Pts',(29.1044938269063,41.7024809720658,39.6818975885143)) ;
#13775=CARTESIAN_POINT('Ctrl Pts',(29.0675555552696,41.512330041934,39.0654838455824)) ;
#13776=CARTESIAN_POINT('Ctrl Pts',(29.0306172836329,41.3221791118021,38.4490701026506)) ;
#13777=CARTESIAN_POINT('Ctrl Pts',(28.9936790119962,40.7979092742571,37.9360354331494)) ;
#13778=CARTESIAN_POINT('Ctrl Pts',(28.9567407403594,40.1776331119795,37.7596379549628)) ;
#13779=CARTESIAN_POINT('Ctrl Pts',(28.9198024687227,39.5573569497018,37.5832404767762)) ;
#13780=CARTESIAN_POINT('Ctrl Pts',(28.882864197086,38.8410744626915,37.7434801899042)) ;
#13781=CARTESIAN_POINT('Ctrl Pts',(28.8459259254493,38.3551253306134,38.1675558119185)) ;
#13782=CARTESIAN_POINT('Ctrl Pts',(28.8089876538126,37.8691761985354,38.5916314339327)) ;
#13783=CARTESIAN_POINT('Ctrl Pts',(28.7720493821759,37.6135604213898,39.2795429648331)) ;
#13784=CARTESIAN_POINT('Ctrl Pts',(28.7351111105392,37.7045035108508,39.9180665126644)) ;
#13785=CARTESIAN_POINT('Ctrl Pts',(28.6981728389025,37.7954466003119,40.5565900604957)) ;
#13786=CARTESIAN_POINT('Ctrl Pts',(28.6612345672657,38.2329485563797,41.1457256252577)) ;
#13787=CARTESIAN_POINT('Ctrl Pts',(28.624296295629,38.817917278673,41.4173218967017)) ;
#13788=CARTESIAN_POINT('Ctrl Pts',(28.6081540944608,39.0735514048515,41.5360107648035)) ;
#13789=CARTESIAN_POINT('Ctrl Pts',(28.5920118932925,39.357347727632,41.5940581457679)) ;
#13790=CARTESIAN_POINT('Ctrl Pts',(28.5758696921242,39.6414773978913,41.5932079635623)) ;
#13791=CARTESIAN_POINT('Origin',(29.6,39.642135623731,39.642135623731)) ;
#13792=CARTESIAN_POINT('',(27.7741303078758,39.6438916302392,41.5958037900958)) ;
#13793=CARTESIAN_POINT('',(27.8758696921242,39.6438946340221,41.5959129847908)) ;
#13794=CARTESIAN_POINT('',(29.6,39.642135623731,41.596135623731)) ;
#13795=CARTESIAN_POINT('Ctrl Pts',(27.7741303078758,39.6438916302392,41.5958037900958)) ;
#13796=CARTESIAN_POINT('Ctrl Pts',(27.8017658864871,39.1590917620955,41.5914733218518)) ;
#13797=CARTESIAN_POINT('Ctrl Pts',(27.8294014650985,38.6713775391436,41.4087948654502)) ;
#13798=CARTESIAN_POINT('Ctrl Pts',(27.8570370437098,38.3164063634699,41.0819502323136)) ;
#13799=CARTESIAN_POINT('Ctrl Pts',(27.8939753153465,37.8419447321562,40.6450831049201)) ;
#13800=CARTESIAN_POINT('Ctrl Pts',(27.9309135869832,37.6046356518907,39.9506553949681)) ;
#13801=CARTESIAN_POINT('Ctrl Pts',(27.96785185862,37.7125071897698,39.3147855252961)) ;
#13802=CARTESIAN_POINT('Ctrl Pts',(28.0047901302567,37.820378727649,38.6789156556241)) ;
#13803=CARTESIAN_POINT('Ctrl Pts',(28.0417284018934,38.2734308836729,38.1016036262322)) ;
#13804=CARTESIAN_POINT('Ctrl Pts',(28.0786666735301,38.8654248336815,37.8456544202854)) ;
#13805=CARTESIAN_POINT('Ctrl Pts',(28.1156049451668,39.4574187836902,37.5897052143387)) ;
#13806=CARTESIAN_POINT('Ctrl Pts',(28.1525432168035,40.1883545276836,37.655118831837)) ;
#13807=CARTESIAN_POINT('Ctrl Pts',(28.1894814884402,40.72549377371,38.0121173915036)) ;
#13808=CARTESIAN_POINT('Ctrl Pts',(28.226419760077,41.2626330197364,38.3691159511701)) ;
#13809=CARTESIAN_POINT('Ctrl Pts',(28.2633580317137,41.6059757677957,39.0176994530047)) ;
#13810=CARTESIAN_POINT('Ctrl Pts',(28.3002963033504,41.5992261455199,39.6626190814621)) ;
#13811=CARTESIAN_POINT('Ctrl Pts',(28.3372345749871,41.5924765232442,40.3075387099194)) ;
#13812=CARTESIAN_POINT('Ctrl Pts',(28.3741728466238,41.2356345306335,40.9487944649996)) ;
#13813=CARTESIAN_POINT('Ctrl Pts',(28.4111111182605,40.6911400384056,41.294472131296)) ;
#13814=CARTESIAN_POINT('Ctrl Pts',(28.4321175147989,40.3814918954385,41.4910552904679)) ;
#13815=CARTESIAN_POINT('Ctrl Pts',(28.4531239113374,40.0111555420393,41.5920463030505)) ;
#13816=CARTESIAN_POINT('Ctrl Pts',(28.4741303078758,39.6414297915345,41.5932509341168)) ;
#13817=CARTESIAN_POINT('Ctrl Pts',(28.5758696921242,39.6414773978913,41.5932079635623)) ;
#13818=CARTESIAN_POINT('Ctrl Pts',(28.5550736216558,40.007522931787,41.5921126699976)) ;
#13819=CARTESIAN_POINT('Ctrl Pts',(28.5342775511873,40.3741217319919,41.4932634125623)) ;
#13820=CARTESIAN_POINT('Ctrl Pts',(28.5134814807189,40.6817691599538,41.3003891117333)) ;
#13821=CARTESIAN_POINT('Ctrl Pts',(28.4765432090822,41.2282168304228,40.9578030771951)) ;
#13822=CARTESIAN_POINT('Ctrl Pts',(28.4396049374455,41.5886766828423,40.3185740299928)) ;
#13823=CARTESIAN_POINT('Ctrl Pts',(28.4026666658088,41.5990767145884,39.6737018167311)) ;
#13824=CARTESIAN_POINT('Ctrl Pts',(28.365728394172,41.6094767463344,39.0288296034693)) ;
#13825=CARTESIAN_POINT('Ctrl Pts',(28.3287901225353,41.2698169574072,38.3783142241481)) ;
#13826=CARTESIAN_POINT('Ctrl Pts',(28.2918518508986,40.7347092510962,38.0182798055956)) ;
#13827=CARTESIAN_POINT('Ctrl Pts',(28.2549135792619,40.1996015447852,37.658245387043)) ;
#13828=CARTESIAN_POINT('Ctrl Pts',(28.2179753076252,39.4690459210904,37.5886919292591)) ;
#13829=CARTESIAN_POINT('Ctrl Pts',(28.1810370359885,38.8756113406825,37.841283921041)) ;
#13830=CARTESIAN_POINT('Ctrl Pts',(28.1440987643517,38.2821767602745,38.0938759128229)) ;
#13831=CARTESIAN_POINT('Ctrl Pts',(28.107160492715,37.8258632231532,38.6686133541705)) ;
#13832=CARTESIAN_POINT('Ctrl Pts',(28.0702222210783,37.7143923484776,39.3038622372428)) ;
#13833=CARTESIAN_POINT('Ctrl Pts',(28.0332839494416,37.6029214738019,39.939111120315)) ;
#13834=CARTESIAN_POINT('Ctrl Pts',(27.9963456778049,37.8362932615717,40.634871445112)) ;
#13835=CARTESIAN_POINT('Ctrl Pts',(27.9594074061682,38.3082729142534,41.0744186707252)) ;
#13836=CARTESIAN_POINT('Ctrl Pts',(27.9315615014869,38.6640746298656,41.4057712111943)) ;
#13837=CARTESIAN_POINT('Ctrl Pts',(27.9037155968056,39.1554746557266,41.5915205741414)) ;
#13838=CARTESIAN_POINT('Ctrl Pts',(27.8758696921242,39.6438946340221,41.5959129847908)) ;
#13839=CARTESIAN_POINT('Origin',(29.6,39.642135623731,39.642135623731)) ;
#13840=CARTESIAN_POINT('',(27.0741303078758,39.6413906238265,41.5989800840457)) ;
#13841=CARTESIAN_POINT('',(27.1758696921242,39.6413307831041,41.5989199275014)) ;
#13842=CARTESIAN_POINT('',(29.6,39.642135623731,41.596135623731)) ;
#13843=CARTESIAN_POINT('Ctrl Pts',(27.0741303078758,39.6413906238265,41.5989800840457)) ;
#13844=CARTESIAN_POINT('Ctrl Pts',(27.0765313183635,39.5994478954968,41.5991853621116)) ;
#13845=CARTESIAN_POINT('Ctrl Pts',(27.0789323288512,39.5575174495919,41.597952947044)) ;
#13846=CARTESIAN_POINT('Ctrl Pts',(27.0813333393388,39.5156825771046,41.5952443691905)) ;
#13847=CARTESIAN_POINT('Ctrl Pts',(27.1182716109756,38.872075274369,41.5535743369209)) ;
#13848=CARTESIAN_POINT('Ctrl Pts',(27.1552098826123,38.2510884686797,41.1625233076746)) ;
#13849=CARTESIAN_POINT('Ctrl Pts',(27.192148154249,37.9354087484862,40.60010614448)) ;
#13850=CARTESIAN_POINT('Ctrl Pts',(27.2290864258857,37.6197290282927,40.0376889812855)) ;
#13851=CARTESIAN_POINT('Ctrl Pts',(27.2660246975224,37.6093563935951,39.3039056841426)) ;
#13852=CARTESIAN_POINT('Ctrl Pts',(27.3029629691591,37.909012689149,38.7327902352957)) ;
#13853=CARTESIAN_POINT('Ctrl Pts',(27.3399012407958,38.2086689847029,38.1616747864487)) ;
#13854=CARTESIAN_POINT('Ctrl Pts',(27.3768395124325,38.8183542105085,37.7532271858975)) ;
#13855=CARTESIAN_POINT('Ctrl Pts',(27.4137777840693,39.4605265067115,37.6933815922678)) ;
#13856=CARTESIAN_POINT('Ctrl Pts',(27.450716055706,40.1026988029146,37.6335359986382)) ;
#13857=CARTESIAN_POINT('Ctrl Pts',(27.4876543273427,40.7773581695152,37.92229241193)) ;
#13858=CARTESIAN_POINT('Ctrl Pts',(27.5245925989794,41.1773851027979,38.4282026819346)) ;
#13859=CARTESIAN_POINT('Ctrl Pts',(27.5615308706161,41.5774120360807,38.9341129519391)) ;
#13860=CARTESIAN_POINT('Ctrl Pts',(27.5984691422528,41.7028065360457,39.6571770786564)) ;
#13861=CARTESIAN_POINT('Ctrl Pts',(27.6354074138895,41.4964863399443,40.2682406826823)) ;
#13862=CARTESIAN_POINT('Ctrl Pts',(27.6723456855263,41.2901661438429,40.8793042867082)) ;
#13863=CARTESIAN_POINT('Ctrl Pts',(27.709283957163,40.7521312516751,41.3783673680427)) ;
#13864=CARTESIAN_POINT('Ctrl Pts',(27.7462222287997,40.1273067144102,41.5382456362924)) ;
#13865=CARTESIAN_POINT('Ctrl Pts',(27.7555249218251,39.9699482185376,41.5785100662469)) ;
#13866=CARTESIAN_POINT('Ctrl Pts',(27.7648276148504,39.8070850417288,41.5972615130296)) ;
#13867=CARTESIAN_POINT('Ctrl Pts',(27.7741303078758,39.6438916302392,41.5958037900958)) ;
#13868=CARTESIAN_POINT('Ctrl Pts',(27.8758696921242,39.6438946340221,41.5959129847908)) ;
#13869=CARTESIAN_POINT('Ctrl Pts',(27.8667773251688,39.8033756680138,41.5973472139854)) ;
#13870=CARTESIAN_POINT('Ctrl Pts',(27.8576849582135,39.9625389747718,41.5794454958518)) ;
#13871=CARTESIAN_POINT('Ctrl Pts',(27.8485925912581,40.1165601657379,41.5409631187002)) ;
#13872=CARTESIAN_POINT('Ctrl Pts',(27.8116543196213,40.7422802469475,41.3846262146325)) ;
#13873=CARTESIAN_POINT('Ctrl Pts',(27.7747160479846,41.2831328917734,40.8886182800675)) ;
#13874=CARTESIAN_POINT('Ctrl Pts',(27.7377777763479,41.4929105802845,40.2787329662382)) ;
#13875=CARTESIAN_POINT('Ctrl Pts',(27.7008395047112,41.7026882687956,39.6688476524089)) ;
#13876=CARTESIAN_POINT('Ctrl Pts',(27.6639012330745,41.5813910009921,38.9450849593151)) ;
#13877=CARTESIAN_POINT('Ctrl Pts',(27.6269629614378,41.1842357746265,38.436917203995)) ;
#13878=CARTESIAN_POINT('Ctrl Pts',(27.5900246898011,40.7870805482609,37.9287494486749)) ;
#13879=CARTESIAN_POINT('Ctrl Pts',(27.5530864181643,40.1140673633333,37.6361766311283)) ;
#13880=CARTESIAN_POINT('Ctrl Pts',(27.5161481465276,39.4715664044991,37.6923842435544)) ;
#13881=CARTESIAN_POINT('Ctrl Pts',(27.4792098748909,38.8290654456649,37.7485918559805)) ;
#13882=CARTESIAN_POINT('Ctrl Pts',(27.4422716032542,38.2170767129241,38.1535798983792)) ;
#13883=CARTESIAN_POINT('Ctrl Pts',(27.4053333316175,37.914190642964,38.7229890613612)) ;
#13884=CARTESIAN_POINT('Ctrl Pts',(27.3683950599808,37.6113045730038,39.2923982243431)) ;
#13885=CARTESIAN_POINT('Ctrl Pts',(27.331456788344,37.6175211658244,40.0262285079083)) ;
#13886=CARTESIAN_POINT('Ctrl Pts',(27.2945185167073,37.9300105111892,40.5904245487143)) ;
#13887=CARTESIAN_POINT('Ctrl Pts',(27.2575802450706,38.2424998565541,41.1546205895204)) ;
#13888=CARTESIAN_POINT('Ctrl Pts',(27.2206419734339,38.8612619544631,41.5491823875673)) ;
#13889=CARTESIAN_POINT('Ctrl Pts',(27.1837037017972,39.5046229441121,41.5944968980767)) ;
#13890=CARTESIAN_POINT('Ctrl Pts',(27.1810923652396,39.5501050957558,41.5977003895408)) ;
#13891=CARTESIAN_POINT('Ctrl Pts',(27.1784810286819,39.5957101859526,41.599158438298)) ;
#13892=CARTESIAN_POINT('Ctrl Pts',(27.1758696921242,39.6413307831041,41.5989199275014)) ;
#13893=CARTESIAN_POINT('Origin',(29.6,39.642135623731,39.642135623731)) ;
#13894=CARTESIAN_POINT('',(26.3741303078758,39.6409887519309,41.5937162339903)) ;
#13895=CARTESIAN_POINT('',(26.4758696921242,39.6410353087582,41.5936514180137)) ;
#13896=CARTESIAN_POINT('',(29.6,39.642135623731,41.596135623731)) ;
#13897=CARTESIAN_POINT('Ctrl Pts',(26.3741303078758,39.6409887519309,41.5937162339903)) ;
#13898=CARTESIAN_POINT('Ctrl Pts',(26.3882350218765,39.3928854212053,41.5950519462106)) ;
#13899=CARTESIAN_POINT('Ctrl Pts',(26.4023397358772,39.1452370348786,41.5511579885616)) ;
#13900=CARTESIAN_POINT('Ctrl Pts',(26.416444449878,38.9165146177542,41.4598535061621)) ;
#13901=CARTESIAN_POINT('Ctrl Pts',(26.4533827215147,38.3175226231131,41.2207398472572)) ;
#13902=CARTESIAN_POINT('Ctrl Pts',(26.4903209931514,37.848333022201,40.6564645263628)) ;
#13903=CARTESIAN_POINT('Ctrl Pts',(26.5272592647882,37.7225310407902,40.0238978397713)) ;
#13904=CARTESIAN_POINT('Ctrl Pts',(26.5641975364249,37.5967290593794,39.3913311531798)) ;
#13905=CARTESIAN_POINT('Ctrl Pts',(26.6011358080616,37.8143146974699,38.6904731008914)) ;
#13906=CARTESIAN_POINT('Ctrl Pts',(26.6380740796983,38.2762382797088,38.2403693843094)) ;
#13907=CARTESIAN_POINT('Ctrl Pts',(26.675012351335,38.7381618619478,37.7902656677275)) ;
#13908=CARTESIAN_POINT('Ctrl Pts',(26.7119506229717,39.4444233883352,37.5909162868521)) ;
#13909=CARTESIAN_POINT('Ctrl Pts',(26.7488888946084,40.0735173795759,37.7330693794226)) ;
#13910=CARTESIAN_POINT('Ctrl Pts',(26.7858271662451,40.7026113708165,37.8752224719931)) ;
#13911=CARTESIAN_POINT('Ctrl Pts',(26.8227654378819,41.2545378269104,38.3588780380096)) ;
#13912=CARTESIAN_POINT('Ctrl Pts',(26.8597037095186,41.4780479210239,38.9638656323544)) ;
#13913=CARTESIAN_POINT('Ctrl Pts',(26.8966419811553,41.7015580151375,39.5688532266993)) ;
#13914=CARTESIAN_POINT('Ctrl Pts',(26.933580252792,41.5966517472707,40.2951728493725)) ;
#13915=CARTESIAN_POINT('Ctrl Pts',(26.9705185244287,41.2110847134464,40.8121881430627)) ;
#13916=CARTESIAN_POINT('Ctrl Pts',(27.0050557855777,40.8505797751371,41.2955971230993)) ;
#13917=CARTESIAN_POINT('Ctrl Pts',(27.0395930467267,40.244714503106,41.5960272680518)) ;
#13918=CARTESIAN_POINT('Ctrl Pts',(27.0741303078758,39.6413906238265,41.5989800840457)) ;
#13919=CARTESIAN_POINT('Ctrl Pts',(27.1758696921242,39.6413307831041,41.5989199275014)) ;
#13920=CARTESIAN_POINT('Ctrl Pts',(27.1415427570452,40.2410295358732,41.5957846194131)) ;
#13921=CARTESIAN_POINT('Ctrl Pts',(27.1072158219661,40.8434078942437,41.2994834007345)) ;
#13922=CARTESIAN_POINT('Ctrl Pts',(27.0728888868871,41.2044328480336,40.8210553245055)) ;
#13923=CARTESIAN_POINT('Ctrl Pts',(27.0359506152503,41.5929218809174,40.306232017453)) ;
#13924=CARTESIAN_POINT('Ctrl Pts',(26.9990123436136,41.701940065296,39.5805181803762)) ;
#13925=CARTESIAN_POINT('Ctrl Pts',(26.9620740719769,41.4818599702313,38.9742744028971)) ;
#13926=CARTESIAN_POINT('Ctrl Pts',(26.9251358003402,41.2617798751665,38.3680306254179)) ;
#13927=CARTESIAN_POINT('Ctrl Pts',(26.8881975287035,40.7126015006585,37.8812569075366)) ;
#13928=CARTESIAN_POINT('Ctrl Pts',(26.8512592570668,40.0843226884506,37.735543144862)) ;
#13929=CARTESIAN_POINT('Ctrl Pts',(26.8143209854301,39.4560438762427,37.5898293821874)) ;
#13930=CARTESIAN_POINT('Ctrl Pts',(26.7773827137934,38.748664626335,37.7851755747196)) ;
#13931=CARTESIAN_POINT('Ctrl Pts',(26.7404444421566,38.2841992294164,38.2326559221377)) ;
#13932=CARTESIAN_POINT('Ctrl Pts',(26.7035061705199,37.8197338324979,38.6801362695557)) ;
#13933=CARTESIAN_POINT('Ctrl Pts',(26.6665678988832,37.5981822885685,39.3797507718596)) ;
#13934=CARTESIAN_POINT('Ctrl Pts',(26.6296296272465,37.7203996390852,40.0130198185474)) ;
#13935=CARTESIAN_POINT('Ctrl Pts',(26.5926913556098,37.8426169896019,40.6462888652352)) ;
#13936=CARTESIAN_POINT('Ctrl Pts',(26.5557530839731,38.3086032345646,41.213212456307)) ;
#13937=CARTESIAN_POINT('Ctrl Pts',(26.5188148123364,38.9062313848036,41.4557147457038)) ;
#13938=CARTESIAN_POINT('Ctrl Pts',(26.5044997722657,39.1378359114635,41.5496939666077)) ;
#13939=CARTESIAN_POINT('Ctrl Pts',(26.490184732195,39.3892113251267,41.5949493644748)) ;
#13940=CARTESIAN_POINT('Ctrl Pts',(26.4758696921242,39.6410353087582,41.5936514180137)) ;
#13941=CARTESIAN_POINT('Origin',(29.6,39.642135623731,39.642135623731)) ;
#13942=CARTESIAN_POINT('',(25.6741303078758,39.6437755905604,41.5948983538003)) ;
#13943=CARTESIAN_POINT('',(25.7758696921242,39.6437968858784,41.5949974857067)) ;
#13944=CARTESIAN_POINT('',(29.6,39.642135623731,41.596135623731)) ;
#13945=CARTESIAN_POINT('Ctrl Pts',(25.6741303078758,39.6437755905604,41.5948983538003)) ;
#13946=CARTESIAN_POINT('Ctrl Pts',(25.6999387253896,39.1904952337914,41.5912583415157)) ;
#13947=CARTESIAN_POINT('Ctrl Pts',(25.7257471429034,38.734936108021,41.4339712696229)) ;
#13948=CARTESIAN_POINT('Ctrl Pts',(25.7515555604172,38.3888234438755,41.1454096254523)) ;
#13949=CARTESIAN_POINT('Ctrl Pts',(25.7884938320539,37.8934500410593,40.732406062153)) ;
#13950=CARTESIAN_POINT('Ctrl Pts',(25.8254321036906,37.6222748349651,40.0504899918325)) ;
#13951=CARTESIAN_POINT('Ctrl Pts',(25.8623703753273,37.6987426280783,39.4100843171763)) ;
#13952=CARTESIAN_POINT('Ctrl Pts',(25.899308646964,37.7752104211915,38.76967864252)) ;
#13953=CARTESIAN_POINT('Ctrl Pts',(25.9362469186007,38.199321213512,38.170783363528)) ;
#13954=CARTESIAN_POINT('Ctrl Pts',(25.9731851902374,38.7780106252096,37.8860285280915)) ;
#13955=CARTESIAN_POINT('Ctrl Pts',(26.0101234618742,39.3567000369072,37.6012736926549)) ;
#13956=CARTESIAN_POINT('Ctrl Pts',(26.0470617335109,40.0899680679818,37.6306593007738)) ;
#13957=CARTESIAN_POINT('Ctrl Pts',(26.0840000051476,40.6440152956615,37.9608083898478)) ;
#13958=CARTESIAN_POINT('Ctrl Pts',(26.1209382767843,41.1980625233412,38.2909574789218)) ;
#13959=CARTESIAN_POINT('Ctrl Pts',(26.157876548421,41.572888947626,38.9218700489509)) ;
#13960=CARTESIAN_POINT('Ctrl Pts',(26.1948148200577,41.5978654959725,39.5663410906184)) ;
#13961=CARTESIAN_POINT('Ctrl Pts',(26.2317530916944,41.622842044319,40.2108121322859)) ;
#13962=CARTESIAN_POINT('Ctrl Pts',(26.2686913633312,41.2979687167271,40.8688416455917)) ;
#13963=CARTESIAN_POINT('Ctrl Pts',(26.3056296349679,40.7711348587462,41.2408804037869)) ;
#13964=CARTESIAN_POINT('Ctrl Pts',(26.3284631926038,40.4454701557764,41.4708578242687)) ;
#13965=CARTESIAN_POINT('Ctrl Pts',(26.3512967502398,40.0426333156918,41.5915539028743)) ;
#13966=CARTESIAN_POINT('Ctrl Pts',(26.3741303078758,39.6409887519309,41.5937162339903)) ;
#13967=CARTESIAN_POINT('Ctrl Pts',(26.4758696921242,39.6410353087582,41.5936514180137)) ;
#13968=CARTESIAN_POINT('Ctrl Pts',(26.4532464605582,40.0390133980566,41.5916001667979)) ;
#13969=CARTESIAN_POINT('Ctrl Pts',(26.4306232289922,40.4381118389579,41.4732769454704)) ;
#13970=CARTESIAN_POINT('Ctrl Pts',(26.4079999974262,40.7620620933454,41.2472490101119)) ;
#13971=CARTESIAN_POINT('Ctrl Pts',(26.3710617257895,41.2909945961329,40.8781999974013)) ;
#13972=CARTESIAN_POINT('Ctrl Pts',(26.3341234541528,41.6195895461926,40.2220209842581)) ;
#13973=CARTESIAN_POINT('Ctrl Pts',(26.2971851825161,41.5982634351316,39.5774188098299)) ;
#13974=CARTESIAN_POINT('Ctrl Pts',(26.2602469108794,41.5769373240706,38.9328166354017)) ;
#13975=CARTESIAN_POINT('Ctrl Pts',(26.2233086392427,41.2056901518889,38.2997912996883)) ;
#13976=CARTESIAN_POINT('Ctrl Pts',(26.1863703676059,40.6535216383902,37.966509588522)) ;
#13977=CARTESIAN_POINT('Ctrl Pts',(26.1494320959692,40.1013531248915,37.6332278773558)) ;
#13978=CARTESIAN_POINT('Ctrl Pts',(26.1124938243325,39.3682632700758,37.5996897907365)) ;
#13979=CARTESIAN_POINT('Ctrl Pts',(26.0755555526958,38.7879703870318,37.8811625890341)) ;
#13980=CARTESIAN_POINT('Ctrl Pts',(26.0386172810591,38.2076775039878,38.1626353873317)) ;
#13981=CARTESIAN_POINT('Ctrl Pts',(26.0016790094224,37.7801815927156,38.759119070546)) ;
#13982=CARTESIAN_POINT('Ctrl Pts',(25.9647407377857,37.7000880122058,39.3990814011989)) ;
#13983=CARTESIAN_POINT('Ctrl Pts',(25.927802466149,37.6199944316959,40.0390437318518)) ;
#13984=CARTESIAN_POINT('Ctrl Pts',(25.8908641945122,37.8873031819484,40.7224847099434)) ;
#13985=CARTESIAN_POINT('Ctrl Pts',(25.8539259228755,38.3803295545664,41.1382872618806)) ;
#13986=CARTESIAN_POINT('Ctrl Pts',(25.8279071792918,38.7276096573102,41.4311721073528)) ;
#13987=CARTESIAN_POINT('Ctrl Pts',(25.801888435708,39.1868812358737,41.5912661586594)) ;
#13988=CARTESIAN_POINT('Ctrl Pts',(25.7758696921242,39.6437968858784,41.5949974857067)) ;
#13989=CARTESIAN_POINT('Origin',(29.6,39.642135623731,39.642135623731)) ;
#13990=CARTESIAN_POINT('',(24.9741303078758,39.6419511053728,41.5993115726679)) ;
#13991=CARTESIAN_POINT('',(25.0758696921242,39.6418839677207,41.5992928593099)) ;
#13992=CARTESIAN_POINT('',(29.6,39.642135623731,41.596135623731)) ;
#13993=CARTESIAN_POINT('Ctrl Pts',(24.9741303078758,39.6419511053728,41.5993115726679)) ;
#13994=CARTESIAN_POINT('Ctrl Pts',(24.9747041572659,39.6319311937436,41.599325146903)) ;
#13995=CARTESIAN_POINT('Ctrl Pts',(24.975278006656,39.6219114778643,41.5992548129635)) ;
#13996=CARTESIAN_POINT('Ctrl Pts',(24.9758518560462,39.6118930676569,41.5990999903527)) ;
#13997=CARTESIAN_POINT('Ctrl Pts',(25.0127901276829,38.9670152234492,41.5891341704855)) ;
#13998=CARTESIAN_POINT('Ctrl Pts',(25.0497283993196,38.3275473055512,41.2290976426987)) ;
#13999=CARTESIAN_POINT('Ctrl Pts',(25.0866666709563,37.9845889021496,40.6828867996612)) ;
#14000=CARTESIAN_POINT('Ctrl Pts',(25.123604942593,37.641630498748,40.1366759566237)) ;
#14001=CARTESIAN_POINT('Ctrl Pts',(25.1605432142298,37.5951816098427,39.4042907983354)) ;
#14002=CARTESIAN_POINT('Ctrl Pts',(25.1974814858665,37.8663867714669,38.8191288448354)) ;
#14003=CARTESIAN_POINT('Ctrl Pts',(25.2344197575032,38.1375919330911,38.2339668913354)) ;
#14004=CARTESIAN_POINT('Ctrl Pts',(25.2713580291399,38.7264511452448,37.7960281426236)) ;
#14005=CARTESIAN_POINT('Ctrl Pts',(25.3082963007766,39.3649029941181,37.7046717625188)) ;
#14006=CARTESIAN_POINT('Ctrl Pts',(25.3452345724133,40.0033548429913,37.6133153824139)) ;
#14007=CARTESIAN_POINT('Ctrl Pts',(25.38217284405,40.6913993285841,37.8685413709159)) ;
#14008=CARTESIAN_POINT('Ctrl Pts',(25.4191111156868,41.1158237614022,38.3541653533783)) ;
#14009=CARTESIAN_POINT('Ctrl Pts',(25.4560493873235,41.5402481942203,38.8397893358407)) ;
#14010=CARTESIAN_POINT('Ctrl Pts',(25.4929876589602,41.7010525742636,39.5558113122634)) ;
#14011=CARTESIAN_POINT('Ctrl Pts',(25.5299259305969,41.5250352795288,40.1762826359117)) ;
#14012=CARTESIAN_POINT('Ctrl Pts',(25.5668642022336,41.3490179847941,40.7967539595599)) ;
#14013=CARTESIAN_POINT('Ctrl Pts',(25.6038024738703,40.8361790152812,41.3216746304337)) ;
#14014=CARTESIAN_POINT('Ctrl Pts',(25.640740745507,40.2199737307557,41.5120894377316)) ;
#14015=CARTESIAN_POINT('Ctrl Pts',(25.6518705996299,40.0343051917945,41.5694632382416)) ;
#14016=CARTESIAN_POINT('Ctrl Pts',(25.6630004537529,39.8392522890029,41.5964681054409)) ;
#14017=CARTESIAN_POINT('Ctrl Pts',(25.6741303078758,39.6437755905604,41.5948983538003)) ;
#14018=CARTESIAN_POINT('Ctrl Pts',(25.7758696921242,39.6437968858784,41.5949974857067)) ;
#14019=CARTESIAN_POINT('Ctrl Pts',(25.7649501640713,39.8355549253086,41.596563446424)) ;
#14020=CARTESIAN_POINT('Ctrl Pts',(25.7540306360183,40.0268980133607,41.5705891289495)) ;
#14021=CARTESIAN_POINT('Ctrl Pts',(25.7431111079654,40.2093737712261,41.5153321335891)) ;
#14022=CARTESIAN_POINT('Ctrl Pts',(25.7061728363287,40.8266476202843,41.3284103275775)) ;
#14023=CARTESIAN_POINT('Ctrl Pts',(25.669234564692,41.3424513234172,40.8064025897715)) ;
#14024=CARTESIAN_POINT('Ctrl Pts',(25.6322962930553,41.5219799101722,40.1869381010139)) ;
#14025=CARTESIAN_POINT('Ctrl Pts',(25.5953580214185,41.7015084969271,39.5674736122563)) ;
#14026=CARTESIAN_POINT('Ctrl Pts',(25.5584197497818,41.544761967304,38.8505523725471)) ;
#14027=CARTESIAN_POINT('Ctrl Pts',(25.5214814781451,41.1230947222761,38.3625323926646)) ;
#14028=CARTESIAN_POINT('Ctrl Pts',(25.4845432065084,40.7014274772481,37.8745124127821)) ;
#14029=CARTESIAN_POINT('Ctrl Pts',(25.4476049348717,40.0148395168153,37.6153936927263)) ;
#14030=CARTESIAN_POINT('Ctrl Pts',(25.410666663235,39.3758804888048,37.7031326625047)) ;
#14031=CARTESIAN_POINT('Ctrl Pts',(25.3737283915982,38.7369214607943,37.7908716322831)) ;
#14032=CARTESIAN_POINT('Ctrl Pts',(25.3367901199615,38.1455913652061,38.2254682918958)) ;
#14033=CARTESIAN_POINT('Ctrl Pts',(25.2998518483248,37.8710764152813,38.8090848685638)) ;
#14034=CARTESIAN_POINT('Ctrl Pts',(25.2629135766881,37.5965614653565,39.3927014452318)) ;
#14035=CARTESIAN_POINT('Ctrl Pts',(25.2259753050514,37.6388616610951,40.1253379389552)) ;
#14036=CARTESIAN_POINT('Ctrl Pts',(25.1890370334147,37.9787210410719,40.6734824163841)) ;
#14037=CARTESIAN_POINT('Ctrl Pts',(25.152098761778,38.3185804210486,41.221626893813)) ;
#14038=CARTESIAN_POINT('Ctrl Pts',(25.1151604901412,38.9559989852635,41.5852793549473)) ;
#14039=CARTESIAN_POINT('Ctrl Pts',(25.0782222185045,39.6008100555266,41.5988973562706)) ;
#14040=CARTESIAN_POINT('Ctrl Pts',(25.0774380430444,39.6144989747774,41.5991864575734)) ;
#14041=CARTESIAN_POINT('Ctrl Pts',(25.0766538675843,39.6281912257218,41.599317803505)) ;
#14042=CARTESIAN_POINT('Ctrl Pts',(25.0758696921242,39.6418839677207,41.5992928593099)) ;
#14043=CARTESIAN_POINT('Origin',(29.6,39.642135623731,39.642135623731)) ;
#14044=CARTESIAN_POINT('',(24.2741303078758,39.6406455788885,41.5943893719784)) ;
#14045=CARTESIAN_POINT('',(24.3758696921242,39.6406789188743,41.5943026756172)) ;
#14046=CARTESIAN_POINT('',(29.6,39.642135623731,41.596135623731)) ;
#14047=CARTESIAN_POINT('Ctrl Pts',(24.2741303078758,39.6406455788885,41.5943893719784)) ;
#14048=CARTESIAN_POINT('Ctrl Pts',(24.286407860779,39.4248694535981,41.5959340169787)) ;
#14049=CARTESIAN_POINT('Ctrl Pts',(24.2986854136822,39.2095524239628,41.5629298688026)) ;
#14050=CARTESIAN_POINT('Ctrl Pts',(24.3109629665853,39.00679142621,41.4933411485449)) ;
#14051=CARTESIAN_POINT('Ctrl Pts',(24.3479012382221,38.3967642594466,41.2839763775683)) ;
#14052=CARTESIAN_POINT('Ctrl Pts',(24.3848395098588,37.9003903593405,40.7434595224611)) ;
#14053=CARTESIAN_POINT('Ctrl Pts',(24.4217777814955,37.7436298309467,40.1178455134642)) ;
#14054=CARTESIAN_POINT('Ctrl Pts',(24.4587160531322,37.5868693025529,39.4922315044672)) ;
#14055=CARTESIAN_POINT('Ctrl Pts',(24.4956543247689,37.7697221458715,38.7815203415805)) ;
#14056=CARTESIAN_POINT('Ctrl Pts',(24.5325925964056,38.2089498028778,38.3092430746743)) ;
#14057=CARTESIAN_POINT('Ctrl Pts',(24.5695308680423,38.6481774598841,37.8369658077682)) ;
#14058=CARTESIAN_POINT('Ctrl Pts',(24.606469139679,39.3437799305781,37.6031224368427)) ;
#14059=CARTESIAN_POINT('Ctrl Pts',(24.6434074113158,39.9791039676379,37.714163507846)) ;
#14060=CARTESIAN_POINT('Ctrl Pts',(24.6803456829525,40.6144280046977,37.8252045788493)) ;
#14061=CARTESIAN_POINT('Ctrl Pts',(24.7172839545892,41.1894736081234,38.2811300917814)) ;
#14062=CARTESIAN_POINT('Ctrl Pts',(24.7542222262259,41.4424676167279,38.8743929198144)) ;
#14063=CARTESIAN_POINT('Ctrl Pts',(24.7911604978626,41.6954616253324,39.4676557478475)) ;
#14064=CARTESIAN_POINT('Ctrl Pts',(24.8280987694993,41.6264040391158,40.1982558909815)) ;
#14065=CARTESIAN_POINT('Ctrl Pts',(24.865037041136,41.2667313607489,40.7336084065746)) ;
#14066=CARTESIAN_POINT('Ctrl Pts',(24.9014014633826,40.9126463273361,41.2606440274954)) ;
#14067=CARTESIAN_POINT('Ctrl Pts',(24.9377658856292,40.2769056833872,41.5984513831741)) ;
#14068=CARTESIAN_POINT('Ctrl Pts',(24.9741303078758,39.6419511053728,41.5993115726679)) ;
#14069=CARTESIAN_POINT('Ctrl Pts',(25.0758696921242,39.6418839677207,41.5992928593099)) ;
#14070=CARTESIAN_POINT('Ctrl Pts',(25.0397155959476,40.2731823650047,41.5981428171641)) ;
#14071=CARTESIAN_POINT('Ctrl Pts',(25.003561499771,40.9055245646462,41.2647771410003)) ;
#14072=CARTESIAN_POINT('Ctrl Pts',(24.9674074035944,41.2605236498834,40.7427920084966)) ;
#14073=CARTESIAN_POINT('Ctrl Pts',(24.9304691319577,41.6232225976656,40.2094851178871)) ;
#14074=CARTESIAN_POINT('Ctrl Pts',(24.893530860321,41.6964169169187,39.4792877951558)) ;
#14075=CARTESIAN_POINT('Ctrl Pts',(24.8565925886843,41.4467869748733,38.8846016104093)) ;
#14076=CARTESIAN_POINT('Ctrl Pts',(24.8196543170475,41.1971570328278,38.2899154256628)) ;
#14077=CARTESIAN_POINT('Ctrl Pts',(24.7827160454108,40.6247028294838,37.8307403789012)) ;
#14078=CARTESIAN_POINT('Ctrl Pts',(24.7457777737741,39.9900178648199,37.7161028548369)) ;
#14079=CARTESIAN_POINT('Ctrl Pts',(24.7088395021374,39.3553329001561,37.6014653307726)) ;
#14080=CARTESIAN_POINT('Ctrl Pts',(24.6719012305007,38.6584171741724,37.8313653294056)) ;
#14081=CARTESIAN_POINT('Ctrl Pts',(24.634962958864,38.2165217563229,38.3011474129055)) ;
#14082=CARTESIAN_POINT('Ctrl Pts',(24.5980246872273,37.7746263384733,38.7709294964055)) ;
#14083=CARTESIAN_POINT('Ctrl Pts',(24.5610864155906,37.587751228758,39.4805936647722)) ;
#14084=CARTESIAN_POINT('Ctrl Pts',(24.5241481439538,37.7409660076168,40.1070854826224)) ;
#14085=CARTESIAN_POINT('Ctrl Pts',(24.4872098723171,37.8941807864756,40.7335773004725)) ;
#14086=CARTESIAN_POINT('Ctrl Pts',(24.4502716006804,38.3874854539086,41.276896767806)) ;
#14087=CARTESIAN_POINT('Ctrl Pts',(24.4133333290437,38.9963170857706,41.4897131448503)) ;
#14088=CARTESIAN_POINT('Ctrl Pts',(24.4008454500705,39.2021473912189,41.5616608847492)) ;
#14089=CARTESIAN_POINT('Ctrl Pts',(24.3883575710974,39.4211817595164,41.5958340358532)) ;
#14090=CARTESIAN_POINT('Ctrl Pts',(24.3758696921242,39.6406789188743,41.5943026756172)) ;
#14091=CARTESIAN_POINT('Origin',(29.6,39.642135623731,39.642135623731)) ;
#14092=CARTESIAN_POINT('',(23.5741303078758,39.6435118677572,41.5941173638984)) ;
#14093=CARTESIAN_POINT('',(23.6758696921242,39.6435489601981,41.5941990304928)) ;
#14094=CARTESIAN_POINT('',(29.6,39.642135623731,41.596135623731)) ;
#14095=CARTESIAN_POINT('Ctrl Pts',(23.5741303078758,39.6435118677572,41.5941173638984)) ;
#14096=CARTESIAN_POINT('Ctrl Pts',(23.598111564292,39.2218969648424,41.5913563986786)) ;
#14097=CARTESIAN_POINT('Ctrl Pts',(23.6220928207083,38.7986808485727,41.4572211327591)) ;
#14098=CARTESIAN_POINT('Ctrl Pts',(23.6460740771245,38.4642739167478,41.2052306124145)) ;
#14099=CARTESIAN_POINT('Ctrl Pts',(23.6830123487612,37.9491877231577,40.8170902194008)) ;
#14100=CARTESIAN_POINT('Ctrl Pts',(23.7199506203979,37.6448028017159,40.1493362684881)) ;
#14101=CARTESIAN_POINT('Ctrl Pts',(23.7568888920346,37.6896817335956,39.50594476016)) ;
#14102=CARTESIAN_POINT('Ctrl Pts',(23.7938271636714,37.7345606654753,38.8625532518319)) ;
#14103=CARTESIAN_POINT('Ctrl Pts',(23.8307654353081,38.1287034506766,38.2435241860883)) ;
#14104=CARTESIAN_POINT('Ctrl Pts',(23.8677037069448,38.6926877925568,37.9306529447932)) ;
#14105=CARTESIAN_POINT('Ctrl Pts',(23.9046419785815,39.2566721344369,37.617781703498)) ;
#14106=CARTESIAN_POINT('Ctrl Pts',(23.9415802502182,39.9904980329958,37.6110682866512)) ;
#14107=CARTESIAN_POINT('Ctrl Pts',(23.9785185218549,40.5601121121495,37.9135687863955)) ;
#14108=CARTESIAN_POINT('Ctrl Pts',(24.0154567934916,41.1297261913032,38.2160692861397)) ;
#14109=CARTESIAN_POINT('Ctrl Pts',(24.0523950651284,41.5351284510516,38.8277837024749)) ;
#14110=CARTESIAN_POINT('Ctrl Pts',(24.0893333367651,41.591771039095,39.4702464397097)) ;
#14111=CARTESIAN_POINT('Ctrl Pts',(24.1262716084018,41.6484136271384,40.1127091769446)) ;
#14112=CARTESIAN_POINT('Ctrl Pts',(24.1632098800385,41.3562965434769,40.785920235079)) ;
#14113=CARTESIAN_POINT('Ctrl Pts',(24.2001481516752,40.8483977849356,41.1834194207233)) ;
#14114=CARTESIAN_POINT('Ctrl Pts',(24.2248088704087,40.5093145556856,41.4487977175311)) ;
#14115=CARTESIAN_POINT('Ctrl Pts',(24.2494695891422,40.0740539606037,41.5912867947634)) ;
#14116=CARTESIAN_POINT('Ctrl Pts',(24.2741303078758,39.6406455788885,41.5943893719784)) ;
#14117=CARTESIAN_POINT('Ctrl Pts',(24.3758696921242,39.6406789188743,41.5943026756172)) ;
#14118=CARTESIAN_POINT('Ctrl Pts',(24.3514192994607,40.0704389883285,41.5913043794964)) ;
#14119=CARTESIAN_POINT('Ctrl Pts',(24.3269689067971,40.5019731626006,41.4514332027079)) ;
#14120=CARTESIAN_POINT('Ctrl Pts',(24.3025185141336,40.8396492187411,41.1902265352361)) ;
#14121=CARTESIAN_POINT('Ctrl Pts',(24.2655802424968,41.3497911235589,40.7956102618225)) ;
#14122=CARTESIAN_POINT('Ctrl Pts',(24.2286419708601,41.6457163369035,40.1240644282402)) ;
#14123=CARTESIAN_POINT('Ctrl Pts',(24.1917036992234,41.5927133191848,39.4812911817476)) ;
#14124=CARTESIAN_POINT('Ctrl Pts',(24.1547654275867,41.539710301466,38.838517935255)) ;
#14125=CARTESIAN_POINT('Ctrl Pts',(24.11782715595,41.1377790526838,38.2245172758521)) ;
#14126=CARTESIAN_POINT('Ctrl Pts',(24.0808888843133,40.5698873460839,37.918795546384)) ;
#14127=CARTESIAN_POINT('Ctrl Pts',(24.0439506126766,40.0019956394839,37.613073816916)) ;
#14128=CARTESIAN_POINT('Ctrl Pts',(24.0070123410398,39.2681434750662,37.6156310173829)) ;
#14129=CARTESIAN_POINT('Ctrl Pts',(23.9700740694031,38.7023961857,37.9253030549788)) ;
#14130=CARTESIAN_POINT('Ctrl Pts',(23.9331357977664,38.1366488963339,38.2349750925746)) ;
#14131=CARTESIAN_POINT('Ctrl Pts',(23.8961975261297,37.7390064820193,38.8517619672996)) ;
#14132=CARTESIAN_POINT('Ctrl Pts',(23.859259254493,37.6904843460513,39.494888991001)) ;
#14133=CARTESIAN_POINT('Ctrl Pts',(23.8223209828563,37.6419622100833,40.1380160147024)) ;
#14134=CARTESIAN_POINT('Ctrl Pts',(23.7853827112196,37.9425603524618,40.8074831873802)) ;
#14135=CARTESIAN_POINT('Ctrl Pts',(23.7484444395829,38.4554400155153,41.1985346130523)) ;
#14136=CARTESIAN_POINT('Ctrl Pts',(23.7242528570966,38.7913347427045,41.4546416911943)) ;
#14137=CARTESIAN_POINT('Ctrl Pts',(23.7000612746104,39.2182810749139,41.5913309295395)) ;
#14138=CARTESIAN_POINT('Ctrl Pts',(23.6758696921242,39.6435489601981,41.5941990304928)) ;
#14139=CARTESIAN_POINT('Origin',(29.6,39.642135623731,39.642135623731)) ;
#14140=CARTESIAN_POINT('',(22.8741303078758,39.6425352575914,41.5992316723864)) ;
#14141=CARTESIAN_POINT('',(22.9758696921242,39.6424692686163,41.5992623449223)) ;
#14142=CARTESIAN_POINT('',(29.6,39.642135623731,41.596135623731)) ;
#14143=CARTESIAN_POINT('Ctrl Pts',(22.8741303078758,39.6425352575914,41.5992316723864)) ;
#14144=CARTESIAN_POINT('Ctrl Pts',(22.9098152678051,39.019376320101,41.5974825577703)) ;
#14145=CARTESIAN_POINT('Ctrl Pts',(22.9455002277344,38.3946539204701,41.2738928837315)) ;
#14146=CARTESIAN_POINT('Ctrl Pts',(22.9811851876637,38.0377808438174,40.7631485070654)) ;
#14147=CARTESIAN_POINT('Ctrl Pts',(23.0181234593004,37.6683738255288,40.2344659876064)) ;
#14148=CARTESIAN_POINT('Ctrl Pts',(23.0550617309371,37.5859611047416,39.5052515727989)) ;
#14149=CARTESIAN_POINT('Ctrl Pts',(23.0920000025738,37.8280587293757,38.9074593918063)) ;
#14150=CARTESIAN_POINT('Ctrl Pts',(23.1289382742105,38.0701563540097,38.3096672108138)) ;
#14151=CARTESIAN_POINT('Ctrl Pts',(23.1658765458472,38.6367643240651,37.843297263636)) ;
#14152=CARTESIAN_POINT('Ctrl Pts',(23.2028148174839,39.2699504710714,37.7206512088624)) ;
#14153=CARTESIAN_POINT('Ctrl Pts',(23.2397530891207,39.9031366180777,37.5980051540887)) ;
#14154=CARTESIAN_POINT('Ctrl Pts',(23.2766913607574,40.6029009420349,37.8190829917191)) ;
#14155=CARTESIAN_POINT('Ctrl Pts',(23.3136296323941,41.050695630241,38.2832453218724)) ;
#14156=CARTESIAN_POINT('Ctrl Pts',(23.3505679040308,41.4984903184471,38.7474076520257)) ;
#14157=CARTESIAN_POINT('Ctrl Pts',(23.3875061756675,41.6943153709021,39.4546544747018)) ;
#14158=CARTESIAN_POINT('Ctrl Pts',(23.4244444473042,41.5490270002059,40.0830317824199)) ;
#14159=CARTESIAN_POINT('Ctrl Pts',(23.4613827189409,41.4037386295096,40.7114090901379)) ;
#14160=CARTESIAN_POINT('Ctrl Pts',(23.4983209905776,40.9173368356621,41.2609168828979)) ;
#14161=CARTESIAN_POINT('Ctrl Pts',(23.5352592622144,40.3112422058692,41.4814073617205)) ;
#14162=CARTESIAN_POINT('Ctrl Pts',(23.5482162774348,40.0986394771733,41.5587498675684)) ;
#14163=CARTESIAN_POINT('Ctrl Pts',(23.5611732926553,39.8713093867623,41.5956091067727)) ;
#14164=CARTESIAN_POINT('Ctrl Pts',(23.5741303078758,39.6435118677572,41.5941173638984)) ;
#14165=CARTESIAN_POINT('Ctrl Pts',(23.6758696921242,39.6435489601981,41.5941990304928)) ;
#14166=CARTESIAN_POINT('Ctrl Pts',(23.6631230029737,39.8676251463055,41.5957102499976)) ;
#14167=CARTESIAN_POINT('Ctrl Pts',(23.6503763138232,40.0912353453651,41.5600687208437)) ;
#14168=CARTESIAN_POINT('Ctrl Pts',(23.6376296246727,40.3008145556867,41.4851674588105)) ;
#14169=CARTESIAN_POINT('Ctrl Pts',(23.600691353036,40.9081482490762,41.2681132002304)) ;
#14170=CARTESIAN_POINT('Ctrl Pts',(23.5637530813993,41.3976544521269,40.721369004404)) ;
#14171=CARTESIAN_POINT('Ctrl Pts',(23.5268148097626,41.5464993836053,40.0938246213784)) ;
#14172=CARTESIAN_POINT('Ctrl Pts',(23.4898765381259,41.6953443150837,39.4662802383529)) ;
#14173=CARTESIAN_POINT('Ctrl Pts',(23.4529382664891,41.5035279749898,38.7579356681281)) ;
#14174=CARTESIAN_POINT('Ctrl Pts',(23.4159999948524,41.0583692984033,38.2912446365514)) ;
#14175=CARTESIAN_POINT('Ctrl Pts',(23.3790617232157,40.6132106218167,37.8245536049748)) ;
#14176=CARTESIAN_POINT('Ctrl Pts',(23.342123451579,39.9147096087375,37.5995161120464)) ;
#14177=CARTESIAN_POINT('Ctrl Pts',(23.3051851799423,39.2808389854979,37.7185740781279)) ;
#14178=CARTESIAN_POINT('Ctrl Pts',(23.2682469083056,38.6469683622583,37.8376320442095)) ;
#14179=CARTESIAN_POINT('Ctrl Pts',(23.2313086366689,38.0777281288583,38.3007854693011)) ;
#14180=CARTESIAN_POINT('Ctrl Pts',(23.1943703650321,37.8322487168373,38.8971969250653)) ;
#14181=CARTESIAN_POINT('Ctrl Pts',(23.1574320933954,37.5867693048163,39.4936083808294)) ;
#14182=CARTESIAN_POINT('Ctrl Pts',(23.1204938217587,37.6650507141741,40.2232778672661)) ;
#14183=CARTESIAN_POINT('Ctrl Pts',(23.083555550122,38.031457559013,40.7540440967425)) ;
#14184=CARTESIAN_POINT('Ctrl Pts',(23.0476602641228,38.3875185739119,41.2698236598248)) ;
#14185=CARTESIAN_POINT('Ctrl Pts',(23.0117649781235,39.0156637705048,41.5977738151495)) ;
#14186=CARTESIAN_POINT('Ctrl Pts',(22.9758696921242,39.6424692686163,41.5992623449223)) ;
#14187=CARTESIAN_POINT('Origin',(29.6,39.642135623731,39.642135623731)) ;
#14188=CARTESIAN_POINT('',(22.1741303078758,39.6404341197698,41.5952239823215)) ;
#14189=CARTESIAN_POINT('',(22.2758696921242,39.6404509077731,41.5951215653697)) ;
#14190=CARTESIAN_POINT('',(29.6,39.642135623731,41.596135623731)) ;
#14191=CARTESIAN_POINT('Ctrl Pts',(22.1741303078758,39.6404341197698,41.5952239823215)) ;
#14192=CARTESIAN_POINT('Ctrl Pts',(22.1845806996814,39.4569685731193,41.5967725865391)) ;
#14193=CARTESIAN_POINT('Ctrl Pts',(22.195031091487,39.2738961209019,41.5730209579894)) ;
#14194=CARTESIAN_POINT('Ctrl Pts',(22.2054814832926,39.0986059707007,41.5223482889448)) ;
#14195=CARTESIAN_POINT('Ctrl Pts',(22.2424197549294,38.4790200926016,41.343239137007)) ;
#14196=CARTESIAN_POINT('Ctrl Pts',(22.2793580265661,37.9566632719586,40.8277889657132)) ;
#14197=CARTESIAN_POINT('Ctrl Pts',(22.3162962982028,37.7693236058759,40.210641817458)) ;
#14198=CARTESIAN_POINT('Ctrl Pts',(22.3532345698395,37.5819839397931,39.5934946692027)) ;
#14199=CARTESIAN_POINT('Ctrl Pts',(22.3901728414763,37.7296614282706,38.874650543986)) ;
#14200=CARTESIAN_POINT('Ctrl Pts',(22.427111113113,38.1451300903487,38.3813427879068)) ;
#14201=CARTESIAN_POINT('Ctrl Pts',(22.4640493847497,38.5605987524268,37.8880350318277)) ;
#14202=CARTESIAN_POINT('Ctrl Pts',(22.5009876563864,39.2438585881055,37.6202636448861)) ;
#14203=CARTESIAN_POINT('Ctrl Pts',(22.5379259280231,39.8838749852862,37.6999239394952)) ;
#14204=CARTESIAN_POINT('Ctrl Pts',(22.5748641996598,40.5238913824668,37.7795842341044)) ;
#14205=CARTESIAN_POINT('Ctrl Pts',(22.6118024712965,41.1206643411492,38.2066762102643)) ;
#14206=CARTESIAN_POINT('Ctrl Pts',(22.6487407429332,41.4025299386401,38.7867783880528)) ;
#14207=CARTESIAN_POINT('Ctrl Pts',(22.68567901457,41.6843955361311,39.3668805658413)) ;
#14208=CARTESIAN_POINT('Ctrl Pts',(22.7226172862067,41.6513537724305,40.0999929452585)) ;
#14209=CARTESIAN_POINT('Ctrl Pts',(22.7595555578434,41.3184459714061,40.6523869599789)) ;
#14210=CARTESIAN_POINT('Ctrl Pts',(22.7964938294801,40.9855381703818,41.2047809746991)) ;
#14211=CARTESIAN_POINT('Ctrl Pts',(22.8334321011168,40.3527643320338,41.5764566247226)) ;
#14212=CARTESIAN_POINT('Ctrl Pts',(22.8703703727535,39.7081767549648,41.5982191376789)) ;
#14213=CARTESIAN_POINT('Ctrl Pts',(22.8716236844609,39.6863059656452,41.5989575374757)) ;
#14214=CARTESIAN_POINT('Ctrl Pts',(22.8728769961683,39.6644215759027,41.5992931040324)) ;
#14215=CARTESIAN_POINT('Ctrl Pts',(22.8741303078758,39.6425352575914,41.5992316723864)) ;
#14216=CARTESIAN_POINT('Ctrl Pts',(22.9758696921242,39.6424692686163,41.5992623449223)) ;
#14217=CARTESIAN_POINT('Ctrl Pts',(22.9748267064868,39.6606819423368,41.5993055961496)) ;
#14218=CARTESIAN_POINT('Ctrl Pts',(22.9737837208493,39.6788934849888,41.5990732253268)) ;
#14219=CARTESIAN_POINT('Ctrl Pts',(22.9727407352119,39.6970971890957,41.5985618316083)) ;
#14220=CARTESIAN_POINT('Ctrl Pts',(22.9358024635752,40.3417976940196,41.5804503644819)) ;
#14221=CARTESIAN_POINT('Ctrl Pts',(22.8988641919385,40.9766664235475,41.2123644577129)) ;
#14222=CARTESIAN_POINT('Ctrl Pts',(22.8619259203017,41.312697439253,40.6618647549232)) ;
#14223=CARTESIAN_POINT('Ctrl Pts',(22.824987648665,41.6487284549585,40.1113650521334)) ;
#14224=CARTESIAN_POINT('Ctrl Pts',(22.7880493770283,41.6859217568417,39.3784515533227)) ;
#14225=CARTESIAN_POINT('Ctrl Pts',(22.7511111053916,41.407346151666,38.7967622904668)) ;
#14226=CARTESIAN_POINT('Ctrl Pts',(22.7141728337549,41.1287705464904,38.2150730276109)) ;
#14227=CARTESIAN_POINT('Ctrl Pts',(22.6772345621182,40.5344260342559,37.7846080007098)) ;
#14228=CARTESIAN_POINT('Ctrl Pts',(22.6402962904815,39.8948710557536,37.7013241743502)) ;
#14229=CARTESIAN_POINT('Ctrl Pts',(22.6033580188448,39.2553160772512,37.6180403479906)) ;
#14230=CARTESIAN_POINT('Ctrl Pts',(22.566419747208,38.5705506324811,37.8819377221724)) ;
#14231=CARTESIAN_POINT('Ctrl Pts',(22.5294814755713,38.1522947206771,38.3728845202077)) ;
#14232=CARTESIAN_POINT('Ctrl Pts',(22.4925432039346,37.7340388088731,38.863831318243)) ;
#14233=CARTESIAN_POINT('Ctrl Pts',(22.4556049322979,37.5822924300353,39.5818275401316)) ;
#14234=CARTESIAN_POINT('Ctrl Pts',(22.4186666606612,37.7661338089679,40.2000258205355)) ;
#14235=CARTESIAN_POINT('Ctrl Pts',(22.3817283890245,37.9499751879004,40.8182241009394)) ;
#14236=CARTESIAN_POINT('Ctrl Pts',(22.3447901173878,38.4694043246034,41.3366244398584)) ;
#14237=CARTESIAN_POINT('Ctrl Pts',(22.307851845751,39.0879658724486,41.519239821202)) ;
#14238=CARTESIAN_POINT('Ctrl Pts',(22.2971911278754,39.266488306176,41.5719442649668)) ;
#14239=CARTESIAN_POINT('Ctrl Pts',(22.2865304099998,39.45326798981,41.5966794474412)) ;
#14240=CARTESIAN_POINT('Ctrl Pts',(22.2758696921242,39.6404509077731,41.5951215653697)) ;
#14241=CARTESIAN_POINT('Origin',(29.6,39.642135623731,39.642135623731)) ;
#14242=CARTESIAN_POINT('',(21.4741303078758,39.6431273922811,41.5935167596094)) ;
#14243=CARTESIAN_POINT('',(21.5758696921242,39.643176897406,41.5935754761129)) ;
#14244=CARTESIAN_POINT('',(29.6,39.642135623731,41.596135623731)) ;
#14245=CARTESIAN_POINT('Ctrl Pts',(21.4741303078758,39.6431273922811,41.5935167596094)) ;
#14246=CARTESIAN_POINT('Ctrl Pts',(21.4962844031945,39.2533349717856,41.5917134339623)) ;
#14247=CARTESIAN_POINT('Ctrl Pts',(21.5184384985131,38.8625785317564,41.4785841605243)) ;
#14248=CARTESIAN_POINT('Ctrl Pts',(21.5405925938318,38.5425752985296,41.2612685428463)) ;
#14249=CARTESIAN_POINT('Ctrl Pts',(21.5775308654685,38.0090230959449,40.8989308711328)) ;
#14250=CARTESIAN_POINT('Ctrl Pts',(21.6144691371053,37.6721649466632,40.2469549586452)) ;
#14251=CARTESIAN_POINT('Ctrl Pts',(21.651407408742,37.6853463410244,39.6021347637736)) ;
#14252=CARTESIAN_POINT('Ctrl Pts',(21.6883456803787,37.6985277353857,38.9573145689019)) ;
#14253=CARTESIAN_POINT('Ctrl Pts',(21.7252839520154,38.0617486733899,38.3196500916461)) ;
#14254=CARTESIAN_POINT('Ctrl Pts',(21.7622222236521,38.6096629521784,37.9794197241878)) ;
#14255=CARTESIAN_POINT('Ctrl Pts',(21.7991604952888,39.1575772309668,37.6391893567295)) ;
#14256=CARTESIAN_POINT('Ctrl Pts',(21.8360987669255,39.8901848505394,37.5963930990685)) ;
#14257=CARTESIAN_POINT('Ctrl Pts',(21.8730370385622,40.4739871207921,37.870512846321)) ;
#14258=CARTESIAN_POINT('Ctrl Pts',(21.909975310199,41.0577893910447,38.1446325935735)) ;
#14259=CARTESIAN_POINT('Ctrl Pts',(21.9469135818357,41.4927863119774,38.7356683457394)) ;
#14260=CARTESIAN_POINT('Ctrl Pts',(21.9838518534724,41.5809578536104,39.3745678231792)) ;
#14261=CARTESIAN_POINT('Ctrl Pts',(22.0207901251091,41.6691293952435,40.013467300619)) ;
#14262=CARTESIAN_POINT('Ctrl Pts',(22.0577283967458,41.4104755575768,40.7002305033326)) ;
#14263=CARTESIAN_POINT('Ctrl Pts',(22.0946666683825,40.9227411709659,41.1222280383986)) ;
#14264=CARTESIAN_POINT('Ctrl Pts',(22.1211545482136,40.5729941673948,41.4248361329995)) ;
#14265=CARTESIAN_POINT('Ctrl Pts',(22.1476424280447,40.1054514553116,41.5912988431321)) ;
#14266=CARTESIAN_POINT('Ctrl Pts',(22.1741303078758,39.6404341197698,41.5952239823215)) ;
#14267=CARTESIAN_POINT('Ctrl Pts',(22.2758696921242,39.6404509077731,41.5951215653697)) ;
#14268=CARTESIAN_POINT('Ctrl Pts',(22.2495921383631,40.1018372090838,41.5912815491187)) ;
#14269=CARTESIAN_POINT('Ctrl Pts',(22.223314584602,40.5656734448422,41.4276925236177)) ;
#14270=CARTESIAN_POINT('Ctrl Pts',(22.1970370308409,40.914337981394,41.1294571891952)) ;
#14271=CARTESIAN_POINT('Ctrl Pts',(22.1600987592042,41.4044545835068,40.7102287520768)) ;
#14272=CARTESIAN_POINT('Ctrl Pts',(22.1231604875675,41.6669938287453,40.0249414540719)) ;
#14273=CARTESIAN_POINT('Ctrl Pts',(22.0862222159308,41.5824421877824,39.3855528493289)) ;
#14274=CARTESIAN_POINT('Ctrl Pts',(22.049283944294,41.4978905468195,38.7461642445858)) ;
#14275=CARTESIAN_POINT('Ctrl Pts',(22.0123456726573,41.0662480196553,38.1526743331045)) ;
#14276=CARTESIAN_POINT('Ctrl Pts',(21.9754074010206,40.4840075992232,37.8752525310723)) ;
#14277=CARTESIAN_POINT('Ctrl Pts',(21.9384691293839,39.9017671787911,37.5978307290401)) ;
#14278=CARTESIAN_POINT('Ctrl Pts',(21.9015308577472,39.1689288650911,37.636477036457)) ;
#14279=CARTESIAN_POINT('Ctrl Pts',(21.8645925861105,38.6190964543723,37.9735988043494)) ;
#14280=CARTESIAN_POINT('Ctrl Pts',(21.8276543144738,38.0692640436535,38.3107205722417)) ;
#14281=CARTESIAN_POINT('Ctrl Pts',(21.790716042837,37.7024375359159,38.9463178006094)) ;
#14282=CARTESIAN_POINT('Ctrl Pts',(21.7537777712003,37.6856042889378,39.5910529552223)) ;
#14283=CARTESIAN_POINT('Ctrl Pts',(21.7168394995636,37.6687710419596,40.2357881098352)) ;
#14284=CARTESIAN_POINT('Ctrl Pts',(21.6799012279269,38.0019310557408,40.8896611906933)) ;
#14285=CARTESIAN_POINT('Ctrl Pts',(21.6429629562902,38.533422666923,41.2550150036193)) ;
#14286=CARTESIAN_POINT('Ctrl Pts',(21.6205985349015,38.8552163467658,41.476219902121)) ;
#14287=CARTESIAN_POINT('Ctrl Pts',(21.5982341135129,39.2497133228765,41.591661008618)) ;
#14288=CARTESIAN_POINT('Ctrl Pts',(21.5758696921242,39.643176897406,41.5935754761129)) ;
#14289=CARTESIAN_POINT('Origin',(29.6,39.642135623731,39.642135623731)) ;
#14290=CARTESIAN_POINT('',(20.7741303078758,39.6430525564623,41.598752263752)) ;
#14291=CARTESIAN_POINT('',(20.8758696921242,39.6430106825472,41.5988377495572)) ;
#14292=CARTESIAN_POINT('',(29.6,39.642135623731,41.596135623731)) ;
#14293=CARTESIAN_POINT('Ctrl Pts',(20.7741303078758,39.6430525564623,41.598752263752)) ;
#14294=CARTESIAN_POINT('Ctrl Pts',(20.8079881067075,39.0514242059577,41.5952420385212)) ;
#14295=CARTESIAN_POINT('Ctrl Pts',(20.8418459055392,38.4568801100053,41.3080512591221)) ;
#14296=CARTESIAN_POINT('Ctrl Pts',(20.875703704371,38.0948628415535,40.8407051836536)) ;
#14297=CARTESIAN_POINT('Ctrl Pts',(20.9126419760077,37.6999082768545,40.3308387162615)) ;
#14298=CARTESIAN_POINT('Ctrl Pts',(20.9495802476444,37.5817171822124,39.6065436368026)) ;
#14299=CARTESIAN_POINT('Ctrl Pts',(20.9865185192811,37.7941178194275,38.9975639952763)) ;
#14300=CARTESIAN_POINT('Ctrl Pts',(21.0234567909178,38.0065184566426,38.38858435375)) ;
#14301=CARTESIAN_POINT('Ctrl Pts',(21.0603950625546,38.5495108257149,37.8949201501563)) ;
#14302=CARTESIAN_POINT('Ctrl Pts',(21.0973333341913,39.1759005105809,37.7412833052911)) ;
#14303=CARTESIAN_POINT('Ctrl Pts',(21.134271605828,39.8022901954467,37.5876464604258)) ;
#14304=CARTESIAN_POINT('Ctrl Pts',(21.1712098774647,40.5120771961061,37.7740369742889)) ;
#14305=CARTESIAN_POINT('Ctrl Pts',(21.2081481491014,40.9821574581571,38.2156132098312)) ;
#14306=CARTESIAN_POINT('Ctrl Pts',(21.2450864207381,41.4522377202081,38.6571894453736)) ;
#14307=CARTESIAN_POINT('Ctrl Pts',(21.2820246923748,41.6826112436507,39.3539514025952)) ;
#14308=CARTESIAN_POINT('Ctrl Pts',(21.3189629640115,41.5684038796714,39.9887143339762)) ;
#14309=CARTESIAN_POINT('Ctrl Pts',(21.3559012356483,41.4541965156921,40.6234772653574)) ;
#14310=CARTESIAN_POINT('Ctrl Pts',(21.392839507285,40.9954082642909,41.196241170898)) ;
#14311=CARTESIAN_POINT('Ctrl Pts',(21.4297777789217,40.4008910106465,41.4462734081986)) ;
#14312=CARTESIAN_POINT('Ctrl Pts',(21.4445619552397,40.1629413851623,41.5463463276301)) ;
#14313=CARTESIAN_POINT('Ctrl Pts',(21.4593461315577,39.9032490442437,41.5947201797419)) ;
#14314=CARTESIAN_POINT('Ctrl Pts',(21.4741303078758,39.6431273922811,41.5935167596094)) ;
#14315=CARTESIAN_POINT('Ctrl Pts',(21.5758696921242,39.643176897406,41.5935754761129)) ;
#14316=CARTESIAN_POINT('Ctrl Pts',(21.5612958418762,39.8995787561265,41.5948230452806)) ;
#14317=CARTESIAN_POINT('Ctrl Pts',(21.5467219916281,40.1555417786995,41.5478612892325)) ;
#14318=CARTESIAN_POINT('Ctrl Pts',(21.53214814138,40.3906611063697,41.4505420266541)) ;
#14319=CARTESIAN_POINT('Ctrl Pts',(21.4952098697433,40.9865847260513,41.2038806917688)) ;
#14320=CARTESIAN_POINT('Ctrl Pts',(21.4582715981066,41.4486087568314,40.6337234770042)) ;
#14321=CARTESIAN_POINT('Ctrl Pts',(21.4213333264699,41.566409737262,39.9996179837209)) ;
#14322=CARTESIAN_POINT('Ctrl Pts',(21.3843950548332,41.6842107176926,39.3655124904376)) ;
#14323=CARTESIAN_POINT('Ctrl Pts',(21.3474567831965,41.4577886477738,38.6674587186358)) ;
#14324=CARTESIAN_POINT('Ctrl Pts',(21.3105185115598,40.990216052329,38.2232263199088)) ;
#14325=CARTESIAN_POINT('Ctrl Pts',(21.2735802399231,40.5226434568841,37.7789939211818)) ;
#14326=CARTESIAN_POINT('Ctrl Pts',(21.2366419682863,39.8139203359133,37.5885828955297)) ;
#14327=CARTESIAN_POINT('Ctrl Pts',(21.1997036966496,39.1866721101622,37.7386714115382)) ;
#14328=CARTESIAN_POINT('Ctrl Pts',(21.1627654250129,38.5594238844111,37.8887599275467)) ;
#14329=CARTESIAN_POINT('Ctrl Pts',(21.1258271533762,38.0136505538797,38.3793479852159)) ;
#14330=CARTESIAN_POINT('Ctrl Pts',(21.0888888817395,37.797801167441,38.9871113914114)) ;
#14331=CARTESIAN_POINT('Ctrl Pts',(21.0519506101028,37.5819517810022,39.5948747976069)) ;
#14332=CARTESIAN_POINT('Ctrl Pts',(21.0150123384661,37.6960263386562,40.3198135523287)) ;
#14333=CARTESIAN_POINT('Ctrl Pts',(20.9780740668294,38.0880931290849,40.831915760622)) ;
#14334=CARTESIAN_POINT('Ctrl Pts',(20.9440059419277,38.4496958731846,41.3042270307907)) ;
#14335=CARTESIAN_POINT('Ctrl Pts',(20.9099378170259,39.0477685794782,41.595492055224)) ;
#14336=CARTESIAN_POINT('Ctrl Pts',(20.8758696921242,39.6430106825472,41.5988377495572)) ;
#14337=CARTESIAN_POINT('Origin',(29.6,39.642135623731,39.642135623731)) ;
#14338=CARTESIAN_POINT('',(20.1,39.642135623731,41.596135623731)) ;
#14339=CARTESIAN_POINT('',(20.1758696921242,39.6403856614379,41.5960667040991)) ;
#14340=CARTESIAN_POINT('',(29.6,39.642135623731,41.596135623731)) ;
#14341=CARTESIAN_POINT('',(20.1,39.1924719723276,41.5436925123374)) ;
#14342=CARTESIAN_POINT('Origin',(20.1,39.642135623731,39.642135623731)) ;
#14343=CARTESIAN_POINT('Ctrl Pts',(20.1,39.1924719723275,41.5436925123374)) ;
#14344=CARTESIAN_POINT('Ctrl Pts',(20.1369382716367,38.561997188093,41.3946033132209)) ;
#14345=CARTESIAN_POINT('Ctrl Pts',(20.1738765432734,38.0168810177416,40.9084697851729)) ;
#14346=CARTESIAN_POINT('Ctrl Pts',(20.2108148149101,37.7999421624532,40.3022386179921)) ;
#14347=CARTESIAN_POINT('Ctrl Pts',(20.2477530865469,37.5830033071648,39.6960074508112)) ;
#14348=CARTESIAN_POINT('Ctrl Pts',(20.2846913581836,37.6942417669393,38.9696786444975)) ;
#14349=CARTESIAN_POINT('Ctrl Pts',(20.3216296298203,38.0847160955708,38.4562506191992)) ;
#14350=CARTESIAN_POINT('Ctrl Pts',(20.358567901457,38.4751904242022,37.9428225939008)) ;
#14351=CARTESIAN_POINT('Ctrl Pts',(20.3955061730937,39.1449006216906,37.6422953496178)) ;
#14352=CARTESIAN_POINT('Ctrl Pts',(20.4324444447304,39.7881721301733,37.6905138623107)) ;
#14353=CARTESIAN_POINT('Ctrl Pts',(20.4693827163671,40.4314436386561,37.7387323750036)) ;
#14354=CARTESIAN_POINT('Ctrl Pts',(20.5063209880039,41.0482764581332,38.1356966446725)) ;
#14355=CARTESIAN_POINT('Ctrl Pts',(20.5432592596406,41.3582757099971,38.701169032257)) ;
#14356=CARTESIAN_POINT('Ctrl Pts',(20.5801975312773,41.6682749618611,39.2666414198415)) ;
#14357=CARTESIAN_POINT('Ctrl Pts',(20.617135802914,41.6714406461119,40.0006219253415)) ;
#14358=CARTESIAN_POINT('Ctrl Pts',(20.6540740745507,41.3661313458041,40.5687529999006)) ;
#14359=CARTESIAN_POINT('Ctrl Pts',(20.6910123461874,41.0608220454964,41.1368840744597)) ;
#14360=CARTESIAN_POINT('Ctrl Pts',(20.7279506178241,40.4470377606301,41.5391657180777)) ;
#14361=CARTESIAN_POINT('Ctrl Pts',(20.7648888894608,39.8042866008192,41.5925876122242)) ;
#14362=CARTESIAN_POINT('Ctrl Pts',(20.7679693622658,39.750684269675,41.597042739246)) ;
#14363=CARTESIAN_POINT('Ctrl Pts',(20.7710498350708,39.6968804811139,41.599071633402)) ;
#14364=CARTESIAN_POINT('Ctrl Pts',(20.7741303078758,39.6430525564623,41.598752263752)) ;
#14365=CARTESIAN_POINT('Ctrl Pts',(20.8758696921242,39.6430106825472,41.5988377495572)) ;
#14366=CARTESIAN_POINT('Ctrl Pts',(20.8729995453892,39.6931582085291,41.5991196151924)) ;
#14367=CARTESIAN_POINT('Ctrl Pts',(20.8701293986542,39.7432856440115,41.5973579435593)) ;
#14368=CARTESIAN_POINT('Ctrl Pts',(20.8672592519192,39.7932498983189,41.5934888294942)) ;
#14369=CARTESIAN_POINT('Ctrl Pts',(20.8303209802825,40.4362808539208,41.5436940282085)) ;
#14370=CARTESIAN_POINT('Ctrl Pts',(20.7933827086458,41.0522837419213,41.1448387637723)) ;
#14371=CARTESIAN_POINT('Ctrl Pts',(20.7564444370091,41.3608307362133,40.5784740403519)) ;
#14372=CARTESIAN_POINT('Ctrl Pts',(20.7195061653724,41.6693777305054,40.0121093169316)) ;
#14373=CARTESIAN_POINT('Ctrl Pts',(20.6825678937356,41.6704688310889,39.2782351345271)) ;
#14374=CARTESIAN_POINT('Ctrl Pts',(20.6456296220989,41.36362737304,38.7109598395018)) ;
#14375=CARTESIAN_POINT('Ctrl Pts',(20.6086913504622,41.0567859149911,38.1436845444765)) ;
#14376=CARTESIAN_POINT('Ctrl Pts',(20.5717530788255,40.4420118983097,37.7430081368304)) ;
#14377=CARTESIAN_POINT('Ctrl Pts',(20.5348148071888,39.7991237067178,37.6912612551126)) ;
#14378=CARTESIAN_POINT('Ctrl Pts',(20.4978765355521,39.156235515126,37.6395143733948)) ;
#14379=CARTESIAN_POINT('Ctrl Pts',(20.4609382639154,38.4852331486237,37.9366970176053)) ;
#14380=CARTESIAN_POINT('Ctrl Pts',(20.4239999922786,38.0916512795126,38.447656902979)) ;
#14381=CARTESIAN_POINT('Ctrl Pts',(20.3870617206419,37.6980694104016,38.9586167883527)) ;
#14382=CARTESIAN_POINT('Ctrl Pts',(20.3501234490052,37.5819080386817,39.6833539148898)) ;
#14383=CARTESIAN_POINT('Ctrl Pts',(20.3131851773685,37.7958866514344,40.2916891358699)) ;
#14384=CARTESIAN_POINT('Ctrl Pts',(20.2762469057318,38.0098652641872,40.90002435685)) ;
#14385=CARTESIAN_POINT('Ctrl Pts',(20.2393086340951,38.5539838614125,41.3919576722732)) ;
#14386=CARTESIAN_POINT('Ctrl Pts',(20.2023703624584,39.1808671084928,41.5440782600819)) ;
#14387=CARTESIAN_POINT('Ctrl Pts',(20.1935368056803,39.3307823186778,41.5804569478217)) ;
#14388=CARTESIAN_POINT('Ctrl Pts',(20.1847032489023,39.4854308170824,41.59740183643)) ;
#14389=CARTESIAN_POINT('Ctrl Pts',(20.1758696921242,39.6403856614379,41.5960667040991)) ;
#14390=CARTESIAN_POINT('Origin',(30.6940562256037,39.642135623731,39.642135623731)) ;
#14391=CARTESIAN_POINT('',(20.5440562256037,39.6428655566193,41.1997186245255)) ;
#14392=CARTESIAN_POINT('',(20.4059437743963,39.6407425498585,41.1975807596125)) ;
#14393=CARTESIAN_POINT('',(30.6940562256037,39.6421356237311,41.197635623731)) ;
#14394=CARTESIAN_POINT('',(20.1,38.4771632437029,38.6076638930866)) ;
#14395=CARTESIAN_POINT('Ctrl Pts',(20.5440562256037,39.6428655566193,41.1997186245255)) ;
#14396=CARTESIAN_POINT('Ctrl Pts',(20.5409757527987,39.6857157801584,41.1999728617264)) ;
#14397=CARTESIAN_POINT('Ctrl Pts',(20.500957008357,40.242137908518,41.1789906663339)) ;
#14398=CARTESIAN_POINT('Ctrl Pts',(20.4239999922786,41.260102964655,40.5118040569248)) ;
#14399=CARTESIAN_POINT('Ctrl Pts',(20.3131851773685,41.2525427468677,38.758927890642)) ;
#14400=CARTESIAN_POINT('Ctrl Pts',(20.2051851799423,39.8168546376957,37.8349872964746)) ;
#14401=CARTESIAN_POINT('Ctrl Pts',(20.1341234541528,38.7943081205531,38.2545323388419)) ;
#14402=CARTESIAN_POINT('Ctrl Pts',(20.1,38.4771632437029,38.6076638930866)) ;
#14403=CARTESIAN_POINT('',(20.1,40.2413475545766,38.2066826248723)) ;
#14404=CARTESIAN_POINT('Origin',(20.1,39.642135623731,39.642135623731)) ;
#14405=CARTESIAN_POINT('Ctrl Pts',(20.4059437743963,39.6407425498585,41.1975807596125)) ;
#14406=CARTESIAN_POINT('Ctrl Pts',(20.3778390595376,40.0332014593976,41.1941992288133)) ;
#14407=CARTESIAN_POINT('Ctrl Pts',(20.3127960730423,40.9471855575388,40.8454705034782)) ;
#14408=CARTESIAN_POINT('Ctrl Pts',(20.2108148149101,41.4478477610965,39.3100962723047)) ;
#14409=CARTESIAN_POINT('Ctrl Pts',(20.1369382716367,40.7172822611094,38.4053556254406)) ;
#14410=CARTESIAN_POINT('Ctrl Pts',(20.1,40.2413475545766,38.2066826248723)) ;
#14411=CARTESIAN_POINT('Origin',(30.6940562256037,39.642135623731,39.642135623731)) ;
#14412=CARTESIAN_POINT('',(21.2440562256037,39.6429251303736,41.1955508524203)) ;
#14413=CARTESIAN_POINT('',(21.1059437743963,39.642832222497,41.1997866763014)) ;
#14414=CARTESIAN_POINT('',(30.6940562256037,39.6421356237311,41.197635623731)) ;
#14415=CARTESIAN_POINT('Ctrl Pts',(21.2440562256037,39.6429251303736,41.1955508524203)) ;
#14416=CARTESIAN_POINT('Ctrl Pts',(21.2292720492857,39.8499974075629,41.1965088462873)) ;
#14417=CARTESIAN_POINT('Ctrl Pts',(21.177549601331,40.5732442315414,41.061786987415)) ;
#14418=CARTESIAN_POINT('Ctrl Pts',(21.0888888817395,41.4498663517249,39.9673877570378)) ;
#14419=CARTESIAN_POINT('Ctrl Pts',(20.9780740668294,40.8996933490919,38.3033961125266)) ;
#14420=CARTESIAN_POINT('Ctrl Pts',(20.8672592519192,39.2045955811405,37.8582623699771)) ;
#14421=CARTESIAN_POINT('Ctrl Pts',(20.7564444370091,37.907833098911,39.0372204078837)) ;
#14422=CARTESIAN_POINT('Ctrl Pts',(20.6487100949039,38.1822480719097,40.7188819177846)) ;
#14423=CARTESIAN_POINT('Ctrl Pts',(20.5779140244354,39.1718942673614,41.1969242768559)) ;
#14424=CARTESIAN_POINT('Ctrl Pts',(20.5440562256037,39.6428655566193,41.1997186245255)) ;
#14425=CARTESIAN_POINT('Ctrl Pts',(21.1059437743963,39.642832222497,41.1997866763014)) ;
#14426=CARTESIAN_POINT('Ctrl Pts',(21.1030736276613,39.6827526302068,41.2000110580801)) ;
#14427=CARTESIAN_POINT('Ctrl Pts',(21.0632652092896,40.2362196732324,41.1805600891616)) ;
#14428=CARTESIAN_POINT('Ctrl Pts',(20.9865185192811,41.2550721079325,40.520864063088)) ;
#14429=CARTESIAN_POINT('Ctrl Pts',(20.875703704371,41.257677850447,38.7682418152935)) ;
#14430=CARTESIAN_POINT('Ctrl Pts',(20.7648888894608,39.7894880096876,37.8113551948838)) ;
#14431=CARTESIAN_POINT('Ctrl Pts',(20.6540740745507,38.1870148554998,38.5210802763619)) ;
#14432=CARTESIAN_POINT('Ctrl Pts',(20.5432592596406,37.9096008119324,40.25188160747)) ;
#14433=CARTESIAN_POINT('Ctrl Pts',(20.4605491595891,38.8794875060849,41.1287484880954)) ;
#14434=CARTESIAN_POINT('Ctrl Pts',(20.4147773311743,39.5173892947945,41.1986436042086)) ;
#14435=CARTESIAN_POINT('Ctrl Pts',(20.4059437743963,39.6407425498585,41.1975807596125)) ;
#14436=CARTESIAN_POINT('Origin',(30.6940562256037,39.642135623731,39.642135623731)) ;
#14437=CARTESIAN_POINT('',(21.9440562256037,39.6407811255675,41.1969099030491)) ;
#14438=CARTESIAN_POINT('',(21.8059437743963,39.6429645393921,41.1955975942428)) ;
#14439=CARTESIAN_POINT('',(30.6940562256037,39.6421356237311,41.197635623731)) ;
#14440=CARTESIAN_POINT('Ctrl Pts',(21.9440562256037,39.6407811255675,41.1969099030491)) ;
#14441=CARTESIAN_POINT('Ctrl Pts',(21.9175683457726,40.0109625306009,41.1937852592368)) ;
#14442=CARTESIAN_POINT('Ctrl Pts',(21.8541421943048,40.9021886596065,40.876475390125)) ;
#14443=CARTESIAN_POINT('Ctrl Pts',(21.7537777712003,41.4616468090319,39.3910334034537)) ;
#14444=CARTESIAN_POINT('Ctrl Pts',(21.6429629562902,40.4227966905405,37.9795347660523)) ;
#14445=CARTESIAN_POINT('Ctrl Pts',(21.53214814138,38.6731992203584,38.0817398511981)) ;
#14446=CARTESIAN_POINT('Ctrl Pts',(21.4213333264699,37.8057629321309,39.6045961885133)) ;
#14447=CARTESIAN_POINT('Ctrl Pts',(21.3253026878778,38.5029121757861,40.9539015719257)) ;
#14448=CARTESIAN_POINT('Ctrl Pts',(21.2662103209224,39.3326272234746,41.1941152981501)) ;
#14449=CARTESIAN_POINT('Ctrl Pts',(21.2440562256037,39.6429251303736,41.1955508524203)) ;
#14450=CARTESIAN_POINT('Ctrl Pts',(21.8059437743963,39.6429645393921,41.1955975942428)) ;
#14451=CARTESIAN_POINT('Ctrl Pts',(21.7913699241482,39.8470756403336,41.1965907333627)) ;
#14452=CARTESIAN_POINT('Ctrl Pts',(21.7398578022635,40.56728344443,41.0644535876924)) ;
#14453=CARTESIAN_POINT('Ctrl Pts',(21.6514074087419,41.4479940364311,39.977619430384)) ;
#14454=CARTESIAN_POINT('Ctrl Pts',(21.5405925938318,40.9072578085518,38.3105427025879)) ;
#14455=CARTESIAN_POINT('Ctrl Pts',(21.4297777789217,39.2147007747696,37.8558072618482)) ;
#14456=CARTESIAN_POINT('Ctrl Pts',(21.3189629640115,37.9112968612974,39.0274189154373)) ;
#14457=CARTESIAN_POINT('Ctrl Pts',(21.2110182958364,38.1766711691164,40.7138608723637)) ;
#14458=CARTESIAN_POINT('Ctrl Pts',(21.140011899298,39.168984171666,41.1971233049938)) ;
#14459=CARTESIAN_POINT('Ctrl Pts',(21.1059437743963,39.642832222497,41.1997866763014)) ;
#14460=CARTESIAN_POINT('Origin',(30.6940562256037,39.642135623731,39.642135623731)) ;
#14461=CARTESIAN_POINT('',(22.6440562256037,39.6424537560083,41.2001002622589)) ;
#14462=CARTESIAN_POINT('',(22.5059437743963,39.6407944898148,41.1968283730754)) ;
#14463=CARTESIAN_POINT('',(30.6940562256037,39.6421356237311,41.197635623731)) ;
#14464=CARTESIAN_POINT('Ctrl Pts',(22.6440562256037,39.6424537560083,41.2001002622589)) ;
#14465=CARTESIAN_POINT('Ctrl Pts',(22.6428029138963,39.6598765646743,41.200149165496)) ;
#14466=CARTESIAN_POINT('Ctrl Pts',(22.6046113305522,40.1907469072132,41.1920090101158)) ;
#14467=CARTESIAN_POINT('Ctrl Pts',(22.5294814755713,41.2152893427001,40.5902182080807)) ;
#14468=CARTESIAN_POINT('Ctrl Pts',(22.4186666606612,41.2941989590302,38.8394152814942)) ;
#14469=CARTESIAN_POINT('Ctrl Pts',(22.307851845751,39.8689988506925,37.8194435789608)) ;
#14470=CARTESIAN_POINT('Ctrl Pts',(22.1970370308409,38.2372526771025,38.4589293400473)) ;
#14471=CARTESIAN_POINT('Ctrl Pts',(22.0862222159307,37.884572533817,40.1756571344811)) ;
#14472=CARTESIAN_POINT('Ctrl Pts',(22.0018952808517,38.8338703266282,41.1124032256132)) ;
#14473=CARTESIAN_POINT('Ctrl Pts',(21.9545066174093,39.4947316589273,41.1981426839398)) ;
#14474=CARTESIAN_POINT('Ctrl Pts',(21.9440562256037,39.6407811255675,41.1969099030491)) ;
#14475=CARTESIAN_POINT('Ctrl Pts',(22.5059437743963,39.6407944898148,41.1968283730754)) ;
#14476=CARTESIAN_POINT('Ctrl Pts',(22.4796662206352,40.0080853760424,41.1937714921755)) ;
#14477=CARTESIAN_POINT('Ctrl Pts',(22.4164503952374,40.8963676775261,40.8804858433475)) ;
#14478=CARTESIAN_POINT('Ctrl Pts',(22.3162962982028,41.4630397864066,39.4013424185359)) ;
#14479=CARTESIAN_POINT('Ctrl Pts',(22.2054814832927,40.432200557639,37.9839828116129)) ;
#14480=CARTESIAN_POINT('Ctrl Pts',(22.0946666683825,38.682052148795,38.0762770764856)) ;
#14481=CARTESIAN_POINT('Ctrl Pts',(21.9838518534724,37.806005117906,39.594196455287)) ;
#14482=CARTESIAN_POINT('Ctrl Pts',(21.8876108888103,38.4970109681013,40.9503919933712)) ;
#14483=CARTESIAN_POINT('Ctrl Pts',(21.8283081957849,39.3297441759424,41.1940735644637)) ;
#14484=CARTESIAN_POINT('Ctrl Pts',(21.8059437743963,39.6429645393921,41.1955975942428)) ;
#14485=CARTESIAN_POINT('Origin',(30.6940562256037,39.642135623731,39.642135623731)) ;
#14486=CARTESIAN_POINT('',(23.3440562256037,39.6432311956772,41.1960289690894)) ;
#14487=CARTESIAN_POINT('',(23.2059437743963,39.6424012248667,41.2001246794184)) ;
#14488=CARTESIAN_POINT('',(30.6940562256037,39.6421356237311,41.197635623731)) ;
#14489=CARTESIAN_POINT('Ctrl Pts',(23.3440562256037,39.6432311956772,41.1960289690894)) ;
#14490=CARTESIAN_POINT('Ctrl Pts',(23.3310992103832,39.8245715440971,41.1972164849753)) ;
#14491=CARTESIAN_POINT('Ctrl Pts',(23.2812039235261,40.5214498349615,41.0842248278971)) ;
#14492=CARTESIAN_POINT('Ctrl Pts',(23.1943703650321,41.4316808979472,40.0558999560533)) ;
#14493=CARTESIAN_POINT('Ctrl Pts',(23.083555550122,40.9640157969843,38.366868585522)) ;
#14494=CARTESIAN_POINT('Ctrl Pts',(22.9727407352119,39.2928539659985,37.8388953361349)) ;
#14495=CARTESIAN_POINT('Ctrl Pts',(22.8619259203017,37.9396932227727,38.9526698287169)) ;
#14496=CARTESIAN_POINT('Ctrl Pts',(22.752364417099,38.1342834924026,40.6744674861658)) ;
#14497=CARTESIAN_POINT('Ctrl Pts',(22.679741185533,39.1463822476838,41.1987078631876)) ;
#14498=CARTESIAN_POINT('Ctrl Pts',(22.6440562256037,39.6424537560083,41.2001002622589)) ;
#14499=CARTESIAN_POINT('Ctrl Pts',(23.2059437743963,39.6424012248667,41.2001246794184)) ;
#14500=CARTESIAN_POINT('Ctrl Pts',(23.2049007887588,39.6568995943509,41.2001591099629)) ;
#14501=CARTESIAN_POINT('Ctrl Pts',(23.1669195314847,40.184837931591,41.1934228620692)) ;
#14502=CARTESIAN_POINT('Ctrl Pts',(23.0920000025738,41.2098945632884,40.5991127594935)) ;
#14503=CARTESIAN_POINT('Ctrl Pts',(22.9811851876637,41.2987187921716,38.848784795215)) ;
#14504=CARTESIAN_POINT('Ctrl Pts',(22.8703703727535,39.8793182464488,37.8207576467842)) ;
#14505=CARTESIAN_POINT('Ctrl Pts',(22.7595555578434,38.2439764102052,38.4509915754534)) ;
#14506=CARTESIAN_POINT('Ctrl Pts',(22.6487407429332,37.8815790320852,40.1656944257316)) ;
#14507=CARTESIAN_POINT('Ctrl Pts',(22.5642034817842,38.8279106834674,41.1101517427012)) ;
#14508=CARTESIAN_POINT('Ctrl Pts',(22.5166044922719,39.4917857749265,41.1980685396886)) ;
#14509=CARTESIAN_POINT('Ctrl Pts',(22.5059437743963,39.6407944898148,41.1968283730754)) ;
#14510=CARTESIAN_POINT('Origin',(30.6940562256037,39.642135623731,39.642135623731)) ;
#14511=CARTESIAN_POINT('',(24.0440562256037,39.6409494595793,41.196245503669)) ;
#14512=CARTESIAN_POINT('',(23.9059437743963,39.6432607234622,41.1960939805468)) ;
#14513=CARTESIAN_POINT('',(30.6940562256037,39.6421356237311,41.197635623731)) ;
#14514=CARTESIAN_POINT('Ctrl Pts',(24.0440562256037,39.6409494595793,41.196245503669)) ;
#14515=CARTESIAN_POINT('Ctrl Pts',(24.0193955068702,39.9859682608884,41.1937756680201)) ;
#14516=CARTESIAN_POINT('Ctrl Pts',(23.9577965164999,40.8514594910534,40.9104441463242)) ;
#14517=CARTESIAN_POINT('Ctrl Pts',(23.859259254493,41.4717945581916,39.4808241401565)) ;
#14518=CARTESIAN_POINT('Ctrl Pts',(23.7484444395829,40.5036217613051,38.0199411699272)) ;
#14519=CARTESIAN_POINT('Ctrl Pts',(23.6376296246727,38.7511148239329,38.0359740049913)) ;
#14520=CARTESIAN_POINT('Ctrl Pts',(23.5268148097626,37.8098316575348,39.5143256607193)) ;
#14521=CARTESIAN_POINT('Ctrl Pts',(23.4289570100729,38.4517613530902,40.9225790274919)) ;
#14522=CARTESIAN_POINT('Ctrl Pts',(23.36803748202,39.3076007036178,41.1938310768686)) ;
#14523=CARTESIAN_POINT('Ctrl Pts',(23.3440562256037,39.6432311956772,41.1960289690894)) ;
#14524=CARTESIAN_POINT('Ctrl Pts',(23.9059437743963,39.6432607234622,41.1960939805468)) ;
#14525=CARTESIAN_POINT('Ctrl Pts',(23.8931970852458,39.821638669977,41.1972970009867)) ;
#14526=CARTESIAN_POINT('Ctrl Pts',(23.8435121244586,40.5154871172593,41.0867035675646)) ;
#14527=CARTESIAN_POINT('Ctrl Pts',(23.7568888920346,41.4293088255812,40.0660286263046)) ;
#14528=CARTESIAN_POINT('Ctrl Pts',(23.6460740771245,40.9712172436731,38.3743756391225)) ;
#14529=CARTESIAN_POINT('Ctrl Pts',(23.5352592622143,39.3030724240549,37.8369460276841)) ;
#14530=CARTESIAN_POINT('Ctrl Pts',(23.4244444473042,37.9436253671659,38.9430388926739)) ;
#14531=CARTESIAN_POINT('Ctrl Pts',(23.3146726180315,38.1288157471692,40.669218461723)) ;
#14532=CARTESIAN_POINT('Ctrl Pts',(23.2418390603956,39.1434268378081,41.198939721352)) ;
#14533=CARTESIAN_POINT('Ctrl Pts',(23.2059437743963,39.6424012248667,41.2001246794184)) ;
#14534=CARTESIAN_POINT('Origin',(30.6940562256037,39.642135623731,39.642135623731)) ;
#14535=CARTESIAN_POINT('',(24.7440562256037,39.641988736164,41.2001638676263)) ;
#14536=CARTESIAN_POINT('',(24.6059437743963,39.6409760001874,41.1961764882187)) ;
#14537=CARTESIAN_POINT('',(30.6940562256037,39.6421356237311,41.197635623731)) ;
#14538=CARTESIAN_POINT('Ctrl Pts',(24.7440562256037,39.641988736164,41.2001638676263)) ;
#14539=CARTESIAN_POINT('Ctrl Pts',(24.7076918033571,40.1474502745986,41.1994791057237)) ;
#14540=CARTESIAN_POINT('Ctrl Pts',(24.6343891094738,41.1676111809988,40.6574060741533)) ;
#14541=CARTESIAN_POINT('Ctrl Pts',(24.5241481439538,41.3316789557939,38.9216381981518)) ;
#14542=CARTESIAN_POINT('Ctrl Pts',(24.4133333290437,39.9583676413693,37.8328068746627)) ;
#14543=CARTESIAN_POINT('Ctrl Pts',(24.3025185141336,38.2971450571862,38.3912664910517)) ;
#14544=CARTESIAN_POINT('Ctrl Pts',(24.1917036992234,37.8604599019426,40.0885713229918)) ;
#14545=CARTESIAN_POINT('Ctrl Pts',(24.1055496030468,38.7820838555419,41.092156082151)) ;
#14546=CARTESIAN_POINT('Ctrl Pts',(24.0563337785069,39.4691788542113,41.1974751327877)) ;
#14547=CARTESIAN_POINT('Ctrl Pts',(24.0440562256037,39.6409494595793,41.196245503669)) ;
#14548=CARTESIAN_POINT('Ctrl Pts',(24.6059437743963,39.6409760001874,41.1961764882187)) ;
#14549=CARTESIAN_POINT('Ctrl Pts',(24.5814933817327,39.9830905283532,41.1937896665114)) ;
#14550=CARTESIAN_POINT('Ctrl Pts',(24.5201047174324,40.8455982589183,40.9142290234479)) ;
#14551=CARTESIAN_POINT('Ctrl Pts',(24.4217777814955,41.4726788523376,39.4911892118972)) ;
#14552=CARTESIAN_POINT('Ctrl Pts',(24.3109629665853,40.5127954478126,38.0248462860509)) ;
#14553=CARTESIAN_POINT('Ctrl Pts',(24.2001481516752,38.7602257828917,38.0309533361934)) ;
#14554=CARTESIAN_POINT('Ctrl Pts',(24.0893333367651,37.8105848789005,39.5039502404432)) ;
#14555=CARTESIAN_POINT('Ctrl Pts',(23.9912652110054,38.445891019574,40.9188512189262)) ;
#14556=CARTESIAN_POINT('Ctrl Pts',(23.9301353568825,39.304722240576,41.193810801922)) ;
#14557=CARTESIAN_POINT('Ctrl Pts',(23.9059437743963,39.6432607234622,41.1960939805468)) ;
#14558=CARTESIAN_POINT('Origin',(30.6940562256037,39.642135623731,39.642135623731)) ;
#14559=CARTESIAN_POINT('',(25.4440562256037,39.6434411346846,41.1966506834151)) ;
#14560=CARTESIAN_POINT('',(25.3059437743963,39.6419352906073,41.2001489706823)) ;
#14561=CARTESIAN_POINT('',(30.6940562256037,39.6421356237311,41.197635623731)) ;
#14562=CARTESIAN_POINT('Ctrl Pts',(25.4440562256037,39.6434411346846,41.1966506834151)) ;
#14563=CARTESIAN_POINT('Ctrl Pts',(25.4329263714808,39.799052191198,41.1979002989099)) ;
#14564=CARTESIAN_POINT('Ctrl Pts',(25.3848582457212,40.4696553434449,41.10505600482)) ;
#14565=CARTESIAN_POINT('Ctrl Pts',(25.2998518483248,41.4091655775236,40.1434123472918)) ;
#14566=CARTESIAN_POINT('Ctrl Pts',(25.1890370334147,41.0251360793291,38.4334243467918)) ;
#14567=CARTESIAN_POINT('Ctrl Pts',(25.0782222185045,39.3819633096162,37.8238992314671)) ;
#14568=CARTESIAN_POINT('Ctrl Pts',(24.9674074035944,37.9756626373976,38.8697749586234)) ;
#14569=CARTESIAN_POINT('Ctrl Pts',(24.8565925886842,38.0865908564746,40.6188411516388)) ;
#14570=CARTESIAN_POINT('Ctrl Pts',(24.7821421960207,39.1126080506474,41.196514648151)) ;
#14571=CARTESIAN_POINT('Ctrl Pts',(24.7446300749939,39.634012291671,41.2001746735233)) ;
#14572=CARTESIAN_POINT('Ctrl Pts',(24.7440562256037,39.641988736164,41.2001638676263)) ;
#14573=CARTESIAN_POINT('Ctrl Pts',(25.3059437743963,39.6419352906073,41.2001489706824)) ;
#14574=CARTESIAN_POINT('Ctrl Pts',(25.2697896782197,40.1444862921299,41.1992334688615)) ;
#14575=CARTESIAN_POINT('Ctrl Pts',(25.1966973104064,41.16216841065,40.6627197145167)) ;
#14576=CARTESIAN_POINT('Ctrl Pts',(25.0866666709563,41.3357325096837,38.9312186673045)) ;
#14577=CARTESIAN_POINT('Ctrl Pts',(24.9758518560461,39.9686099201725,37.8346268783008)) ;
#14578=CARTESIAN_POINT('Ctrl Pts',(24.8650370411361,38.304251048472,38.3836690193557)) ;
#14579=CARTESIAN_POINT('Ctrl Pts',(24.7542222262259,37.8579600047224,40.0784734419163)) ;
#14580=CARTESIAN_POINT('Ctrl Pts',(24.6678578039793,38.7761213015138,41.0897245806797)) ;
#14581=CARTESIAN_POINT('Ctrl Pts',(24.6184316533695,39.4662432308008,41.1973955418764)) ;
#14582=CARTESIAN_POINT('Ctrl Pts',(24.6059437743963,39.6409760001874,41.1961764882187)) ;
#14583=CARTESIAN_POINT('Origin',(30.6940562256037,39.642135623731,39.642135623731)) ;
#14584=CARTESIAN_POINT('',(26.1440562256037,39.6412226456937,41.1957096458694)) ;
#14585=CARTESIAN_POINT('',(26.0059437743963,39.6434580870219,41.1967295982976)) ;
#14586=CARTESIAN_POINT('',(30.6940562256037,39.6421356237311,41.197635623731)) ;
#14587=CARTESIAN_POINT('Ctrl Pts',(26.1440562256037,39.6412226456937,41.1957096458694)) ;
#14588=CARTESIAN_POINT('Ctrl Pts',(26.1212226679677,39.9609555622393,41.1939883019333)) ;
#14589=CARTESIAN_POINT('Ctrl Pts',(26.0614508386951,40.800410911607,40.9424746399457)) ;
#14590=CARTESIAN_POINT('Ctrl Pts',(25.9647407377856,41.477513974956,39.571005327472)) ;
#14591=CARTESIAN_POINT('Ctrl Pts',(25.8539259228755,40.5823617185973,38.064273747103)) ;
#14592=CARTESIAN_POINT('Ctrl Pts',(25.7431111079654,38.8311870681316,37.9940956814497)) ;
#14593=CARTESIAN_POINT('Ctrl Pts',(25.6322962930552,37.8183349635443,39.4243642686637)) ;
#14594=CARTESIAN_POINT('Ctrl Pts',(25.532611332268,38.4009054869355,40.8893367037083)) ;
#14595=CARTESIAN_POINT('Ctrl Pts',(25.4698646431175,39.2826030615248,41.1937530175458)) ;
#14596=CARTESIAN_POINT('Ctrl Pts',(25.4440562256037,39.6434411346846,41.1966506834151)) ;
#14597=CARTESIAN_POINT('Ctrl Pts',(26.0059437743963,39.6434580870219,41.1967295982976)) ;
#14598=CARTESIAN_POINT('Ctrl Pts',(25.9950242463433,39.7961088702019,41.1979761959925)) ;
#14599=CARTESIAN_POINT('Ctrl Pts',(25.9471664466537,40.4636946757718,41.1073531908352)) ;
#14600=CARTESIAN_POINT('Ctrl Pts',(25.8623703753273,41.4062982291994,40.1534120973844)) ;
#14601=CARTESIAN_POINT('Ctrl Pts',(25.7515555604172,41.0319596004962,38.4412764960012)) ;
#14602=CARTESIAN_POINT('Ctrl Pts',(25.640740745507,39.392265272267,37.822454844445)) ;
#14603=CARTESIAN_POINT('Ctrl Pts',(25.5299259305969,37.9800636903518,38.8603490676194)) ;
#14604=CARTESIAN_POINT('Ctrl Pts',(25.4191111156867,38.0810840912803,40.6100154944158)) ;
#14605=CARTESIAN_POINT('Ctrl Pts',(25.3444503969532,39.1067023870668,41.1951390511897)) ;
#14606=CARTESIAN_POINT('Ctrl Pts',(25.3067279498564,39.631035055101,41.2001688277425)) ;
#14607=CARTESIAN_POINT('Ctrl Pts',(25.3059437743963,39.6419352906073,41.2001489706824)) ;
#14608=CARTESIAN_POINT('Origin',(30.6940562256037,39.642135623731,39.642135623731)) ;
#14609=CARTESIAN_POINT('',(26.8440562256037,39.6415425595799,41.1998999830041)) ;
#14610=CARTESIAN_POINT('',(26.7059437743963,39.6412597076922,41.1956580485042)) ;
#14611=CARTESIAN_POINT('',(30.6940562256037,39.6421356237311,41.197635623731)) ;
#14612=CARTESIAN_POINT('Ctrl Pts',(26.8440562256037,39.6415425595799,41.1998999830041)) ;
#14613=CARTESIAN_POINT('Ctrl Pts',(26.8095189644547,40.1218241840523,41.1975493661777)) ;
#14614=CARTESIAN_POINT('Ctrl Pts',(26.7380434316689,41.1199631784081,40.7026026237249)) ;
#14615=CARTESIAN_POINT('Ctrl Pts',(26.6296296272465,41.3650697227584,39.0056049473486)) ;
#14616=CARTESIAN_POINT('Ctrl Pts',(26.5188148123364,40.0469710495945,37.8505493184767)) ;
#14617=CARTESIAN_POINT('Ctrl Pts',(26.4079999974262,38.3602927420783,38.3266311433769)) ;
#14618=CARTESIAN_POINT('Ctrl Pts',(26.2971851825161,37.8406594871401,40.0004049924068)) ;
#14619=CARTESIAN_POINT('Ctrl Pts',(26.2092039252419,38.7302854054079,41.0703220356036)) ;
#14620=CARTESIAN_POINT('Ctrl Pts',(26.1581609396045,39.4437176656815,41.1967729520918)) ;
#14621=CARTESIAN_POINT('Ctrl Pts',(26.1440562256037,39.6412226456937,41.1957096458694)) ;
#14622=CARTESIAN_POINT('Ctrl Pts',(26.7059437743963,39.6412597076922,41.1956580485042)) ;
#14623=CARTESIAN_POINT('Ctrl Pts',(26.6833205428303,39.9580738929038,41.194025130763)) ;
#14624=CARTESIAN_POINT('Ctrl Pts',(26.6237590396275,40.7945171726604,40.9460395382985)) ;
#14625=CARTESIAN_POINT('Ctrl Pts',(26.5272592647882,41.4778874257816,39.5814013470451)) ;
#14626=CARTESIAN_POINT('Ctrl Pts',(26.416444449878,40.5912830608963,38.0696241059467)) ;
#14627=CARTESIAN_POINT('Ctrl Pts',(26.3056296349679,38.8405339270694,37.9895291820938)) ;
#14628=CARTESIAN_POINT('Ctrl Pts',(26.1948148200577,37.8195975555487,39.4140384490947)) ;
#14629=CARTESIAN_POINT('Ctrl Pts',(26.0949195332006,38.3950733473823,40.8853847393576)) ;
#14630=CARTESIAN_POINT('Ctrl Pts',(26.0319625179801,39.2797261046359,41.1937592404563)) ;
#14631=CARTESIAN_POINT('Ctrl Pts',(26.0059437743963,39.6434580870219,41.1967295982976)) ;
#14632=CARTESIAN_POINT('Origin',(30.6940562256037,39.642135623731,39.642135623731)) ;
#14633=CARTESIAN_POINT('',(27.5440562256037,39.6435335091576,41.197371464458)) ;
#14634=CARTESIAN_POINT('',(27.4059437743963,39.6414949228124,41.1998520948235)) ;
#14635=CARTESIAN_POINT('',(30.6940562256037,39.6421356237311,41.197635623731)) ;
#14636=CARTESIAN_POINT('Ctrl Pts',(27.5440562256037,39.6435335091576,41.197371464458)) ;
#14637=CARTESIAN_POINT('Ctrl Pts',(27.5347535325783,39.7734451527461,41.1985318984516)) ;
#14638=CARTESIAN_POINT('Ctrl Pts',(27.4885125679163,40.4178911838916,41.1243328333579)) ;
#14639=CARTESIAN_POINT('Ctrl Pts',(27.4053333316175,41.3823734685628,40.2297114846548)) ;
#14640=CARTESIAN_POINT('Ctrl Pts',(27.2945185167073,41.0829090703606,38.5029055750713)) ;
#14641=CARTESIAN_POINT('Ctrl Pts',(27.1837037017972,39.4717023486403,37.8133038337068)) ;
#14642=CARTESIAN_POINT('Ctrl Pts',(27.0728888868871,38.0156654467869,38.7887494467938)) ;
#14643=CARTESIAN_POINT('Ctrl Pts',(26.9620740719769,38.0404371457719,40.5411546443971)) ;
#14644=CARTESIAN_POINT('Ctrl Pts',(26.8857965182158,39.0612544298047,41.1839889943965)) ;
#14645=CARTESIAN_POINT('Ctrl Pts',(26.8464572360914,39.6081536578824,41.2000633965309)) ;
#14646=CARTESIAN_POINT('Ctrl Pts',(26.8440562256037,39.6415425595799,41.1998999830041)) ;
#14647=CARTESIAN_POINT('Ctrl Pts',(27.4059437743963,39.6414949228124,41.1998520948236)) ;
#14648=CARTESIAN_POINT('Ctrl Pts',(27.3716168393172,40.1188907313755,41.1973562034564)) ;
#14649=CARTESIAN_POINT('Ctrl Pts',(27.3003516326014,41.1144275745993,40.7076660016292)) ;
#14650=CARTESIAN_POINT('Ctrl Pts',(27.192148154249,41.3686471870141,39.0153731842676)) ;
#14651=CARTESIAN_POINT('Ctrl Pts',(27.0813333393388,40.0571114221001,37.8528708534111)) ;
#14652=CARTESIAN_POINT('Ctrl Pts',(26.9705185244287,38.367763791755,38.3193923515952)) ;
#14653=CARTESIAN_POINT('Ctrl Pts',(26.8597037095185,37.8386592473608,39.9901963817902)) ;
#14654=CARTESIAN_POINT('Ctrl Pts',(26.7715121261745,38.724323513277,41.0677045090039)) ;
#14655=CARTESIAN_POINT('Ctrl Pts',(26.720258814467,39.4407928670888,41.1966912909403)) ;
#14656=CARTESIAN_POINT('Ctrl Pts',(26.7059437743963,39.6412597076922,41.1956580485042)) ;
#14657=CARTESIAN_POINT('Origin',(30.6940562256037,39.642135623731,39.642135623731)) ;
#14658=CARTESIAN_POINT('',(28.2440562256037,39.6415737394006,41.1953392395473)) ;
#14659=CARTESIAN_POINT('',(28.1059437743963,39.6435359003472,41.1974583899176)) ;
#14660=CARTESIAN_POINT('',(30.6940562256037,39.6421356237311,41.197635623731)) ;
#14661=CARTESIAN_POINT('Ctrl Pts',(28.2440562256037,39.6415737394006,41.1953392395473)) ;
#14662=CARTESIAN_POINT('Ctrl Pts',(28.2230498290653,39.9358973857211,41.1943802817051)) ;
#14663=CARTESIAN_POINT('Ctrl Pts',(28.1651051608901,40.7491092810725,40.9726167632119)) ;
#14664=CARTESIAN_POINT('Ctrl Pts',(28.0702222210783,41.4787901727068,39.6613583328092)) ;
#14665=CARTESIAN_POINT('Ctrl Pts',(27.9594074061682,40.6588265422981,38.1124254201628)) ;
#14666=CARTESIAN_POINT('Ctrl Pts',(27.848592591258,38.9132218087539,37.956206051659)) ;
#14667=CARTESIAN_POINT('Ctrl Pts',(27.7377777763479,37.8312525732956,39.3349299949331)) ;
#14668=CARTESIAN_POINT('Ctrl Pts',(27.6362656544631,38.3504124819495,40.8541260832666)) ;
#14669=CARTESIAN_POINT('Ctrl Pts',(27.571691804215,39.257604033775,41.1939241546557)) ;
#14670=CARTESIAN_POINT('Ctrl Pts',(27.5440562256037,39.6435335091576,41.197371464458)) ;
#14671=CARTESIAN_POINT('Ctrl Pts',(28.1059437743963,39.6435359003471,41.1974583899176)) ;
#14672=CARTESIAN_POINT('Ctrl Pts',(28.0968514074409,39.7704922710606,41.1986001215001)) ;
#14673=CARTESIAN_POINT('Ctrl Pts',(28.0508207688488,40.4119358388835,41.126454460646)) ;
#14674=CARTESIAN_POINT('Ctrl Pts',(27.96785185862,41.3790176807763,40.2395580544964)) ;
#14675=CARTESIAN_POINT('Ctrl Pts',(27.8570370437098,41.0893382026773,38.5110838439939)) ;
#14676=CARTESIAN_POINT('Ctrl Pts',(27.7462222287997,39.4820628559708,37.812367849582)) ;
#14677=CARTESIAN_POINT('Ctrl Pts',(27.6354074138896,38.02052476931,38.7795514216669)) ;
#14678=CARTESIAN_POINT('Ctrl Pts',(27.5245925989794,38.0353711001173,40.5320688312148)) ;
#14679=CARTESIAN_POINT('Ctrl Pts',(27.4481047191483,39.0553359645197,41.1824628553531)) ;
#14680=CARTESIAN_POINT('Ctrl Pts',(27.408555110954,39.6051782191946,41.2000419635769)) ;
#14681=CARTESIAN_POINT('Ctrl Pts',(27.4059437743963,39.6414949228124,41.1998520948236)) ;
#14682=CARTESIAN_POINT('Origin',(30.6940562256037,39.642135623731,39.642135623731)) ;
#14683=CARTESIAN_POINT('',(28.9440562256037,39.6410873345839,41.199362363652)) ;
#14684=CARTESIAN_POINT('',(28.8059437743963,39.6416116368869,41.195305032435)) ;
#14685=CARTESIAN_POINT('',(30.6940562256037,39.6421356237311,41.197635623731)) ;
#14686=CARTESIAN_POINT('Ctrl Pts',(28.9440562256037,39.6410873345839,41.199362363652)) ;
#14687=CARTESIAN_POINT('Ctrl Pts',(28.9113461255522,40.0963330616707,41.1960267055326)) ;
#14688=CARTESIAN_POINT('Ctrl Pts',(28.8416977538641,41.0716738723266,40.7456795001595)) ;
#14689=CARTESIAN_POINT('Ctrl Pts',(28.7351111105392,41.3942255244127,39.0910907111602)) ;
#14690=CARTESIAN_POINT('Ctrl Pts',(28.624296295629,40.1346271265577,37.8726387777184)) ;
#14691=CARTESIAN_POINT('Ctrl Pts',(28.5134814807189,38.4265266238107,38.2651743224326)) ;
#14692=CARTESIAN_POINT('Ctrl Pts',(28.4026666658087,37.8252273599387,39.911374245203)) ;
#14693=CARTESIAN_POINT('Ctrl Pts',(28.312858247437,38.6785065574203,41.0468480488814)) ;
#14694=CARTESIAN_POINT('Ctrl Pts',(28.259988100702,39.4183499435878,41.1960665416592)) ;
#14695=CARTESIAN_POINT('Ctrl Pts',(28.2440562256037,39.6415737394006,41.1953392395473)) ;
#14696=CARTESIAN_POINT('Ctrl Pts',(28.8059437743963,39.6416116368869,41.195305032435)) ;
#14697=CARTESIAN_POINT('Ctrl Pts',(28.7851477039278,39.9330056123089,41.1944331137349)) ;
#14698=CARTESIAN_POINT('Ctrl Pts',(28.7274133618227,40.7432003839351,40.9759731746722)) ;
#14699=CARTESIAN_POINT('Ctrl Pts',(28.6327407480808,41.4786453053513,39.671756482491)) ;
#14700=CARTESIAN_POINT('Ctrl Pts',(28.5219259331707,40.6674772372708,38.1182099023464)) ;
#14701=CARTESIAN_POINT('Ctrl Pts',(28.4111111182605,38.9227802986979,37.9521038579512)) ;
#14702=CARTESIAN_POINT('Ctrl Pts',(28.3002963033504,37.8330223043396,39.324679226451)) ;
#14703=CARTESIAN_POINT('Ctrl Pts',(28.1985738553956,38.3446264340712,40.8499443789831)) ;
#14704=CARTESIAN_POINT('Ctrl Pts',(28.1337896790776,39.2547246023744,41.1939617702834)) ;
#14705=CARTESIAN_POINT('Ctrl Pts',(28.1059437743963,39.6435359003471,41.1974583899176)) ;
#14706=CARTESIAN_POINT('Origin',(20.1,39.642135623731,39.642135623731)) ;
#14707=CARTESIAN_POINT('Ctrl Pts',(20.1,38.4771632437029,38.6076638930866)) ;
#14708=CARTESIAN_POINT('Ctrl Pts',(20.1,38.4471842989757,38.633695702627)) ;
#14709=CARTESIAN_POINT('Ctrl Pts',(20.1,38.4183276248831,38.6608956116623)) ;
#14710=CARTESIAN_POINT('Ctrl Pts',(20.1,38.3906795143262,38.6892240882464)) ;
#14711=CARTESIAN_POINT('Ctrl Pts',(20.1,38.3492091017984,38.7317150066697)) ;
#14712=CARTESIAN_POINT('Ctrl Pts',(20.1,38.3104558584504,38.7767427355807)) ;
#14713=CARTESIAN_POINT('Ctrl Pts',(20.1,38.2744245066081,38.8239788897696)) ;
#14714=CARTESIAN_POINT('Ctrl Pts',(20.1,38.2522070410619,38.8531054025028)) ;
#14715=CARTESIAN_POINT('Ctrl Pts',(20.1,38.231024980398,38.883072537858)) ;
#14716=CARTESIAN_POINT('Ctrl Pts',(20.1,38.2108850074198,38.9138110407869)) ;
#14717=CARTESIAN_POINT('Ctrl Pts',(20.1,38.2038364321758,38.9245688829656)) ;
#14718=CARTESIAN_POINT('Ctrl Pts',(20.1,38.1969169630732,38.9354192430819)) ;
#14719=CARTESIAN_POINT('Ctrl Pts',(20.1,38.1901324830045,38.9463496455857)) ;
#14720=CARTESIAN_POINT('Ctrl Pts',(20.1,38.1572723307046,38.9992902817637)) ;
#14721=CARTESIAN_POINT('Ctrl Pts',(20.1,38.1275364351092,39.0541653253696)) ;
#14722=CARTESIAN_POINT('Ctrl Pts',(20.1,38.1009316604637,39.1106156981426)) ;
#14723=CARTESIAN_POINT('Ctrl Pts',(20.1,38.0804217583057,39.1541338875573)) ;
#14724=CARTESIAN_POINT('Ctrl Pts',(20.1,38.0617732267877,39.1985894369993)) ;
#14725=CARTESIAN_POINT('Ctrl Pts',(20.1,38.0450033095947,39.2438334856589)) ;
#14726=CARTESIAN_POINT('Ctrl Pts',(20.1,38.0383575665427,39.2617632296501)) ;
#14727=CARTESIAN_POINT('Ctrl Pts',(20.1,38.0320069970726,39.2798169309718)) ;
#14728=CARTESIAN_POINT('Ctrl Pts',(20.1,38.0259532717025,39.2979857743449)) ;
#14729=CARTESIAN_POINT('Ctrl Pts',(20.1,38.0220625131859,39.3096629776816)) ;
#14730=CARTESIAN_POINT('Ctrl Pts',(20.1,38.0182944593548,39.3213878357419)) ;
#14731=CARTESIAN_POINT('Ctrl Pts',(20.1,38.014653688814,39.3331439108972)) ;
#14732=CARTESIAN_POINT('Ctrl Pts',(20.1,37.9955205478867,39.3949249652588)) ;
#14733=CARTESIAN_POINT('Ctrl Pts',(20.1,37.9798674930171,39.4576596257358)) ;
#14734=CARTESIAN_POINT('Ctrl Pts',(20.1,37.9677029541813,39.5209827002554)) ;
#14735=CARTESIAN_POINT('Ctrl Pts',(20.1,37.9552821571085,39.5856397389857)) ;
#14736=CARTESIAN_POINT('Ctrl Pts',(20.1,37.9464978419906,39.6509111700541)) ;
#14737=CARTESIAN_POINT('Ctrl Pts',(20.1,37.9414013169079,39.7164413416117)) ;
#14738=CARTESIAN_POINT('Ctrl Pts',(20.1,37.9380042773892,39.7601198438917)) ;
#14739=CARTESIAN_POINT('Ctrl Pts',(20.1,37.9362465210122,39.8039139704257)) ;
#14740=CARTESIAN_POINT('Ctrl Pts',(20.1,37.9361552286675,39.84772306421)) ;
#14741=CARTESIAN_POINT('Ctrl Pts',(20.1,37.93610984702,39.8695006717415)) ;
#14742=CARTESIAN_POINT('Ctrl Pts',(20.1,37.9364764227937,39.891282016996)) ;
#14743=CARTESIAN_POINT('Ctrl Pts',(20.1,37.9372592574947,39.9130548757857)) ;
#14744=CARTESIAN_POINT('Ctrl Pts',(20.1,37.9377989933606,39.9280664647964)) ;
#14745=CARTESIAN_POINT('Ctrl Pts',(20.1,37.9385366154168,39.9430740212226)) ;
#14746=CARTESIAN_POINT('Ctrl Pts',(20.1,37.9394737196895,39.9580735415047)) ;
#14747=CARTESIAN_POINT('Ctrl Pts',(20.1,37.9401376118804,39.9686999623553)) ;
#14748=CARTESIAN_POINT('Ctrl Pts',(20.1,37.9409010314124,39.9793127680792)) ;
#14749=CARTESIAN_POINT('Ctrl Pts',(20.1,37.9417640229791,39.9899103038919)) ;
#14750=CARTESIAN_POINT('Ctrl Pts',(20.1,37.9472618141605,40.0574231756069)) ;
#14751=CARTESIAN_POINT('Ctrl Pts',(20.1,37.9567969806614,40.124316733486)) ;
#14752=CARTESIAN_POINT('Ctrl Pts',(20.1,37.9704106721731,40.1902188479243)) ;
#14753=CARTESIAN_POINT('Ctrl Pts',(20.1,37.9736714320761,40.2060037635811)) ;
#14754=CARTESIAN_POINT('Ctrl Pts',(20.1,37.9771663964514,40.2217318853767)) ;
#14755=CARTESIAN_POINT('Ctrl Pts',(20.1,37.9808965550334,40.237398231313)) ;
#14756=CARTESIAN_POINT('Ctrl Pts',(20.1,37.9959250015805,40.3005164171257)) ;
#14757=CARTESIAN_POINT('Ctrl Pts',(20.1,38.0147669309706,40.3626320365636)) ;
#14758=CARTESIAN_POINT('Ctrl Pts',(20.1,38.0371591550646,40.4235632338164)) ;
#14759=CARTESIAN_POINT('Ctrl Pts',(20.1,38.0493406366329,40.4567101089616)) ;
#14760=CARTESIAN_POINT('Ctrl Pts',(20.1,38.0625737285448,40.4895064459427)) ;
#14761=CARTESIAN_POINT('Ctrl Pts',(20.1,38.0768223050403,40.5219221617345)) ;
#14762=CARTESIAN_POINT('Ctrl Pts',(20.1,38.0891447183764,40.5499558287257)) ;
#14763=CARTESIAN_POINT('Ctrl Pts',(20.1,38.1022266974373,40.5777048279095)) ;
#14764=CARTESIAN_POINT('Ctrl Pts',(20.1,38.116047303518,40.6051489944802)) ;
#14765=CARTESIAN_POINT('Ctrl Pts',(20.1,38.1207119187167,40.6144117197005)) ;
#14766=CARTESIAN_POINT('Ctrl Pts',(20.1,38.1254594051322,40.6236370495224)) ;
#14767=CARTESIAN_POINT('Ctrl Pts',(20.1,38.1302848214216,40.6328168606391)) ;
#14768=CARTESIAN_POINT('Ctrl Pts',(20.1,38.1618484692572,40.6928631463702)) ;
#14769=CARTESIAN_POINT('Ctrl Pts',(20.1,38.1967886424964,40.7510552902723)) ;
#14770=CARTESIAN_POINT('Ctrl Pts',(20.1,38.2347975138951,40.8072008920799)) ;
#14771=CARTESIAN_POINT('Ctrl Pts',(20.1,38.2736045218223,40.8645254780053)) ;
#14772=CARTESIAN_POINT('Ctrl Pts',(20.1,38.3156108209451,40.9197174906792)) ;
#14773=CARTESIAN_POINT('Ctrl Pts',(20.1,38.3605432443238,40.9725628487746)) ;
#14774=CARTESIAN_POINT('Ctrl Pts',(20.1,38.4058108269567,41.0258023901674)) ;
#14775=CARTESIAN_POINT('Ctrl Pts',(20.1,38.454048885018,41.0766610251022)) ;
#14776=CARTESIAN_POINT('Ctrl Pts',(20.1,38.5050257934815,41.1248975541876)) ;
#14777=CARTESIAN_POINT('Ctrl Pts',(20.1,38.5181105797675,41.1372789380982)) ;
#14778=CARTESIAN_POINT('Ctrl Pts',(20.1,38.5313760345214,41.1494874120446)) ;
#14779=CARTESIAN_POINT('Ctrl Pts',(20.1,38.5448186744254,41.1615185503207)) ;
#14780=CARTESIAN_POINT('Ctrl Pts',(20.1,38.5539017265004,41.1696478654154)) ;
#14781=CARTESIAN_POINT('Ctrl Pts',(20.1,38.5630662700531,41.1776966072414)) ;
#14782=CARTESIAN_POINT('Ctrl Pts',(20.1,38.5722987266649,41.1856529081345)) ;
#14783=CARTESIAN_POINT('Ctrl Pts',(20.1,38.6269868720595,41.2327817881649)) ;
#14784=CARTESIAN_POINT('Ctrl Pts',(20.1,38.6841537809393,41.2767594894807)) ;
#14785=CARTESIAN_POINT('Ctrl Pts',(20.1,38.7435015175629,41.3173659232921)) ;
#14786=CARTESIAN_POINT('Ctrl Pts',(20.1,38.8029893136318,41.3580681874572)) ;
#14787=CARTESIAN_POINT('Ctrl Pts',(20.1,38.8646688888385,41.3953841416024)) ;
#14788=CARTESIAN_POINT('Ctrl Pts',(20.1,38.9282849740291,41.4290653215661)) ;
#14789=CARTESIAN_POINT('Ctrl Pts',(20.1,38.9905426948541,41.4620273231251)) ;
#14790=CARTESIAN_POINT('Ctrl Pts',(20.1,39.0546558560331,41.4915088253113)) ;
#14791=CARTESIAN_POINT('Ctrl Pts',(20.1,39.1204174970525,41.5172396967087)) ;
#14792=CARTESIAN_POINT('Ctrl Pts',(20.1,39.1442223983483,41.5265539541447)) ;
#14793=CARTESIAN_POINT('Ctrl Pts',(20.1,39.1682435659401,41.5353763365805)) ;
#14794=CARTESIAN_POINT('Ctrl Pts',(20.1,39.1924719723276,41.5436925123374)) ;
#14795=CARTESIAN_POINT('',(20.1,40.8748717950665,41.1621520113221)) ;
#14796=CARTESIAN_POINT('Origin',(20.1,39.642135623731,39.642135623731)) ;
#14797=CARTESIAN_POINT('Ctrl Pts',(20.1,40.8749138146613,41.1621829179885)) ;
#14798=CARTESIAN_POINT('Ctrl Pts',(20.1,40.910118556837,41.1277159927359)) ;
#14799=CARTESIAN_POINT('Ctrl Pts',(20.1,40.9438718690891,41.091885062196)) ;
#14800=CARTESIAN_POINT('Ctrl Pts',(20.1,40.9760625743085,41.0547102740498)) ;
#14801=CARTESIAN_POINT('Ctrl Pts',(20.1,41.0231100315383,41.0003784648081)) ;
#14802=CARTESIAN_POINT('Ctrl Pts',(20.1,41.0668218688122,40.943176514036)) ;
#14803=CARTESIAN_POINT('Ctrl Pts',(20.1,41.10711615432,40.8834720571114)) ;
#14804=CARTESIAN_POINT('Ctrl Pts',(20.1,41.1273251615833,40.8535281633699)) ;
#14805=CARTESIAN_POINT('Ctrl Pts',(20.1,41.1466737625269,40.822954478093)) ;
#14806=CARTESIAN_POINT('Ctrl Pts',(20.1,41.1651469177346,40.7917962001638)) ;
#14807=CARTESIAN_POINT('Ctrl Pts',(20.1,41.1726171516231,40.7791963155703)) ;
#14808=CARTESIAN_POINT('Ctrl Pts',(20.1,41.1799453503731,40.7664987577444)) ;
#14809=CARTESIAN_POINT('Ctrl Pts',(20.1,41.1871266089476,40.7537132305828)) ;
#14810=CARTESIAN_POINT('Ctrl Pts',(20.1,41.2220665911135,40.6915060162942)) ;
#14811=CARTESIAN_POINT('Ctrl Pts',(20.1,41.25346410526,40.6273417786838)) ;
#14812=CARTESIAN_POINT('Ctrl Pts',(20.1,41.2812451501811,40.5615844124439)) ;
#14813=CARTESIAN_POINT('Ctrl Pts',(20.1,41.3017750166453,40.512990489797)) ;
#14814=CARTESIAN_POINT('Ctrl Pts',(20.1,41.3203288925696,40.4635259999673)) ;
#14815=CARTESIAN_POINT('Ctrl Pts',(20.1,41.3368587922048,40.413335412753)) ;
#14816=CARTESIAN_POINT('Ctrl Pts',(20.1,41.345542673033,40.3869680973014)) ;
#14817=CARTESIAN_POINT('Ctrl Pts',(20.1,41.3536677048483,40.3604003853126)) ;
#14818=CARTESIAN_POINT('Ctrl Pts',(20.1,41.3612251844057,40.333653400688)) ;
#14819=CARTESIAN_POINT('Ctrl Pts',(20.1,41.3646856421227,40.3214063534219)) ;
#14820=CARTESIAN_POINT('Ctrl Pts',(20.1,41.3680270907377,40.3091217232312)) ;
#14821=CARTESIAN_POINT('Ctrl Pts',(20.1,41.3712486093269,40.2968015581035)) ;
#14822=CARTESIAN_POINT('Ctrl Pts',(20.1,41.3743356306514,40.2849957555236)) ;
#14823=CARTESIAN_POINT('Ctrl Pts',(20.1,41.3773099420866,40.2731672101754)) ;
#14824=CARTESIAN_POINT('Ctrl Pts',(20.1,41.3801712759402,40.2613177481751)) ;
#14825=CARTESIAN_POINT('Ctrl Pts',(20.1,41.3965090601543,40.193659109539)) ;
#14826=CARTESIAN_POINT('Ctrl Pts',(20.1,41.4091677309796,40.1253186782015)) ;
#14827=CARTESIAN_POINT('Ctrl Pts',(20.1,41.4180675225836,40.056631121656)) ;
#14828=CARTESIAN_POINT('Ctrl Pts',(20.1,41.4267500723293,39.9896202125065)) ;
#14829=CARTESIAN_POINT('Ctrl Pts',(20.1,41.4318548797362,39.922277949119)) ;
#14830=CARTESIAN_POINT('Ctrl Pts',(20.1,41.4332596199026,39.8549209631959)) ;
#14831=CARTESIAN_POINT('Ctrl Pts',(20.1,41.4341904769168,39.8102865715126)) ;
#14832=CARTESIAN_POINT('Ctrl Pts',(20.1,41.433495615042,39.7656458625524)) ;
#14833=CARTESIAN_POINT('Ctrl Pts',(20.1,41.4311276841363,39.7210954770712)) ;
#14834=CARTESIAN_POINT('Ctrl Pts',(20.1,41.4290930699883,39.6828161318511)) ;
#14835=CARTESIAN_POINT('Ctrl Pts',(20.1,41.4258231001969,39.6446034913311)) ;
#14836=CARTESIAN_POINT('Ctrl Pts',(20.1,41.4212821252632,39.606522140799)) ;
#14837=CARTESIAN_POINT('Ctrl Pts',(20.1,41.4199698659409,39.5955173217966)) ;
#14838=CARTESIAN_POINT('Ctrl Pts',(20.1,41.4185516770161,39.5845261308585)) ;
#14839=CARTESIAN_POINT('Ctrl Pts',(20.1,41.4170284226326,39.5735605724709)) ;
#14840=CARTESIAN_POINT('Ctrl Pts',(20.1,41.4080640020682,39.5090277681156)) ;
#14841=CARTESIAN_POINT('Ctrl Pts',(20.1,41.3954525129461,39.445276444527)) ;
#14842=CARTESIAN_POINT('Ctrl Pts',(20.1,41.379089864571,39.3825977231924)) ;
#14843=CARTESIAN_POINT('Ctrl Pts',(20.1,41.3742617457321,39.3641031428327)) ;
#14844=CARTESIAN_POINT('Ctrl Pts',(20.1,41.3691067076579,39.3457020687507)) ;
#14845=CARTESIAN_POINT('Ctrl Pts',(20.1,41.3636212695664,39.3274023311227)) ;
#14846=CARTESIAN_POINT('Ctrl Pts',(20.1,41.3437063393713,39.26096497619)) ;
#14847=CARTESIAN_POINT('Ctrl Pts',(20.1,41.3194401862383,39.1958601556226)) ;
#14848=CARTESIAN_POINT('Ctrl Pts',(20.1,41.2910929607224,39.1323838710923)) ;
#14849=CARTESIAN_POINT('Ctrl Pts',(20.1,41.2781499478771,39.1034013392539)) ;
#14850=CARTESIAN_POINT('Ctrl Pts',(20.1,41.2643554850943,39.0747588764659)) ;
#14851=CARTESIAN_POINT('Ctrl Pts',(20.1,41.2497324379344,39.0464878757334)) ;
#14852=CARTESIAN_POINT('Ctrl Pts',(20.1,41.2363854250346,39.0206838550432)) ;
#14853=CARTESIAN_POINT('Ctrl Pts',(20.1,41.2223480942368,38.9951893103491)) ;
#14854=CARTESIAN_POINT('Ctrl Pts',(20.1,41.2076368596568,38.9700298460359)) ;
#14855=CARTESIAN_POINT('Ctrl Pts',(20.1,41.2020737310709,38.9605156659469)) ;
#14856=CARTESIAN_POINT('Ctrl Pts',(20.1,41.1964186186447,38.9510569671551)) ;
#14857=CARTESIAN_POINT('Ctrl Pts',(20.1,41.1906742072217,38.9416571161833)) ;
#14858=CARTESIAN_POINT('Ctrl Pts',(20.1,41.1568739608253,38.886348181022)) ;
#14859=CARTESIAN_POINT('Ctrl Pts',(20.1,41.1199697709051,38.8330473189996)) ;
#14860=CARTESIAN_POINT('Ctrl Pts',(20.1,41.0802042130272,38.7819809617283)) ;
#14861=CARTESIAN_POINT('Ctrl Pts',(20.1,41.0406084383323,38.7311326375777)) ;
#14862=CARTESIAN_POINT('Ctrl Pts',(20.1,40.9981747532311,38.6824991338018)) ;
#14863=CARTESIAN_POINT('Ctrl Pts',(20.1,40.9531114790019,38.6363446012905)) ;
#14864=CARTESIAN_POINT('Ctrl Pts',(20.1,40.9089802289544,38.5911446629832)) ;
#14865=CARTESIAN_POINT('Ctrl Pts',(20.1,40.8623261731692,38.5483217771446)) ;
#14866=CARTESIAN_POINT('Ctrl Pts',(20.1,40.8133282868011,38.5081708244776)) ;
#14867=CARTESIAN_POINT('Ctrl Pts',(20.1,40.8047841243671,38.5011693742745)) ;
#14868=CARTESIAN_POINT('Ctrl Pts',(20.1,40.7961686677144,38.4942492979095)) ;
#14869=CARTESIAN_POINT('Ctrl Pts',(20.1,40.7874828419659,38.4874123235512)) ;
#14870=CARTESIAN_POINT('Ctrl Pts',(20.1,40.7782551910926,38.4801488561234)) ;
#14871=CARTESIAN_POINT('Ctrl Pts',(20.1,40.7689549068099,38.4729845740318)) ;
#14872=CARTESIAN_POINT('Ctrl Pts',(20.1,40.7595878194887,38.4659243469758)) ;
#14873=CARTESIAN_POINT('Ctrl Pts',(20.1,40.7100628332441,38.4285960253916)) ;
#14874=CARTESIAN_POINT('Ctrl Pts',(20.1,40.6586327257531,38.3941416234219)) ;
#14875=CARTESIAN_POINT('Ctrl Pts',(20.1,40.6054916711262,38.3627919275834)) ;
#14876=CARTESIAN_POINT('Ctrl Pts',(20.1,40.5533162503354,38.3320118916297)) ;
#14877=CARTESIAN_POINT('Ctrl Pts',(20.1,40.4994906913971,38.3042243928691)) ;
#14878=CARTESIAN_POINT('Ctrl Pts',(20.1,40.4441860769283,38.2796959625828)) ;
#14879=CARTESIAN_POINT('Ctrl Pts',(20.1,40.3906414806518,38.2559481268986)) ;
#14880=CARTESIAN_POINT('Ctrl Pts',(20.1,40.3357098152915,38.2352550726404)) ;
#14881=CARTESIAN_POINT('Ctrl Pts',(20.1,40.2795449025621,38.2179077161054)) ;
#14882=CARTESIAN_POINT('Ctrl Pts',(20.1,40.2668745968585,38.2139943064735)) ;
#14883=CARTESIAN_POINT('Ctrl Pts',(20.1,40.2541415454427,38.2102513721407)) ;
#14884=CARTESIAN_POINT('Ctrl Pts',(20.1,40.2413475545766,38.2066826248723)) ;
#14885=CARTESIAN_POINT('Ctrl Pts',(29.6300740822721,38.2459897433641,40.3279613528596)) ;
#14886=CARTESIAN_POINT('Ctrl Pts',(29.5931358106354,38.4733801681185,40.7908635031756)) ;
#14887=CARTESIAN_POINT('Ctrl Pts',(29.5192592673619,39.4210811034059,41.4647659628203)) ;
#14888=CARTESIAN_POINT('Ctrl Pts',(29.4084444524518,41.0530787209739,40.8197841334159)) ;
#14889=CARTESIAN_POINT('Ctrl Pts',(29.2976296375416,41.3968998908732,39.1007906955674)) ;
#14890=CARTESIAN_POINT('Ctrl Pts',(29.1868148226315,40.1448501483431,37.8755725352669)) ;
#14891=CARTESIAN_POINT('Ctrl Pts',(29.0760000077214,38.4342400021641,38.2582535083027)) ;
#14892=CARTESIAN_POINT('Ctrl Pts',(28.9651851928112,37.8237840021384,39.9011087585314)) ;
#14893=CARTESIAN_POINT('Ctrl Pts',(28.8543703779011,38.8686165906699,41.3080694099963)) ;
#14894=CARTESIAN_POINT('Ctrl Pts',(28.7435555629909,40.617802981239,41.1983492914825)) ;
#14895=CARTESIAN_POINT('Ctrl Pts',(28.6327407480808,41.4786453053513,39.671756482491)) ;
#14896=CARTESIAN_POINT('Ctrl Pts',(28.5219259331707,40.6674772372708,38.1182099023464)) ;
#14897=CARTESIAN_POINT('Ctrl Pts',(28.4111111182605,38.9227802986979,37.9521038579512)) ;
#14898=CARTESIAN_POINT('Ctrl Pts',(28.3002963033504,37.8330223043396,39.324679226451)) ;
#14899=CARTESIAN_POINT('Ctrl Pts',(28.1894814884402,38.3903556961656,40.9862787943451)) ;
#14900=CARTESIAN_POINT('Ctrl Pts',(28.0786666735301,40.0873652411245,41.4241133393722)) ;
#14901=CARTESIAN_POINT('Ctrl Pts',(27.96785185862,41.3790176807763,40.2395580544964)) ;
#14902=CARTESIAN_POINT('Ctrl Pts',(27.8570370437098,41.0893382026773,38.5110838439939)) ;
#14903=CARTESIAN_POINT('Ctrl Pts',(27.7462222287997,39.4820628559708,37.812367849582)) ;
#14904=CARTESIAN_POINT('Ctrl Pts',(27.6354074138896,38.02052476931,38.7795514216669)) ;
#14905=CARTESIAN_POINT('Ctrl Pts',(27.5245925989794,38.0353711001173,40.5320688312148)) ;
#14906=CARTESIAN_POINT('Ctrl Pts',(27.4137777840693,39.5130851891104,41.4743526749128)) ;
#14907=CARTESIAN_POINT('Ctrl Pts',(27.3029629691591,41.1082923469922,40.7485070740931)) ;
#14908=CARTESIAN_POINT('Ctrl Pts',(27.192148154249,41.3686471870141,39.0153731842676)) ;
#14909=CARTESIAN_POINT('Ctrl Pts',(27.0813333393388,40.0571114221001,37.8528708534111)) ;
#14910=CARTESIAN_POINT('Ctrl Pts',(26.9705185244287,38.367763791755,38.3193923515952)) ;
#14911=CARTESIAN_POINT('Ctrl Pts',(26.8597037095185,37.8386592473608,39.9901963817902)) ;
#14912=CARTESIAN_POINT('Ctrl Pts',(26.7488888946085,38.9515173907173,41.3441108842142)) ;
#14913=CARTESIAN_POINT('Ctrl Pts',(26.6380740796983,40.6931441635229,41.1484736934281)) ;
#14914=CARTESIAN_POINT('Ctrl Pts',(26.5272592647882,41.4778874257816,39.5814013470451)) ;
#14915=CARTESIAN_POINT('Ctrl Pts',(26.416444449878,40.5912830608963,38.0696241059467)) ;
#14916=CARTESIAN_POINT('Ctrl Pts',(26.3056296349679,38.8405339270694,37.9895291820938)) ;
#14917=CARTESIAN_POINT('Ctrl Pts',(26.1948148200577,37.8195975555487,39.4140384490947)) ;
#14918=CARTESIAN_POINT('Ctrl Pts',(26.0840000051476,38.4579784578276,41.0462172230273)) ;
#14919=CARTESIAN_POINT('Ctrl Pts',(25.9731851902374,40.1744671234318,41.4000595428663)) ;
#14920=CARTESIAN_POINT('Ctrl Pts',(25.8623703753273,41.4062982291994,40.1534120973844)) ;
#14921=CARTESIAN_POINT('Ctrl Pts',(25.7515555604172,41.0319596004962,38.4412764960012)) ;
#14922=CARTESIAN_POINT('Ctrl Pts',(25.640740745507,39.392265272267,37.822454844445)) ;
#14923=CARTESIAN_POINT('Ctrl Pts',(25.5299259305969,37.9800636903518,38.8603490676194)) ;
#14924=CARTESIAN_POINT('Ctrl Pts',(25.4191111156867,38.0810840912803,40.6100154944158)) ;
#14925=CARTESIAN_POINT('Ctrl Pts',(25.3082963007766,39.6033531444577,41.4784823367307)) ;
#14926=CARTESIAN_POINT('Ctrl Pts',(25.1974814858665,41.1609314396763,40.6750599193646)) ;
#14927=CARTESIAN_POINT('Ctrl Pts',(25.0866666709563,41.3357325096837,38.9312186673045)) ;
#14928=CARTESIAN_POINT('Ctrl Pts',(24.9758518560461,39.9686099201725,37.8346268783008)) ;
#14929=CARTESIAN_POINT('Ctrl Pts',(24.8650370411361,38.304251048472,38.3836690193557)) ;
#14930=CARTESIAN_POINT('Ctrl Pts',(24.7542222262259,37.8579600047224,40.0784734419163)) ;
#14931=CARTESIAN_POINT('Ctrl Pts',(24.6434074113158,39.0360594062455,41.3760170930483)) ;
#14932=CARTESIAN_POINT('Ctrl Pts',(24.5325925964056,40.7659567397109,41.0949602622614)) ;
#14933=CARTESIAN_POINT('Ctrl Pts',(24.4217777814955,41.4726788523376,39.4911892118972)) ;
#14934=CARTESIAN_POINT('Ctrl Pts',(24.3109629665853,40.5127954478126,38.0248462860509)) ;
#14935=CARTESIAN_POINT('Ctrl Pts',(24.2001481516752,38.7602257828917,38.0309533361934)) ;
#14936=CARTESIAN_POINT('Ctrl Pts',(24.0893333367651,37.8105848789005,39.5039502404432)) ;
#14937=CARTESIAN_POINT('Ctrl Pts',(23.9785185218549,38.5284667782912,41.102757078366)) ;
#14938=CARTESIAN_POINT('Ctrl Pts',(23.8677037069448,40.2602808334951,41.3717511390089)) ;
#14939=CARTESIAN_POINT('Ctrl Pts',(23.7568888920346,41.4293088255812,40.0660286263046)) ;
#14940=CARTESIAN_POINT('Ctrl Pts',(23.6460740771245,40.9712172436731,38.3743756391225)) ;
#14941=CARTESIAN_POINT('Ctrl Pts',(23.5352592622143,39.3030724240549,37.8369460276841)) ;
#14942=CARTESIAN_POINT('Ctrl Pts',(23.4244444473042,37.9436253671659,38.9430388926739)) ;
#14943=CARTESIAN_POINT('Ctrl Pts',(23.3136296323941,38.1305753143352,40.6856195776569)) ;
#14944=CARTESIAN_POINT('Ctrl Pts',(23.2028148174839,39.6937149694595,41.4781674595636)) ;
#14945=CARTESIAN_POINT('Ctrl Pts',(23.0920000025738,41.2098945632884,40.5991127594935)) ;
#14946=CARTESIAN_POINT('Ctrl Pts',(22.9811851876637,41.2987187921716,38.848784795215)) ;
#14947=CARTESIAN_POINT('Ctrl Pts',(22.8703703727535,39.8793182464488,37.8207576467842)) ;
#14948=CARTESIAN_POINT('Ctrl Pts',(22.7595555578434,38.2439764102052,38.4509915754534)) ;
#14949=CARTESIAN_POINT('Ctrl Pts',(22.6487407429332,37.8815790320852,40.1656944257316)) ;
#14950=CARTESIAN_POINT('Ctrl Pts',(22.5379259280231,39.122068318894,41.4037267602073)) ;
#14951=CARTESIAN_POINT('Ctrl Pts',(22.427111113113,40.8360493115319,41.037930533244)) ;
#14952=CARTESIAN_POINT('Ctrl Pts',(22.3162962982028,41.4630397864066,39.4013424185359)) ;
#14953=CARTESIAN_POINT('Ctrl Pts',(22.2054814832927,40.432200557639,37.9839828116129)) ;
#14954=CARTESIAN_POINT('Ctrl Pts',(22.0946666683825,38.682052148795,38.0762770764856)) ;
#14955=CARTESIAN_POINT('Ctrl Pts',(21.9838518534724,37.806005117906,39.594196455287)) ;
#14956=CARTESIAN_POINT('Ctrl Pts',(21.8730370385622,38.6016505653522,41.1557618246954)) ;
#14957=CARTESIAN_POINT('Ctrl Pts',(21.7622222236521,40.3445983661982,41.3392564020827)) ;
#14958=CARTESIAN_POINT('Ctrl Pts',(21.6514074087419,41.4479940364311,39.977619430384)) ;
#14959=CARTESIAN_POINT('Ctrl Pts',(21.5405925938318,40.9072578085518,38.3105427025879)) ;
#14960=CARTESIAN_POINT('Ctrl Pts',(21.4297777789217,39.2147007747696,37.8558072618482)) ;
#14961=CARTESIAN_POINT('Ctrl Pts',(21.3189629640115,37.9112968612974,39.0274189154373)) ;
#14962=CARTESIAN_POINT('Ctrl Pts',(21.2081481491014,38.1837272212218,40.7587017705598)) ;
#14963=CARTESIAN_POINT('Ctrl Pts',(21.0973333341912,39.7839475036059,41.4734014691738)) ;
#14964=CARTESIAN_POINT('Ctrl Pts',(20.9865185192811,41.2550721079325,40.520864063088)) ;
#14965=CARTESIAN_POINT('Ctrl Pts',(20.875703704371,41.257677850447,38.7682418152935)) ;
#14966=CARTESIAN_POINT('Ctrl Pts',(20.7648888894608,39.7894880096876,37.8113551948838)) ;
#14967=CARTESIAN_POINT('Ctrl Pts',(20.6540740745507,38.1870148554998,38.5210802763619)) ;
#14968=CARTESIAN_POINT('Ctrl Pts',(20.5432592596406,37.9096008119324,40.25188160747)) ;
#14969=CARTESIAN_POINT('Ctrl Pts',(20.4324444447304,39.209052927568,41.4267059761609)) ;
#14970=CARTESIAN_POINT('Ctrl Pts',(20.3216296298203,40.9038184910527,40.9784637190458)) ;
#14971=CARTESIAN_POINT('Ctrl Pts',(20.2108148149101,41.4478477610965,39.3100962723047)) ;
#14972=CARTESIAN_POINT('Ctrl Pts',(20.1369382716367,40.7172822611094,38.4053556254406)) ;
#14973=CARTESIAN_POINT('Ctrl Pts',(20.1,40.2413475545766,38.2066826248723)) ;
#14974=CARTESIAN_POINT('Ctrl Pts',(29.5533827215147,38.1267645996105,40.3865280630401)) ;
#14975=CARTESIAN_POINT('Ctrl Pts',(29.516444449878,38.3735732359292,40.8889601623331)) ;
#14976=CARTESIAN_POINT('Ctrl Pts',(29.4425679066046,39.402203952147,41.6204111337465)) ;
#14977=CARTESIAN_POINT('Ctrl Pts',(29.3317530916944,41.1735674864837,40.9203504960237)) ;
#14978=CARTESIAN_POINT('Ctrl Pts',(29.2209382767843,41.5467495770312,39.0545620544289)) ;
#14979=CARTESIAN_POINT('Ctrl Pts',(29.1101234618742,40.1877799111328,37.7247152780606)) ;
#14980=CARTESIAN_POINT('Ctrl Pts',(28.999308646964,38.3310906600031,38.1400756398793)) ;
#14981=CARTESIAN_POINT('Ctrl Pts',(28.8884938320539,37.6685042161736,39.9232240042654)) ;
#14982=CARTESIAN_POINT('Ctrl Pts',(28.7776790171437,38.8025612312625,41.4503333366708)) ;
#14983=CARTESIAN_POINT('Ctrl Pts',(28.6668642022336,40.7011209801604,41.3312435691208)) ;
#14984=CARTESIAN_POINT('Ctrl Pts',(28.5560493873234,41.6354757153215,39.6742859825908)) ;
#14985=CARTESIAN_POINT('Ctrl Pts',(28.4452345724133,40.7550372143405,37.9880728831733)) ;
#14986=CARTESIAN_POINT('Ctrl Pts',(28.3344197575032,38.8613502982639,37.8077820624592)) ;
#14987=CARTESIAN_POINT('Ctrl Pts',(28.223604942593,37.6785314315704,39.2975697494733)) ;
#14988=CARTESIAN_POINT('Ctrl Pts',(28.1127901276829,38.283458813891,41.101063119533)) ;
#14989=CARTESIAN_POINT('Ctrl Pts',(28.0019753127728,40.1253860281235,41.5762869426473)) ;
#14990=CARTESIAN_POINT('Ctrl Pts',(27.8911604978626,41.5273402993839,40.2905754848318)) ;
#14991=CARTESIAN_POINT('Ctrl Pts',(27.7803456829525,41.2129233795143,38.4144966514031)) ;
#14992=CARTESIAN_POINT('Ctrl Pts',(27.6695308680423,39.4683932967824,37.6561131709153)) ;
#14993=CARTESIAN_POINT('Ctrl Pts',(27.5587160531322,37.8820458396011,38.7058902613705)) ;
#14994=CARTESIAN_POINT('Ctrl Pts',(27.4479012382221,37.8981599862932,40.6080654846344)) ;
#14995=CARTESIAN_POINT('Ctrl Pts',(27.3370864233119,39.5020648101976,41.6308165118133)) ;
#14996=CARTESIAN_POINT('Ctrl Pts',(27.2262716084018,41.2334961301744,40.842986667572)) ;
#14997=CARTESIAN_POINT('Ctrl Pts',(27.1154567934916,41.5160842079009,38.9618502372781)) ;
#14998=CARTESIAN_POINT('Ctrl Pts',(27.0046419785815,40.0925486567836,37.7000749654925)) ;
#14999=CARTESIAN_POINT('Ctrl Pts',(26.8938271636713,38.2589376533124,38.2064354901474)) ;
#15000=CARTESIAN_POINT('Ctrl Pts',(26.7830123487612,37.6846497464535,40.0199193459146)) ;
#15001=CARTESIAN_POINT('Ctrl Pts',(26.6721975338511,38.8925414203207,41.489452605269)) ;
#15002=CARTESIAN_POINT('Ctrl Pts',(26.5613827189409,40.7828959910397,41.2771087991335)) ;
#15003=CARTESIAN_POINT('Ctrl Pts',(26.4505679040308,41.6346531159385,39.5762148884017)) ;
#15004=CARTESIAN_POINT('Ctrl Pts',(26.3397530891207,40.6723363671666,37.9353380586228)) ;
#15005=CARTESIAN_POINT('Ctrl Pts',(26.2289382742105,38.7720804231329,37.8484033561016)) ;
#15006=CARTESIAN_POINT('Ctrl Pts',(26.1181234593004,37.6639602641803,39.3945598839832)) ;
#15007=CARTESIAN_POINT('Ctrl Pts',(26.0073086443902,38.3568562826186,41.1661200446965)) ;
#15008=CARTESIAN_POINT('Ctrl Pts',(25.8964938294801,40.2199260546718,41.5501790503721)) ;
#15009=CARTESIAN_POINT('Ctrl Pts',(25.78567901457,41.5569504949829,40.197073015578)) ;
#15010=CARTESIAN_POINT('Ctrl Pts',(25.6748641996598,41.1506448795578,38.3387280416135)) ;
#15011=CARTESIAN_POINT('Ctrl Pts',(25.5640493847497,39.3709273669721,37.6670615538535)) ;
#15012=CARTESIAN_POINT('Ctrl Pts',(25.4532345698395,37.8381295501071,38.7935876955824)) ;
#15013=CARTESIAN_POINT('Ctrl Pts',(25.3424197549294,37.9477766797981,40.6926684738367)) ;
#15014=CARTESIAN_POINT('Ctrl Pts',(25.2316049400192,39.6000412794646,41.6352988298477)) ;
#15015=CARTESIAN_POINT('Ctrl Pts',(25.1207901251091,41.2906303859217,40.7632674264492)) ;
#15016=CARTESIAN_POINT('Ctrl Pts',(25.009975310199,41.4803587518464,38.8705092690112)) ;
#15017=CARTESIAN_POINT('Ctrl Pts',(24.8991604952888,39.9964894888283,37.6802730295803)) ;
#15018=CARTESIAN_POINT('Ctrl Pts',(24.7883456803787,38.1900011817109,38.27620112225)) ;
#15019=CARTESIAN_POINT('Ctrl Pts',(24.6775308654686,37.7055987094957,40.1157349056572)) ;
#15020=CARTESIAN_POINT('Ctrl Pts',(24.5667160505584,38.9843029779442,41.5240834737454)) ;
#15021=CARTESIAN_POINT('Ctrl Pts',(24.4559012356483,40.861926463212,41.2190255399759)) ;
#15022=CARTESIAN_POINT('Ctrl Pts',(24.3450864207381,41.6289997516412,39.4782990061507)) ;
#15023=CARTESIAN_POINT('Ctrl Pts',(24.234271605828,40.5871462331756,37.8867363961837)) ;
#15024=CARTESIAN_POINT('Ctrl Pts',(24.1234567909179,38.6849142921439,37.8933649634122)) ;
#15025=CARTESIAN_POINT('Ctrl Pts',(24.0126419760077,37.6541779418353,39.4921497743036)) ;
#15026=CARTESIAN_POINT('Ctrl Pts',(23.9018271610976,38.4333640171409,41.2274881722633)) ;
#15027=CARTESIAN_POINT('Ctrl Pts',(23.7910123461874,40.3130679043387,41.5194532246915)) ;
#15028=CARTESIAN_POINT('Ctrl Pts',(23.6801975312773,41.5819261021132,40.1022273537289)) ;
#15029=CARTESIAN_POINT('Ctrl Pts',(23.5693827163671,41.0847153740808,38.2661141253828)) ;
#15030=CARTESIAN_POINT('Ctrl Pts',(23.4585679014571,39.2741178145893,37.6827902248286)) ;
#15031=CARTESIAN_POINT('Ctrl Pts',(23.3477530865468,37.7985795432634,38.8833388932469)) ;
#15032=CARTESIAN_POINT('Ctrl Pts',(23.2369382716368,38.0014942507341,40.7747288363389)) ;
#15033=CARTESIAN_POINT('Ctrl Pts',(23.1261234567265,39.6981196344702,41.6349570634594)) ;
#15034=CARTESIAN_POINT('Ctrl Pts',(23.0153086418165,41.343774759884,40.6808346899769)) ;
#15035=CARTESIAN_POINT('Ctrl Pts',(22.9044938269063,41.440184214356,38.7810358816474)) ;
#15036=CARTESIAN_POINT('Ctrl Pts',(22.7936790119962,39.8995726716397,37.665219422459)) ;
#15037=CARTESIAN_POINT('Ctrl Pts',(22.682864197086,38.1245793360405,38.349272749087)) ;
#15038=CARTESIAN_POINT('Ctrl Pts',(22.5720493821759,37.7312347051225,40.2104042044945)) ;
#15039=CARTESIAN_POINT('Ctrl Pts',(22.4612345672658,39.0776566996982,41.5541594330641)) ;
#15040=CARTESIAN_POINT('Ctrl Pts',(22.3504197523556,40.9380046537774,41.1571257055231)) ;
#15041=CARTESIAN_POINT('Ctrl Pts',(22.2396049374455,41.6185375489323,39.3807796643797)) ;
#15042=CARTESIAN_POINT('Ctrl Pts',(22.1287901225353,40.4996688692564,37.842383348283)) ;
#15043=CARTESIAN_POINT('Ctrl Pts',(22.0179753076252,38.6000649496604,37.942559165615)) ;
#15044=CARTESIAN_POINT('Ctrl Pts',(21.907160492715,37.6492070879968,39.5901026465171)) ;
#15045=CARTESIAN_POINT('Ctrl Pts',(21.7963456778049,38.5127974000755,41.2850193069807)) ;
#15046=CARTESIAN_POINT('Ctrl Pts',(21.6855308628947,40.4045858092226,41.484183570233)) ;
#15047=CARTESIAN_POINT('Ctrl Pts',(21.5747160479846,41.6022069534912,40.0062683743358)) ;
#15048=CARTESIAN_POINT('Ctrl Pts',(21.4639012330745,41.0152940649862,38.1968301173366)) ;
#15049=CARTESIAN_POINT('Ctrl Pts',(21.3530864181643,39.1781995881605,37.7032621311913)) ;
#15050=CARTESIAN_POINT('Ctrl Pts',(21.2422716032542,37.7634903153144,38.9749246245865)) ;
#15051=CARTESIAN_POINT('Ctrl Pts',(21.131456788344,38.0591851129179,40.8540519493901)) ;
#15052=CARTESIAN_POINT('Ctrl Pts',(21.0206419734339,39.7960576577108,41.6297840769974)) ;
#15053=CARTESIAN_POINT('Ctrl Pts',(20.9098271585238,41.3928102819289,40.5959038751708)) ;
#15054=CARTESIAN_POINT('Ctrl Pts',(20.7990123436136,41.3956385441889,38.6936148609031)) ;
#15055=CARTESIAN_POINT('Ctrl Pts',(20.6881975287035,39.8020713003344,37.6550140396507)) ;
#15056=CARTESIAN_POINT('Ctrl Pts',(20.5773827137934,38.062753497707,38.4253467381798)) ;
#15057=CARTESIAN_POINT('Ctrl Pts',(20.4665678988832,37.7616494302755,40.303951418789)) ;
#15058=CARTESIAN_POINT('Ctrl Pts',(20.3557530839731,39.1720694379247,41.579100980006)) ;
#15059=CARTESIAN_POINT('Ctrl Pts',(20.2449382690629,41.0115610438497,41.0925806687903)) ;
#15060=CARTESIAN_POINT('Ctrl Pts',(20.1341234541528,41.6020481868418,39.2817414707311)) ;
#15061=CARTESIAN_POINT('Ctrl Pts',(20.0602469108794,40.8090953833627,38.2997396757312)) ;
#15062=CARTESIAN_POINT('Ctrl Pts',(20.0233086392427,40.2925178008944,38.0841008140837)) ;
#15063=CARTESIAN_POINT('Ctrl Pts',(29.4766913607574,38.0075394558569,40.4450947732207)) ;
#15064=CARTESIAN_POINT('Ctrl Pts',(29.4397530891207,38.2737663037398,40.9870568214907)) ;
#15065=CARTESIAN_POINT('Ctrl Pts',(29.3658765458472,39.3833268008881,41.7760563046727)) ;
#15066=CARTESIAN_POINT('Ctrl Pts',(29.2550617309371,41.2940562519934,41.0209168586316)) ;
#15067=CARTESIAN_POINT('Ctrl Pts',(29.1442469160269,41.6965992631892,39.0083334132903)) ;
#15068=CARTESIAN_POINT('Ctrl Pts',(29.0334321011168,40.2307096739224,37.5738580208544)) ;
#15069=CARTESIAN_POINT('Ctrl Pts',(28.9226172862067,38.2279413178422,38.0218977714557)) ;
#15070=CARTESIAN_POINT('Ctrl Pts',(28.8118024712965,37.5132244302088,39.9453392499995)) ;
#15071=CARTESIAN_POINT('Ctrl Pts',(28.7009876563864,38.7365058718551,41.5925972633453)) ;
#15072=CARTESIAN_POINT('Ctrl Pts',(28.5901728414763,40.7844389790819,41.4641378467591)) ;
#15073=CARTESIAN_POINT('Ctrl Pts',(28.4793580265661,41.7923061252916,39.6768154826907)) ;
#15074=CARTESIAN_POINT('Ctrl Pts',(28.368543211656,40.8425971914102,37.8579358640001)) ;
#15075=CARTESIAN_POINT('Ctrl Pts',(28.2577283967458,38.7999202978298,37.6634602669672)) ;
#15076=CARTESIAN_POINT('Ctrl Pts',(28.1469135818357,37.5240405588012,39.2704602724957)) ;
#15077=CARTESIAN_POINT('Ctrl Pts',(28.0360987669255,38.1765619316163,41.215847444721)) ;
#15078=CARTESIAN_POINT('Ctrl Pts',(27.9252839520154,40.1634068151226,41.7284605459223)) ;
#15079=CARTESIAN_POINT('Ctrl Pts',(27.8144691371052,41.6756629179915,40.3415929151672)) ;
#15080=CARTESIAN_POINT('Ctrl Pts',(27.7036543221951,41.3365085563514,38.3179094588122)) ;
#15081=CARTESIAN_POINT('Ctrl Pts',(27.592839507285,39.4547237375941,37.4998584922485)) ;
#15082=CARTESIAN_POINT('Ctrl Pts',(27.4820246923748,37.7435669098921,38.6322291010743)) ;
#15083=CARTESIAN_POINT('Ctrl Pts',(27.3712098774647,37.7609488724691,40.6840621380539)) ;
#15084=CARTESIAN_POINT('Ctrl Pts',(27.2603950625546,39.4910444312848,41.7872803487137)) ;
#15085=CARTESIAN_POINT('Ctrl Pts',(27.1495802476444,41.3586999133566,40.9374662610509)) ;
#15086=CARTESIAN_POINT('Ctrl Pts',(27.0387654327343,41.6635212287878,38.9083272902888)) ;
#15087=CARTESIAN_POINT('Ctrl Pts',(26.9279506178241,40.127985891467,37.5472790775738)) ;
#15088=CARTESIAN_POINT('Ctrl Pts',(26.817135802914,38.1501115148698,38.0934786286996)) ;
#15089=CARTESIAN_POINT('Ctrl Pts',(26.7063209880039,37.5306402455464,40.049642310039)) ;
#15090=CARTESIAN_POINT('Ctrl Pts',(26.5955061730937,38.833565449924,41.6347943263239)) ;
#15091=CARTESIAN_POINT('Ctrl Pts',(26.4846913581836,40.8726478185564,41.4057439048389)) ;
#15092=CARTESIAN_POINT('Ctrl Pts',(26.3738765432735,41.7914188060955,39.5710284297584)) ;
#15093=CARTESIAN_POINT('Ctrl Pts',(26.2630617283633,40.7533896734369,37.8010520112989)) ;
#15094=CARTESIAN_POINT('Ctrl Pts',(26.1522469134532,38.7036269191965,37.7072775301095)) ;
#15095=CARTESIAN_POINT('Ctrl Pts',(26.041432098543,37.5083229728118,39.3750813188718)) ;
#15096=CARTESIAN_POINT('Ctrl Pts',(25.9306172836329,38.2557341074098,41.2860228663657)) ;
#15097=CARTESIAN_POINT('Ctrl Pts',(25.8198024687227,40.2653849859115,41.7002985578778)) ;
#15098=CARTESIAN_POINT('Ctrl Pts',(25.7089876538126,41.7076027607666,40.2407339337718)) ;
#15099=CARTESIAN_POINT('Ctrl Pts',(25.5981728389025,41.2693301586193,38.2361795872257)) ;
#15100=CARTESIAN_POINT('Ctrl Pts',(25.4873580239923,39.3495894616773,37.5116682632619)) ;
#15101=CARTESIAN_POINT('Ctrl Pts',(25.3765432090822,37.6961954098625,38.7268263235454)) ;
#15102=CARTESIAN_POINT('Ctrl Pts',(25.265728394172,37.8144692683159,40.7753214532577)) ;
#15103=CARTESIAN_POINT('Ctrl Pts',(25.1549135792619,39.5967294144714,41.7921153229646)) ;
#15104=CARTESIAN_POINT('Ctrl Pts',(25.0440987643517,41.4203293321672,40.8514749335338)) ;
#15105=CARTESIAN_POINT('Ctrl Pts',(24.9332839494416,41.6249849940091,38.8097998707178)) ;
#15106=CARTESIAN_POINT('Ctrl Pts',(24.8224691345314,40.0243690574841,37.52591918086)) ;
#15107=CARTESIAN_POINT('Ctrl Pts',(24.7116543196214,38.0757513149498,38.1687332251443)) ;
#15108=CARTESIAN_POINT('Ctrl Pts',(24.6008395047112,37.5532374142691,40.1529963693981)) ;
#15109=CARTESIAN_POINT('Ctrl Pts',(24.4900246898011,38.932546549643,41.6721498544424)) ;
#15110=CARTESIAN_POINT('Ctrl Pts',(24.3792098748909,40.9578961867131,41.3430908176903)) ;
#15111=CARTESIAN_POINT('Ctrl Pts',(24.2683950599807,41.7853206509447,39.4654088004043)) ;
#15112=CARTESIAN_POINT('Ctrl Pts',(24.1575802450707,40.6614970185386,37.7486265063164)) ;
#15113=CARTESIAN_POINT('Ctrl Pts',(24.0467654301604,38.6096028013962,37.755776590631)) ;
#15114=CARTESIAN_POINT('Ctrl Pts',(23.9359506152504,37.49777100477,39.480349308164)) ;
#15115=CARTESIAN_POINT('Ctrl Pts',(23.8251358003402,38.3382612559907,41.3522192661607)) ;
#15116=CARTESIAN_POINT('Ctrl Pts',(23.7143209854301,40.3658549751821,41.6671553103742)) ;
#15117=CARTESIAN_POINT('Ctrl Pts',(23.6035061705199,41.7345433786454,40.1384260811533)) ;
#15118=CARTESIAN_POINT('Ctrl Pts',(23.4926913556098,41.1982135044883,38.157852611643)) ;
#15119=CARTESIAN_POINT('Ctrl Pts',(23.3818765406997,39.2451632051238,37.5286344219733)) ;
#15120=CARTESIAN_POINT('Ctrl Pts',(23.2710617257895,37.6535337193609,38.8236388938198)) ;
#15121=CARTESIAN_POINT('Ctrl Pts',(23.1602469108794,37.8724131871331,40.8638380950209)) ;
#15122=CARTESIAN_POINT('Ctrl Pts',(23.0494320959692,39.702524299481,41.791746667355)) ;
#15123=CARTESIAN_POINT('Ctrl Pts',(22.9386172810591,41.4776549564797,40.7625566204605)) ;
#15124=CARTESIAN_POINT('Ctrl Pts',(22.8278024661489,41.5816496365404,38.7132869680797)) ;
#15125=CARTESIAN_POINT('Ctrl Pts',(22.7169876512388,39.9198270968306,37.5096811981338)) ;
#15126=CARTESIAN_POINT('Ctrl Pts',(22.6061728363287,38.0051822618756,38.2475539227206)) ;
#15127=CARTESIAN_POINT('Ctrl Pts',(22.4953580214185,37.58089037816,40.2551139832574)) ;
#15128=CARTESIAN_POINT('Ctrl Pts',(22.3845432065084,39.0332450805022,41.7045921059208)) ;
#15129=CARTESIAN_POINT('Ctrl Pts',(22.2737283915983,41.039959996023,41.2763208778023)) ;
#15130=CARTESIAN_POINT('Ctrl Pts',(22.1629135766881,41.7740353114579,39.3602169102235)) ;
#15131=CARTESIAN_POINT('Ctrl Pts',(22.052098761778,40.5671371808738,37.7007838849531)) ;
#15132=CARTESIAN_POINT('Ctrl Pts',(21.9412839468678,38.5180777505257,37.8088412547445)) ;
#15133=CARTESIAN_POINT('Ctrl Pts',(21.8304691319577,37.4924090580876,39.5860088377472)) ;
#15134=CARTESIAN_POINT('Ctrl Pts',(21.7196543170475,38.4239442347988,41.414276789266)) ;
#15135=CARTESIAN_POINT('Ctrl Pts',(21.6088395021374,40.4645732522469,41.6291107383832)) ;
#15136=CARTESIAN_POINT('Ctrl Pts',(21.4980246872273,41.7564198705513,40.0349173182877)) ;
#15137=CARTESIAN_POINT('Ctrl Pts',(21.3872098723171,41.1233303214206,38.0831175320853)) ;
#15138=CARTESIAN_POINT('Ctrl Pts',(21.276395057407,39.1416984015515,37.5507170005344)) ;
#15139=CARTESIAN_POINT('Ctrl Pts',(21.1655802424968,37.6156837693313,38.9224303337358)) ;
#15140=CARTESIAN_POINT('Ctrl Pts',(21.0547654275867,37.934643004614,40.9494021282203)) ;
#15141=CARTESIAN_POINT('Ctrl Pts',(20.9439506126766,39.8081678118156,41.786166684821)) ;
#15142=CARTESIAN_POINT('Ctrl Pts',(20.8331357977664,41.5305484559254,40.6709436872534)) ;
#15143=CARTESIAN_POINT('Ctrl Pts',(20.7223209828563,41.5335992379307,38.6189879065129)) ;
#15144=CARTESIAN_POINT('Ctrl Pts',(20.6115061679461,39.8146545909814,37.4986728844175)) ;
#15145=CARTESIAN_POINT('Ctrl Pts',(20.500691353036,37.9384921399142,38.3296131999977)) ;
#15146=CARTESIAN_POINT('Ctrl Pts',(20.3898765381259,37.6136980486187,40.356021230108)) ;
#15147=CARTESIAN_POINT('Ctrl Pts',(20.2790617232157,39.1350859482812,41.7314959838511)) ;
#15148=CARTESIAN_POINT('Ctrl Pts',(20.1682469083056,41.1193035966469,41.2066976185349)) ;
#15149=CARTESIAN_POINT('Ctrl Pts',(20.0574320933954,41.756248612587,39.2533866691575)) ;
#15150=CARTESIAN_POINT('Ctrl Pts',(19.983555550122,40.9009085056161,38.1941237260219)) ;
#15151=CARTESIAN_POINT('Ctrl Pts',(19.9466172784853,40.3436880472122,37.9615190032951)) ;
#15152=CARTESIAN_POINT('Ctrl Pts',(29.4,37.8883143121033,40.5036614834013)) ;
#15153=CARTESIAN_POINT('Ctrl Pts',(29.3630617283633,38.1739593715505,41.0851534806482)) ;
#15154=CARTESIAN_POINT('Ctrl Pts',(29.2891851850899,39.3644496496292,41.9317014755988)) ;
#15155=CARTESIAN_POINT('Ctrl Pts',(29.1783703701797,41.4145450175032,41.1214832212394)) ;
#15156=CARTESIAN_POINT('Ctrl Pts',(29.0675555552696,41.8464489493472,38.9621047721517)) ;
#15157=CARTESIAN_POINT('Ctrl Pts',(28.9567407403594,40.2736394367121,37.4230007636482)) ;
#15158=CARTESIAN_POINT('Ctrl Pts',(28.8459259254493,38.1247919756811,37.9037199030322)) ;
#15159=CARTESIAN_POINT('Ctrl Pts',(28.7351111105392,37.3579446442441,39.9674544957336)) ;
#15160=CARTESIAN_POINT('Ctrl Pts',(28.624296295629,38.6704505124476,41.7348611900198)) ;
#15161=CARTESIAN_POINT('Ctrl Pts',(28.5134814807189,40.8677569780034,41.5970321243973)) ;
#15162=CARTESIAN_POINT('Ctrl Pts',(28.4026666658087,41.9491365352617,39.6793449827905)) ;
#15163=CARTESIAN_POINT('Ctrl Pts',(28.2918518508986,40.9301571684799,37.7277988448269)) ;
#15164=CARTESIAN_POINT('Ctrl Pts',(28.1810370359885,38.7384902973957,37.5191384714753)) ;
#15165=CARTESIAN_POINT('Ctrl Pts',(28.0702222210783,37.369549686032,39.2433507955181)) ;
#15166=CARTESIAN_POINT('Ctrl Pts',(27.9594074061682,38.0696650493416,41.330631769909)) ;
#15167=CARTESIAN_POINT('Ctrl Pts',(27.8485925912581,40.2014276021217,41.8806341491974)) ;
#15168=CARTESIAN_POINT('Ctrl Pts',(27.7377777763479,41.8239855365992,40.3926103455026)) ;
#15169=CARTESIAN_POINT('Ctrl Pts',(27.6269629614378,41.4600937331885,38.2213222662214)) ;
#15170=CARTESIAN_POINT('Ctrl Pts',(27.5161481465276,39.4410541784057,37.3436038135818)) ;
#15171=CARTESIAN_POINT('Ctrl Pts',(27.4053333316175,37.6050879801832,38.5585679407779)) ;
#15172=CARTESIAN_POINT('Ctrl Pts',(27.2945185167073,37.623737758645,40.7600587914735)) ;
#15173=CARTESIAN_POINT('Ctrl Pts',(27.1837037017972,39.4800240523721,41.9437441856142)) ;
#15174=CARTESIAN_POINT('Ctrl Pts',(27.072888886887,41.4839036965388,41.0319458545299)) ;
#15175=CARTESIAN_POINT('Ctrl Pts',(26.9620740719769,41.8109582496746,38.8548043432993)) ;
#15176=CARTESIAN_POINT('Ctrl Pts',(26.8512592570668,40.1634231261504,37.3944831896552)) ;
#15177=CARTESIAN_POINT('Ctrl Pts',(26.7404444421566,38.0412853764272,37.9805217672518)) ;
#15178=CARTESIAN_POINT('Ctrl Pts',(26.6296296272465,37.3766307446391,40.0793652741634)) ;
#15179=CARTESIAN_POINT('Ctrl Pts',(26.5188148123364,38.7745894795274,41.7801360473788)) ;
#15180=CARTESIAN_POINT('Ctrl Pts',(26.4079999974262,40.9623996460732,41.5343790105443)) ;
#15181=CARTESIAN_POINT('Ctrl Pts',(26.2971851825161,41.9481844962523,39.565841971115)) ;
#15182=CARTESIAN_POINT('Ctrl Pts',(26.1863703676059,40.8344429797072,37.666765963975)) ;
#15183=CARTESIAN_POINT('Ctrl Pts',(26.0755555526958,38.63517341526,37.5661517041173)) ;
#15184=CARTESIAN_POINT('Ctrl Pts',(25.9647407377857,37.3526856814434,39.3556027537603)) ;
#15185=CARTESIAN_POINT('Ctrl Pts',(25.8539259228755,38.1546119322008,41.405925688035)) ;
#15186=CARTESIAN_POINT('Ctrl Pts',(25.7431111079654,40.3108439171514,41.8504180653835)) ;
#15187=CARTESIAN_POINT('Ctrl Pts',(25.6322962930553,41.8582550265502,40.2843948519655)) ;
#15188=CARTESIAN_POINT('Ctrl Pts',(25.5214814781451,41.3880154376809,38.133631132838)) ;
#15189=CARTESIAN_POINT('Ctrl Pts',(25.410666663235,39.3282515563825,37.3562749726704)) ;
#15190=CARTESIAN_POINT('Ctrl Pts',(25.2998518483248,37.5542612696178,38.6600649515084)) ;
#15191=CARTESIAN_POINT('Ctrl Pts',(25.1890370334147,37.6811618568337,40.8579744326787)) ;
#15192=CARTESIAN_POINT('Ctrl Pts',(25.0782222185045,39.5934175494783,41.9489318160816)) ;
#15193=CARTESIAN_POINT('Ctrl Pts',(24.9674074035944,41.5500282784125,40.9396824406184)) ;
#15194=CARTESIAN_POINT('Ctrl Pts',(24.8565925886842,41.7696112361718,38.7490904724245)) ;
#15195=CARTESIAN_POINT('Ctrl Pts',(24.7457777737741,40.0522486261398,37.3715653321395)) ;
#15196=CARTESIAN_POINT('Ctrl Pts',(24.634962958864,37.9615014481887,38.0612653280387)) ;
#15197=CARTESIAN_POINT('Ctrl Pts',(24.5241481439539,37.4008761190426,40.190257833139)) ;
#15198=CARTESIAN_POINT('Ctrl Pts',(24.4133333290437,38.8807901213416,41.8202162351395)) ;
#15199=CARTESIAN_POINT('Ctrl Pts',(24.3025185141336,41.0538659102142,41.4671560954048)) ;
#15200=CARTESIAN_POINT('Ctrl Pts',(24.1917036992234,41.9416415502482,39.4525185946579)) ;
#15201=CARTESIAN_POINT('Ctrl Pts',(24.0808888843133,40.7358478039017,37.6105166164492)) ;
#15202=CARTESIAN_POINT('Ctrl Pts',(23.9700740694031,38.5342913106484,37.6181882178497)) ;
#15203=CARTESIAN_POINT('Ctrl Pts',(23.859259254493,37.3413640677048,39.4685488420246)) ;
#15204=CARTESIAN_POINT('Ctrl Pts',(23.7484444395828,38.2431584948403,41.4769503600581)) ;
#15205=CARTESIAN_POINT('Ctrl Pts',(23.6376296246727,40.4186420460256,41.8148573960569)) ;
#15206=CARTESIAN_POINT('Ctrl Pts',(23.5268148097626,41.8871606551775,40.1746248085776)) ;
#15207=CARTESIAN_POINT('Ctrl Pts',(23.4159999948524,41.311711634896,38.0495910979033)) ;
#15208=CARTESIAN_POINT('Ctrl Pts',(23.3051851799423,39.2162085956582,37.3744786191179)) ;
#15209=CARTESIAN_POINT('Ctrl Pts',(23.1943703650321,37.5084878954584,38.7639388943928)) ;
#15210=CARTESIAN_POINT('Ctrl Pts',(23.083555550122,37.743332123532,40.9529473537028)) ;
#15211=CARTESIAN_POINT('Ctrl Pts',(22.9727407352119,39.7069289644918,41.9485362712508)) ;
#15212=CARTESIAN_POINT('Ctrl Pts',(22.8619259203017,41.6115351530753,40.844278550944)) ;
#15213=CARTESIAN_POINT('Ctrl Pts',(22.7511111053916,41.7231150587249,38.645538054512)) ;
#15214=CARTESIAN_POINT('Ctrl Pts',(22.6402962904815,39.9400815220214,37.3541429738087)) ;
#15215=CARTESIAN_POINT('Ctrl Pts',(22.5294814755713,37.8857851877109,38.1458350963543)) ;
#15216=CARTESIAN_POINT('Ctrl Pts',(22.4186666606612,37.4305460511974,40.2998237620203)) ;
#15217=CARTESIAN_POINT('Ctrl Pts',(22.307851845751,38.9888334613064,41.8550247787775)) ;
#15218=CARTESIAN_POINT('Ctrl Pts',(22.1970370308409,41.1419153382684,41.3955160500816)) ;
#15219=CARTESIAN_POINT('Ctrl Pts',(22.0862222159308,41.9295330739837,39.3396541560672)) ;
#15220=CARTESIAN_POINT('Ctrl Pts',(21.9754074010206,40.6346054924911,37.5591844216232)) ;
#15221=CARTESIAN_POINT('Ctrl Pts',(21.8645925861105,38.4360905513911,37.675123343874)) ;
#15222=CARTESIAN_POINT('Ctrl Pts',(21.7537777712003,37.3356110281783,39.5819150289772)) ;
#15223=CARTESIAN_POINT('Ctrl Pts',(21.6429629562902,38.3350910695221,41.5435342715513)) ;
#15224=CARTESIAN_POINT('Ctrl Pts',(21.53214814138,40.5245606952712,41.7740379065334)) ;
#15225=CARTESIAN_POINT('Ctrl Pts',(21.4213333264699,41.9106327876115,40.0635662622395)) ;
#15226=CARTESIAN_POINT('Ctrl Pts',(21.3105185115598,41.2313665778549,37.9694049468339)) ;
#15227=CARTESIAN_POINT('Ctrl Pts',(21.1997036966496,39.1051972149425,37.3981718698776)) ;
#15228=CARTESIAN_POINT('Ctrl Pts',(21.0888888817395,37.4678772233483,38.869936042885)) ;
#15229=CARTESIAN_POINT('Ctrl Pts',(20.9780740668294,37.8101008963102,41.0447523070506)) ;
#15230=CARTESIAN_POINT('Ctrl Pts',(20.8672592519192,39.8202779659203,41.9425492926447)) ;
#15231=CARTESIAN_POINT('Ctrl Pts',(20.7564444370091,41.6682866299218,40.7459834993361)) ;
#15232=CARTESIAN_POINT('Ctrl Pts',(20.6456296220989,41.6715599316725,38.5443609521226)) ;
#15233=CARTESIAN_POINT('Ctrl Pts',(20.5348148071888,39.8272378816283,37.3423317291844)) ;
#15234=CARTESIAN_POINT('Ctrl Pts',(20.4239999922786,37.8142307821214,38.2338796618157)) ;
#15235=CARTESIAN_POINT('Ctrl Pts',(20.3131851773685,37.4657466669618,40.4080910414269)) ;
#15236=CARTESIAN_POINT('Ctrl Pts',(20.2023703624584,39.0981024586378,41.8838909876963)) ;
#15237=CARTESIAN_POINT('Ctrl Pts',(20.0915555475482,41.227046149444,41.3208145682793)) ;
#15238=CARTESIAN_POINT('Ctrl Pts',(19.9807407326381,41.9104490383323,39.2250318675839)) ;
#15239=CARTESIAN_POINT('Ctrl Pts',(19.9068641893647,40.9927216278695,38.0885077763125)) ;
#15240=CARTESIAN_POINT('Ctrl Pts',(19.8699259177279,40.39485829353,37.8389371925064)) ;
#15241=CARTESIAN_POINT('Ctrl Pts',(20.1758696921242,39.6403856614379,41.5960667040991)) ;
#15242=CARTESIAN_POINT('Ctrl Pts',(20.1505797947495,40.0840112824575,41.5922443072459)) ;
#15243=CARTESIAN_POINT('Ctrl Pts',(20.1252898973747,40.5301478361562,41.4385916227714)) ;
#15244=CARTESIAN_POINT('Ctrl Pts',(20.1,40.8749138146614,41.1621829179884)) ;
#15245=CARTESIAN_POINT('',(29.4,40.9082616204537,40.5457424023813)) ;
#15246=CARTESIAN_POINT('Ctrl Pts',(29.4,40.9099017087087,40.5477081290461)) ;
#15247=CARTESIAN_POINT('Ctrl Pts',(29.4,40.8911935153115,40.5827280609995)) ;
#15248=CARTESIAN_POINT('Ctrl Pts',(29.4,40.8710967810982,40.6169137862787)) ;
#15249=CARTESIAN_POINT('Ctrl Pts',(29.4,40.849630844981,40.650172378807)) ;
#15250=CARTESIAN_POINT('Ctrl Pts',(29.4,40.8174332982874,40.7000581643625)) ;
#15251=CARTESIAN_POINT('Ctrl Pts',(29.4,40.7821579182634,40.7478593980477)) ;
#15252=CARTESIAN_POINT('Ctrl Pts',(29.4,40.7441238056603,40.7934984035053)) ;
#15253=CARTESIAN_POINT('Ctrl Pts',(29.4,40.720671405954,40.8216400932919)) ;
#15254=CARTESIAN_POINT('Ctrl Pts',(29.4,40.6961690606009,40.8489593935245)) ;
#15255=CARTESIAN_POINT('Ctrl Pts',(29.4,40.6706828011567,40.875434378279)) ;
#15256=CARTESIAN_POINT('Ctrl Pts',(29.4,40.6617631345853,40.8847000783717)) ;
#15257=CARTESIAN_POINT('Ctrl Pts',(29.4,40.6527245408652,40.89386049634)) ;
#15258=CARTESIAN_POINT('Ctrl Pts',(29.4,40.6435778736667,40.902907120743)) ;
#15259=CARTESIAN_POINT('Ctrl Pts',(29.4,40.5992766463879,40.9467237979089)) ;
#15260=CARTESIAN_POINT('Ctrl Pts',(29.4,40.5523942995144,40.9879249952783)) ;
#15261=CARTESIAN_POINT('Ctrl Pts',(29.4,40.5032793806035,41.0264241184463)) ;
#15262=CARTESIAN_POINT('Ctrl Pts',(29.4,40.465416175545,41.0561034954543)) ;
#15263=CARTESIAN_POINT('Ctrl Pts',(29.4,40.4262249186537,41.0841767525349)) ;
#15264=CARTESIAN_POINT('Ctrl Pts',(29.4,40.3858469011584,41.1105939537831)) ;
#15265=CARTESIAN_POINT('Ctrl Pts',(29.4,40.3698454319037,41.1210628687965)) ;
#15266=CARTESIAN_POINT('Ctrl Pts',(29.4,40.3536574290092,41.131271591281)) ;
#15267=CARTESIAN_POINT('Ctrl Pts',(29.4,40.3372911151227,41.1412165309672)) ;
#15268=CARTESIAN_POINT('Ctrl Pts',(29.4,40.3267725201988,41.1476081224291)) ;
#15269=CARTESIAN_POINT('Ctrl Pts',(29.4,40.3161801620067,41.1538906909963)) ;
#15270=CARTESIAN_POINT('Ctrl Pts',(29.4,40.3055290468822,41.1600561153331)) ;
#15271=CARTESIAN_POINT('Ctrl Pts',(29.4,40.2495545026299,41.1924571187342)) ;
#15272=CARTESIAN_POINT('Ctrl Pts',(29.4,40.1918758690529,41.2216774859145)) ;
#15273=CARTESIAN_POINT('Ctrl Pts',(29.4,40.1328473057965,41.2476277355336)) ;
#15274=CARTESIAN_POINT('Ctrl Pts',(29.4,40.0725752515564,41.2741246510318)) ;
#15275=CARTESIAN_POINT('Ctrl Pts',(29.4,40.0108950153682,41.2972129741303)) ;
#15276=CARTESIAN_POINT('Ctrl Pts',(29.4,39.9481419144707,41.3167635433489)) ;
#15277=CARTESIAN_POINT('Ctrl Pts',(29.4,39.9063144539236,41.3297947824584)) ;
#15278=CARTESIAN_POINT('Ctrl Pts',(29.4,39.8640094931252,41.3412535685766)) ;
#15279=CARTESIAN_POINT('Ctrl Pts',(29.4,39.8213191168389,41.3510910041002)) ;
#15280=CARTESIAN_POINT('Ctrl Pts',(29.4,39.8000975814559,41.3559812277103)) ;
#15281=CARTESIAN_POINT('Ctrl Pts',(29.4,39.7787807324178,41.3604706528433)) ;
#15282=CARTESIAN_POINT('Ctrl Pts',(29.4,39.7573795302911,41.3645523656715)) ;
#15283=CARTESIAN_POINT('Ctrl Pts',(29.4,39.742623604249,41.3673666679832)) ;
#15284=CARTESIAN_POINT('Ctrl Pts',(29.4,39.7278275724937,41.3699871322496)) ;
#15285=CARTESIAN_POINT('Ctrl Pts',(29.4,39.7129949834893,41.3724113112808)) ;
#15286=CARTESIAN_POINT('Ctrl Pts',(29.4,39.7024878196002,41.3741285601285)) ;
#15287=CARTESIAN_POINT('Ctrl Pts',(29.4,39.6919717860519,41.3757457576257)) ;
#15288=CARTESIAN_POINT('Ctrl Pts',(29.4,39.6814484822052,41.3772624926511)) ;
#15289=CARTESIAN_POINT('Ctrl Pts',(29.4,39.6144049308324,41.3869255513325)) ;
#15290=CARTESIAN_POINT('Ctrl Pts',(29.4,39.5470667639266,41.3925146504903)) ;
#15291=CARTESIAN_POINT('Ctrl Pts',(29.4,39.4797876237661,41.39390686565)) ;
#15292=CARTESIAN_POINT('Ctrl Pts',(29.4,39.4636730092403,41.3942403272635)) ;
#15293=CARTESIAN_POINT('Ctrl Pts',(29.4,39.4475616490742,41.3943328224262)) ;
#15294=CARTESIAN_POINT('Ctrl Pts',(29.4,39.4314581800028,41.3941822776708)) ;
#15295=CARTESIAN_POINT('Ctrl Pts',(29.4,39.3665783523775,41.3935757426604)) ;
#15296=CARTESIAN_POINT('Ctrl Pts',(29.4,39.3018273724191,41.3890282454472)) ;
#15297=CARTESIAN_POINT('Ctrl Pts',(29.4,39.2374411018851,41.3807559085843)) ;
#15298=CARTESIAN_POINT('Ctrl Pts',(29.4,39.2024146503065,41.3762557161649)) ;
#15299=CARTESIAN_POINT('Ctrl Pts',(29.4,39.1674959422765,41.3706522775741)) ;
#15300=CARTESIAN_POINT('Ctrl Pts',(29.4,39.1327223454014,41.3639741186901)) ;
#15301=CARTESIAN_POINT('Ctrl Pts',(29.4,39.1026495332469,41.358198730588)) ;
#15302=CARTESIAN_POINT('Ctrl Pts',(29.4,39.0726852321098,41.351619475739)) ;
#15303=CARTESIAN_POINT('Ctrl Pts',(29.4,39.0428537605999,41.3442522807742)) ;
#15304=CARTESIAN_POINT('Ctrl Pts',(29.4,39.0327852838907,41.3417657647841)) ;
#15305=CARTESIAN_POINT('Ctrl Pts',(29.4,39.0227348244623,41.339190133892)) ;
#15306=CARTESIAN_POINT('Ctrl Pts',(29.4,39.0127114014828,41.3365283979405)) ;
#15307=CARTESIAN_POINT('Ctrl Pts',(29.4,38.9471470175288,41.3191176712587)) ;
#15308=CARTESIAN_POINT('Ctrl Pts',(29.4,38.8826389394181,41.2980024905982)) ;
#15309=CARTESIAN_POINT('Ctrl Pts',(29.4,38.8194432421882,41.2734401520375)) ;
#15310=CARTESIAN_POINT('Ctrl Pts',(29.4,38.7549205183317,41.2483620366326)) ;
#15311=CARTESIAN_POINT('Ctrl Pts',(29.4,38.6917649898121,41.2196903008299)) ;
#15312=CARTESIAN_POINT('Ctrl Pts',(29.4,38.6302461565059,41.1876436249062)) ;
#15313=CARTESIAN_POINT('Ctrl Pts',(29.4,38.5682684460675,41.155357908579)) ;
#15314=CARTESIAN_POINT('Ctrl Pts',(29.4,38.5079509547186,41.1196463915286)) ;
#15315=CARTESIAN_POINT('Ctrl Pts',(29.4,38.4495803765141,41.0806812192905)) ;
#15316=CARTESIAN_POINT('Ctrl Pts',(29.4,38.4345977593732,41.0706796007452)) ;
#15317=CARTESIAN_POINT('Ctrl Pts',(29.4,38.4197435148233,41.0604633668381)) ;
#15318=CARTESIAN_POINT('Ctrl Pts',(29.4,38.4050227327501,41.0500349287453)) ;
#15319=CARTESIAN_POINT('Ctrl Pts',(29.4,38.395076102545,41.0429885763974)) ;
#15320=CARTESIAN_POINT('Ctrl Pts',(29.4,38.3851898915416,41.035844847252)) ;
#15321=CARTESIAN_POINT('Ctrl Pts',(29.4,38.3753786911808,41.0286143383668)) ;
#15322=CARTESIAN_POINT('Ctrl Pts',(29.4,38.3172621602953,40.985784503332)) ;
#15323=CARTESIAN_POINT('Ctrl Pts',(29.4,38.2616662256681,40.9398368489584)) ;
#15324=CARTESIAN_POINT('Ctrl Pts',(29.4,38.2088717556074,40.8910128665259)) ;
#15325=CARTESIAN_POINT('Ctrl Pts',(29.4,38.1559526948364,40.8420736634151)) ;
#15326=CARTESIAN_POINT('Ctrl Pts',(29.4,38.1058473267557,40.7902441084932)) ;
#15327=CARTESIAN_POINT('Ctrl Pts',(29.4,38.0588546893559,40.7357177820414)) ;
#15328=CARTESIAN_POINT('Ctrl Pts',(29.4,38.0128654690254,40.6823557368411)) ;
#15329=CARTESIAN_POINT('Ctrl Pts',(29.4,37.9698566114721,40.6264102871568)) ;
#15330=CARTESIAN_POINT('Ctrl Pts',(29.4,37.9301375288794,40.5680230943791)) ;
#15331=CARTESIAN_POINT('Ctrl Pts',(29.4,37.9157597103701,40.5468876499976)) ;
#15332=CARTESIAN_POINT('Ctrl Pts',(29.4,37.9018133110483,40.5254319089879)) ;
#15333=CARTESIAN_POINT('Ctrl Pts',(29.4,37.8883143121033,40.5036614834013)) ;
#15334=CARTESIAN_POINT('Ctrl Pts',(29.4,40.9099017087087,40.5477081290461)) ;
#15335=CARTESIAN_POINT('Ctrl Pts',(29.3658765458472,41.1836081239267,40.1599355816674)) ;
#15336=CARTESIAN_POINT('Ctrl Pts',(29.2948148200577,41.3650964581925,39.0696688144179)) ;
#15337=CARTESIAN_POINT('Ctrl Pts',(29.1868148226315,40.1448501483431,37.8755725352669)) ;
#15338=CARTESIAN_POINT('Ctrl Pts',(29.0760000077214,38.4342400021641,38.2582535083027)) ;
#15339=CARTESIAN_POINT('Ctrl Pts',(28.9651851928112,37.8237840021384,39.9011087585314)) ;
#15340=CARTESIAN_POINT('Ctrl Pts',(28.8751664483696,38.6725380053612,41.044032034868)) ;
#15341=CARTESIAN_POINT('Ctrl Pts',(28.8220859755646,39.4154275518878,41.1959818279421)) ;
#15342=CARTESIAN_POINT('Ctrl Pts',(28.8059437743963,39.6416116368869,41.195305032435)) ;
#15343=CARTESIAN_POINT('Origin',(29.4,39.642135623731,39.642135623731)) ;
#15344=CARTESIAN_POINT('',(29.4,39.642135623731,41.596135623731)) ;
#15345=CARTESIAN_POINT('Origin',(29.4,39.642135623731,39.642135623731)) ;
#15346=CARTESIAN_POINT('',(29.4,40.9082616204539,38.7385288450808)) ;
#15347=CARTESIAN_POINT('Ctrl Pts',(29.4,37.8858801137886,38.7785081419809)) ;
#15348=CARTESIAN_POINT('Ctrl Pts',(29.4,37.9116490910512,38.7365164424919)) ;
#15349=CARTESIAN_POINT('Ctrl Pts',(29.4,37.9390708494547,38.6956362623256)) ;
#15350=CARTESIAN_POINT('Ctrl Pts',(29.4,37.9681504858012,38.6559804743706)) ;
#15351=CARTESIAN_POINT('Ctrl Pts',(29.4,38.0106510442209,38.5980226267355)) ;
#15352=CARTESIAN_POINT('Ctrl Pts',(29.4,38.0566920308732,38.5426781003507)) ;
#15353=CARTESIAN_POINT('Ctrl Pts',(29.4,38.1059332588112,38.490108579696)) ;
#15354=CARTESIAN_POINT('Ctrl Pts',(29.4,38.1306294723998,38.4637431098508)) ;
#15355=CARTESIAN_POINT('Ctrl Pts',(29.4,38.1561311460157,38.4380763320497)) ;
#15356=CARTESIAN_POINT('Ctrl Pts',(29.4,38.1823975605347,38.4131329663715)) ;
#15357=CARTESIAN_POINT('Ctrl Pts',(29.4,38.1930192567399,38.4030462888625)) ;
#15358=CARTESIAN_POINT('Ctrl Pts',(29.4,38.2037677831062,38.3930763509752)) ;
#15359=CARTESIAN_POINT('Ctrl Pts',(29.4,38.2146347705142,38.3832300940798)) ;
#15360=CARTESIAN_POINT('Ctrl Pts',(29.4,38.2675074522367,38.335323716034)) ;
#15361=CARTESIAN_POINT('Ctrl Pts',(29.4,38.3230763648864,38.2904355096495)) ;
#15362=CARTESIAN_POINT('Ctrl Pts',(29.4,38.3810032036924,38.2487185952537)) ;
#15363=CARTESIAN_POINT('Ctrl Pts',(29.4,38.4238104588198,38.2178902843278)) ;
#15364=CARTESIAN_POINT('Ctrl Pts',(29.4,38.4679061537415,38.1887947021649)) ;
#15365=CARTESIAN_POINT('Ctrl Pts',(29.4,38.5131601184473,38.1615107790893)) ;
#15366=CARTESIAN_POINT('Ctrl Pts',(29.4,38.5369340087092,38.1471773389735)) ;
#15367=CARTESIAN_POINT('Ctrl Pts',(29.4,38.561027626749,38.1333441438862)) ;
#15368=CARTESIAN_POINT('Ctrl Pts',(29.4,38.5854223149118,38.1200243793908)) ;
#15369=CARTESIAN_POINT('Ctrl Pts',(29.4,38.5965922808676,38.11392545675)) ;
#15370=CARTESIAN_POINT('Ctrl Pts',(29.4,38.6078253694791,38.1079341964166)) ;
#15371=CARTESIAN_POINT('Ctrl Pts',(29.4,38.6191197890281,38.102051951947)) ;
#15372=CARTESIAN_POINT('Ctrl Pts',(29.4,38.6299426725146,38.0964152880833)) ;
#15373=CARTESIAN_POINT('Ctrl Pts',(29.4,38.640812808894,38.0908834475283)) ;
#15374=CARTESIAN_POINT('Ctrl Pts',(29.4,38.6517284773785,38.0854570976242)) ;
#15375=CARTESIAN_POINT('Ctrl Pts',(29.4,38.7140552839742,38.054473465108)) ;
#15376=CARTESIAN_POINT('Ctrl Pts',(29.4,38.7778654686989,38.0269249898323)) ;
#15377=CARTESIAN_POINT('Ctrl Pts',(29.4,38.8428505039851,38.002963908533)) ;
#15378=CARTESIAN_POINT('Ctrl Pts',(29.4,38.9062492642292,37.979587713663)) ;
#15379=CARTESIAN_POINT('Ctrl Pts',(29.4,38.9707671925793,37.9596258261471)) ;
#15380=CARTESIAN_POINT('Ctrl Pts',(29.4,39.0361228154364,37.9432679613406)) ;
#15381=CARTESIAN_POINT('Ctrl Pts',(29.4,39.079431002153,37.9324283513369)) ;
#15382=CARTESIAN_POINT('Ctrl Pts',(29.4,39.1231071037785,37.9231722948001)) ;
#15383=CARTESIAN_POINT('Ctrl Pts',(29.4,39.1670674387888,37.9155674593897)) ;
#15384=CARTESIAN_POINT('Ctrl Pts',(29.4,39.2048397834777,37.9090331037176)) ;
#15385=CARTESIAN_POINT('Ctrl Pts',(29.4,39.2428219878473,37.9037179738841)) ;
#15386=CARTESIAN_POINT('Ctrl Pts',(29.4,39.280959018589,37.8996711971933)) ;
#15387=CARTESIAN_POINT('Ctrl Pts',(29.4,39.2919799253728,37.8985017524878)) ;
#15388=CARTESIAN_POINT('Ctrl Pts',(29.4,39.3030111173088,37.8974386139797)) ;
#15389=CARTESIAN_POINT('Ctrl Pts',(29.4,39.3140406985631,37.8964836104455)) ;
#15390=CARTESIAN_POINT('Ctrl Pts',(29.4,39.3789502991843,37.89086337006)) ;
#15391=CARTESIAN_POINT('Ctrl Pts',(29.4,39.4439095597764,37.8889726547203)) ;
#15392=CARTESIAN_POINT('Ctrl Pts',(29.4,39.5086578198928,37.8909777261666)) ;
#15393=CARTESIAN_POINT('Ctrl Pts',(29.4,39.5277630833133,37.891569362422)) ;
#15394=CARTESIAN_POINT('Ctrl Pts',(29.4,39.5468499309991,37.8925005294073)) ;
#15395=CARTESIAN_POINT('Ctrl Pts',(29.4,39.5659115036032,37.8937763630377)) ;
#15396=CARTESIAN_POINT('Ctrl Pts',(29.4,39.6351147135408,37.8984082884514)) ;
#15397=CARTESIAN_POINT('Ctrl Pts',(29.4,39.7039870331875,37.9075788728914)) ;
#15398=CARTESIAN_POINT('Ctrl Pts',(29.4,39.7721797673507,37.9210906044853)) ;
#15399=CARTESIAN_POINT('Ctrl Pts',(29.4,39.8033157439461,37.9272598975022)) ;
#15400=CARTESIAN_POINT('Ctrl Pts',(29.4,39.8343096425566,37.93433496609)) ;
#15401=CARTESIAN_POINT('Ctrl Pts',(29.4,39.8651257692214,37.9423005035321)) ;
#15402=CARTESIAN_POINT('Ctrl Pts',(29.4,39.8932532269645,37.9495710576884)) ;
#15403=CARTESIAN_POINT('Ctrl Pts',(29.4,39.9212325733677,37.9575835088157)) ;
#15404=CARTESIAN_POINT('Ctrl Pts',(29.4,39.9490351922892,37.9663275513776)) ;
#15405=CARTESIAN_POINT('Ctrl Pts',(29.4,39.9595483179186,37.9696339743525)) ;
#15406=CARTESIAN_POINT('Ctrl Pts',(29.4,39.9700278224812,37.9730424119132)) ;
#15407=CARTESIAN_POINT('Ctrl Pts',(29.4,39.980469829338,37.9765509966401)) ;
#15408=CARTESIAN_POINT('Ctrl Pts',(29.4,40.0419133031625,37.997196418232)) ;
#15409=CARTESIAN_POINT('Ctrl Pts',(29.4,40.1020897414224,38.021314799644)) ;
#15410=CARTESIAN_POINT('Ctrl Pts',(29.4,40.1607244120033,38.0487200327042)) ;
#15411=CARTESIAN_POINT('Ctrl Pts',(29.4,40.219108739998,38.0760082582524)) ;
#15412=CARTESIAN_POINT('Ctrl Pts',(29.4,40.2759652711504,38.1065560863141)) ;
#15413=CARTESIAN_POINT('Ctrl Pts',(29.4,40.3309901219769,38.1402191974643)) ;
#15414=CARTESIAN_POINT('Ctrl Pts',(29.4,40.3848769210849,38.1731860711705)) ;
#15415=CARTESIAN_POINT('Ctrl Pts',(29.4,40.437007641609,38.2091414431635)) ;
#15416=CARTESIAN_POINT('Ctrl Pts',(29.4,40.4870549707429,38.2479764423802)) ;
#15417=CARTESIAN_POINT('Ctrl Pts',(29.4,40.4957821815725,38.2547484566234)) ;
#15418=CARTESIAN_POINT('Ctrl Pts',(29.4,40.5044459225108,38.2616080859552)) ;
#15419=CARTESIAN_POINT('Ctrl Pts',(29.4,40.5130443028292,38.268554812991)) ;
#15420=CARTESIAN_POINT('Ctrl Pts',(29.4,40.5221789060073,38.2759347604356)) ;
#15421=CARTESIAN_POINT('Ctrl Pts',(29.4,40.5312329743323,38.2834075887112)) ;
#15422=CARTESIAN_POINT('Ctrl Pts',(29.4,40.5402004635945,38.2909686978449)) ;
#15423=CARTESIAN_POINT('Ctrl Pts',(29.4,40.5876132249798,38.3309456694014)) ;
#15424=CARTESIAN_POINT('Ctrl Pts',(29.4,40.63264805134,38.373419504188)) ;
#15425=CARTESIAN_POINT('Ctrl Pts',(29.4,40.6750367350389,38.4182522509551)) ;
#15426=CARTESIAN_POINT('Ctrl Pts',(29.4,40.7166551699106,38.4622703375909)) ;
#15427=CARTESIAN_POINT('Ctrl Pts',(29.4,40.7557232872012,38.5085630921309)) ;
#15428=CARTESIAN_POINT('Ctrl Pts',(29.4,40.7919431689768,38.5570230298163)) ;
#15429=CARTESIAN_POINT('Ctrl Pts',(29.4,40.8270103880344,38.6039407768387)) ;
#15430=CARTESIAN_POINT('Ctrl Pts',(29.4,40.8594080675513,38.6528905689044)) ;
#15431=CARTESIAN_POINT('Ctrl Pts',(29.4,40.8888183567986,38.703787175567)) ;
#15432=CARTESIAN_POINT('Ctrl Pts',(29.4,40.8954530221445,38.7152689379396)) ;
#15433=CARTESIAN_POINT('Ctrl Pts',(29.4,40.901935450219,38.7268498061172)) ;
#15434=CARTESIAN_POINT('Ctrl Pts',(29.4,40.9082616204538,38.7385288450808)) ;
#15435=CARTESIAN_POINT('Origin',(29.4,39.642135623731,39.642135623731)) ;
#15436=CARTESIAN_POINT('Origin',(29.4,39.642135623731,39.642135623731)) ;
#15437=CARTESIAN_POINT('Origin',(30.6940562256037,39.642135623731,39.642135623731)) ;
#15438=CARTESIAN_POINT('Ctrl Pts',(29.4,40.9082616204539,38.7385288450808)) ;
#15439=CARTESIAN_POINT('Ctrl Pts',(29.3630617283633,40.6086643314031,38.3187357169443)) ;
#15440=CARTESIAN_POINT('Ctrl Pts',(29.2891851850898,39.5640416497925,37.8078105578506)) ;
#15441=CARTESIAN_POINT('Ctrl Pts',(29.1783703701797,38.0585610812911,38.709446862677)) ;
#15442=CARTESIAN_POINT('Ctrl Pts',(29.0675555552696,37.9986782664391,40.4614642406582)) ;
#15443=CARTESIAN_POINT('Ctrl Pts',(28.9894508404109,39.0097624153104,41.1701268863298)) ;
#15444=CARTESIAN_POINT('Ctrl Pts',(28.948284397189,39.5822413804429,41.1997935373523)) ;
#15445=CARTESIAN_POINT('Ctrl Pts',(28.9440562256037,39.6410873345839,41.199362363652)) ;
#15446=CARTESIAN_POINT('Ctrl Pts',(29.6300740822721,41.2326275540406,38.5070358837873)) ;
#15447=CARTESIAN_POINT('Ctrl Pts',(29.5931358106354,40.8562771182931,37.9796969108663)) ;
#15448=CARTESIAN_POINT('Ctrl Pts',(29.5192592673619,39.5440349325862,37.3378789996678)) ;
#15449=CARTESIAN_POINT('Ctrl Pts',(29.4084444524518,37.6528687282456,38.4705034545895)) ;
#15450=CARTESIAN_POINT('Ctrl Pts',(29.2976296375417,37.5776446715302,40.6713661717707)) ;
#15451=CARTESIAN_POINT('Ctrl Pts',(29.1868148226315,39.3796763444381,41.9343990601139)) ;
#15452=CARTESIAN_POINT('Ctrl Pts',(29.0760000077213,41.4218307707905,41.1108446083453)) ;
#15453=CARTESIAN_POINT('Ctrl Pts',(28.9651851928113,41.8430894430381,38.9499197708456)) ;
#15454=CARTESIAN_POINT('Ctrl Pts',(28.8543703779011,40.2607974022739,37.4193154134393)) ;
#15455=CARTESIAN_POINT('Ctrl Pts',(28.743555562991,38.1151025245061,37.9124137447615)) ;
#15456=CARTESIAN_POINT('Ctrl Pts',(28.6327407480808,37.3597577725899,39.9803498740405)) ;
#15457=CARTESIAN_POINT('Ctrl Pts',(28.5219259331707,38.6823515624876,41.7403489526177)) ;
#15458=CARTESIAN_POINT('Ctrl Pts',(28.4111111182605,40.8787925380227,41.5900502200798)) ;
#15459=CARTESIAN_POINT('Ctrl Pts',(28.3002963033504,41.949318515855,39.6662829548393)) ;
#15460=CARTESIAN_POINT('Ctrl Pts',(28.1894814884402,40.9192902716771,37.7205324493354)) ;
#15461=CARTESIAN_POINT('Ctrl Pts',(28.0786666735301,38.7264830396968,37.5242915968402)) ;
#15462=CARTESIAN_POINT('Ctrl Pts',(27.96785185862,37.3673265716251,39.2562276850161)) ;
#15463=CARTESIAN_POINT('Ctrl Pts',(27.8570370437098,38.0792538124217,41.3395108148721)) ;
#15464=CARTESIAN_POINT('Ctrl Pts',(27.7462222287997,40.2140963595073,41.8774304493772)) ;
#15465=CARTESIAN_POINT('Ctrl Pts',(27.6354074138895,41.8282010360107,40.3802412053737)) ;
#15466=CARTESIAN_POINT('Ctrl Pts',(27.5245925989794,41.4520175361157,38.2110488252218)) ;
#15467=CARTESIAN_POINT('Ctrl Pts',(27.4137777840693,39.428039436314,37.3447795853464)) ;
#15468=CARTESIAN_POINT('Ctrl Pts',(27.3029629691591,37.5989837588974,38.5701223869998)) ;
#15469=CARTESIAN_POINT('Ctrl Pts',(27.192148154249,37.6301016629904,40.7714722784283)) ;
#15470=CARTESIAN_POINT('Ctrl Pts',(27.0813333393388,39.4930620800583,41.9446253661672)) ;
#15471=CARTESIAN_POINT('Ctrl Pts',(26.9705185244287,41.491745479404,41.0214924720458)) ;
#15472=CARTESIAN_POINT('Ctrl Pts',(26.8597037095186,41.8064642830042,38.842533604026)) ;
#15473=CARTESIAN_POINT('Ctrl Pts',(26.7488888946084,40.1506849147227,37.3915669059767)) ;
#15474=CARTESIAN_POINT('Ctrl Pts',(26.6380740796983,38.0319003355603,37.9896150486028)) ;
#15475=CARTESIAN_POINT('Ctrl Pts',(26.5272592647882,37.3791434212889,40.0921892054684)) ;
#15476=CARTESIAN_POINT('Ctrl Pts',(26.416444449878,38.7867122240252,41.7850151681516)) ;
#15477=CARTESIAN_POINT('Ctrl Pts',(26.3056296349679,40.9730953891353,41.5268711588974)) ;
#15478=CARTESIAN_POINT('Ctrl Pts',(26.1948148200577,41.9477153719108,39.5527826189801)) ;
#15479=CARTESIAN_POINT('Ctrl Pts',(26.0840000051476,40.8232360990565,37.6600449088926)) ;
#15480=CARTESIAN_POINT('Ctrl Pts',(25.9731851902374,38.6234320058325,37.571888084536)) ;
#15481=CARTESIAN_POINT('Ctrl Pts',(25.8623703753273,37.3510996288709,39.368573921512)) ;
#15482=CARTESIAN_POINT('Ctrl Pts',(25.7515555604171,38.1646252471535,41.4143221324735)) ;
#15483=CARTESIAN_POINT('Ctrl Pts',(25.640740745507,40.3233400457684,41.8465953013074)) ;
#15484=CARTESIAN_POINT('Ctrl Pts',(25.5299259305969,41.8618569543069,40.2718332886862)) ;
#15485=CARTESIAN_POINT('Ctrl Pts',(25.4191111156868,41.3794438141769,38.1237673594179)) ;
#15486=CARTESIAN_POINT('Ctrl Pts',(25.3082963007766,39.3153103573985,37.3580893939119)) ;
#15487=CARTESIAN_POINT('Ctrl Pts',(25.1974814858665,37.5487327209373,38.6719056400471)) ;
#15488=CARTESIAN_POINT('Ctrl Pts',(25.0866666709563,37.6880793876533,40.869061114912)) ;
#15489=CARTESIAN_POINT('Ctrl Pts',(24.9758518560462,39.6064831413471,41.9491706982723)) ;
#15490=CARTESIAN_POINT('Ctrl Pts',(24.865037041136,41.5573464528993,40.9288560341155)) ;
#15491=CARTESIAN_POINT('Ctrl Pts',(24.7542222262259,41.764519211549,38.7370556047135)) ;
#15492=CARTESIAN_POINT('Ctrl Pts',(24.6434074113157,40.0393824012721,37.3692790659172)) ;
#15493=CARTESIAN_POINT('Ctrl Pts',(24.5325925964056,37.95257498919,38.0708091786937)) ;
#15494=CARTESIAN_POINT('Ctrl Pts',(24.4217777814955,37.4040164592344,40.2029426673539)) ;
#15495=CARTESIAN_POINT('Ctrl Pts',(24.3109629665854,38.8931381595526,41.8244932326755)) ;
#15496=CARTESIAN_POINT('Ctrl Pts',(24.2001481516752,41.0641794598153,41.4591312932135)) ;
#15497=CARTESIAN_POINT('Ctrl Pts',(24.0893333367651,41.9405307108,39.4394981188101)) ;
#15498=CARTESIAN_POINT('Ctrl Pts',(23.9785185218549,40.7243239315548,37.6043548698045)) ;
#15499=CARTESIAN_POINT('Ctrl Pts',(23.8677037069448,38.5228462358779,37.6244951203447)) ;
#15500=CARTESIAN_POINT('Ctrl Pts',(23.7568888920346,37.340417880274,39.4815823175755)) ;
#15501=CARTESIAN_POINT('Ctrl Pts',(23.6460740771245,38.2535726445995,41.4848441703134)) ;
#15502=CARTESIAN_POINT('Ctrl Pts',(23.5352592622144,40.4309350418146,41.8104246756579)) ;
#15503=CARTESIAN_POINT('Ctrl Pts',(23.4244444473042,41.8901404233572,40.1619012973779)) ;
#15504=CARTESIAN_POINT('Ctrl Pts',(23.3136296323941,41.302665265992,38.0401608293496)) ;
#15505=CARTESIAN_POINT('Ctrl Pts',(23.2028148174839,39.2033722941205,37.3769273164583)) ;
#15506=CARTESIAN_POINT('Ctrl Pts',(23.0920000025738,37.5035483839543,38.7760371579915)) ;
#15507=CARTESIAN_POINT('Ctrl Pts',(22.9811851876637,37.750786546316,40.9636804024138)) ;
#15508=CARTESIAN_POINT('Ctrl Pts',(22.8703703727535,39.7199904936858,41.948132274746)) ;
#15509=CARTESIAN_POINT('Ctrl Pts',(22.7595555578434,41.6183120087299,40.8331053246757)) ;
#15510=CARTESIAN_POINT('Ctrl Pts',(22.6487407429333,41.7174372998317,38.6337681864242)) ;
#15511=CARTESIAN_POINT('Ctrl Pts',(22.5379259280231,39.9271184237843,37.3524922579445)) ;
#15512=CARTESIAN_POINT('Ctrl Pts',(22.427111113113,37.877338916748,38.1558064187693)) ;
#15513=CARTESIAN_POINT('Ctrl Pts',(22.3162962982028,37.4343064513157,40.3123387944194)) ;
#15514=CARTESIAN_POINT('Ctrl Pts',(22.2054814832926,39.0013769132445,41.8586893083008)) ;
#15515=CARTESIAN_POINT('Ctrl Pts',(22.0946666683825,41.1518217199103,41.3869937060463)) ;
#15516=CARTESIAN_POINT('Ctrl Pts',(21.9838518534724,41.9277832329101,39.3267040979053)) ;
#15517=CARTESIAN_POINT('Ctrl Pts',(21.8730370385623,40.622792470112,37.5535968414076)) ;
#15518=CARTESIAN_POINT('Ctrl Pts',(21.7622222236521,38.4249696113942,37.6819856143904)) ;
#15519=CARTESIAN_POINT('Ctrl Pts',(21.651407408742,37.3353067973815,39.5949790461577)) ;
#15520=CARTESIAN_POINT('Ctrl Pts',(21.5405925938318,38.3458812452266,41.5509067836203)) ;
#15521=CARTESIAN_POINT('Ctrl Pts',(21.4297777789217,40.5366200128897,41.7690050764386)) ;
#15522=CARTESIAN_POINT('Ctrl Pts',(21.3189629640115,41.9129847670933,40.0507133598168)) ;
#15523=CARTESIAN_POINT('Ctrl Pts',(21.2081481491014,41.2218641967656,37.960427488152)) ;
#15524=CARTESIAN_POINT('Ctrl Pts',(21.0973333341913,39.0925031947873,37.4012559465627)) ;
#15525=CARTESIAN_POINT('Ctrl Pts',(20.9865185192811,37.4635260875702,38.8822485573436)) ;
#15526=CARTESIAN_POINT('Ctrl Pts',(20.875703704371,37.8180993714967,41.0551337957205)) ;
#15527=CARTESIAN_POINT('Ctrl Pts',(20.7648888894609,39.8332534757639,41.9414473616958)) ;
#15528=CARTESIAN_POINT('Ctrl Pts',(20.6540740745507,41.6746063303626,40.7346024308416)) ;
#15529=CARTESIAN_POINT('Ctrl Pts',(20.5432592596406,41.6651092776103,38.5326609143414)) ;
#15530=CARTESIAN_POINT('Ctrl Pts',(20.4324444447304,39.814610819179,37.3417681053347)) ;
#15531=CARTESIAN_POINT('Ctrl Pts',(20.3216296298203,37.8054802267138,38.2433498381838)) ;
#15532=CARTESIAN_POINT('Ctrl Pts',(20.2108148149101,37.4717648473903,40.4223362571249)) ;
#15533=CARTESIAN_POINT('Ctrl Pts',(20.1369382716367,38.561997188093,41.394603313221)) ;
#15534=CARTESIAN_POINT('Ctrl Pts',(20.1,39.1924719723276,41.5436925123374)) ;
#15535=CARTESIAN_POINT('Ctrl Pts',(29.5533827215147,41.1245055761783,38.5842002042185)) ;
#15536=CARTESIAN_POINT('Ctrl Pts',(29.516444449878,40.7737395226631,38.0927098462256)) ;
#15537=CARTESIAN_POINT('Ctrl Pts',(29.4425679066046,39.5507038383217,37.4945228523954)) ;
#15538=CARTESIAN_POINT('Ctrl Pts',(29.3317530916944,37.7880995125941,38.5501512572853)) ;
#15539=CARTESIAN_POINT('Ctrl Pts',(29.2209382767843,37.7179892031665,40.6013988613999)) ;
#15540=CARTESIAN_POINT('Ctrl Pts',(29.1101234618742,39.3975183817629,41.7785705068217)) ;
#15541=CARTESIAN_POINT('Ctrl Pts',(28.999308646964,41.3008467182311,41.0110014608924)) ;
#15542=CARTESIAN_POINT('Ctrl Pts',(28.8884938320539,41.6934681368296,38.9969767509505)) ;
#15543=CARTESIAN_POINT('Ctrl Pts',(28.7776790171438,40.2187406437018,37.5704232015323)) ;
#15544=CARTESIAN_POINT('Ctrl Pts',(28.6668642022336,38.2189105576076,38.0300006039852)) ;
#15545=CARTESIAN_POINT('Ctrl Pts',(28.5560493873235,37.5149143017061,39.9573579977613)) ;
#15546=CARTESIAN_POINT('Ctrl Pts',(28.4452345724133,38.7475978859959,41.5977119666809)) ;
#15547=CARTESIAN_POINT('Ctrl Pts',(28.3344197575032,40.7947243393968,41.4576305737739)) ;
#15548=CARTESIAN_POINT('Ctrl Pts',(28.223604942593,41.7924757348056,39.6646414141626)) ;
#15549=CARTESIAN_POINT('Ctrl Pts',(28.1127901276829,40.8324690285507,37.8511634396112)) ;
#15550=CARTESIAN_POINT('Ctrl Pts',(28.0019753127728,38.7887292960491,37.6682630817799)) ;
#15551=CARTESIAN_POINT('Ctrl Pts',(27.8911604978626,37.521968572182,39.2824617883217)) ;
#15552=CARTESIAN_POINT('Ctrl Pts',(27.7803456829525,38.1854988485539,41.2241228903294)) ;
#15553=CARTESIAN_POINT('Ctrl Pts',(27.6695308680424,40.1752143477012,41.7254746342936)) ;
#15554=CARTESIAN_POINT('Ctrl Pts',(27.5587160531322,41.6795918468614,40.3300646318007)) ;
#15555=CARTESIAN_POINT('Ctrl Pts',(27.4479012382221,41.328981380864,38.308334408505)) ;
#15556=CARTESIAN_POINT('Ctrl Pts',(27.3370864233119,39.4425937404228,37.5009543347999)) ;
#15557=CARTESIAN_POINT('Ctrl Pts',(27.2262716084018,37.7378776548606,38.6429980735978)) ;
#15558=CARTESIAN_POINT('Ctrl Pts',(27.1154567934916,37.7668801572509,40.6946997337513)) ;
#15559=CARTESIAN_POINT('Ctrl Pts',(27.0046419785815,39.503196131091,41.7881016264263)) ;
#15560=CARTESIAN_POINT('Ctrl Pts',(26.8938271636713,41.3660086101638,40.9277235017194)) ;
#15561=CARTESIAN_POINT('Ctrl Pts',(26.7830123487612,41.6593327629223,38.8968907184669)) ;
#15562=CARTESIAN_POINT('Ctrl Pts',(26.6721975338511,40.1161136263466,37.5445610434767)) ;
#15563=CARTESIAN_POINT('Ctrl Pts',(26.5613827189409,38.1413644710663,38.1019537468609)) ;
#15564=CARTESIAN_POINT('Ctrl Pts',(26.4505679040308,37.532982109906,40.0615944677811)) ;
#15565=CARTESIAN_POINT('Ctrl Pts',(26.3397530891206,38.8448640876866,41.6393417634346)) ;
#15566=CARTESIAN_POINT('Ctrl Pts',(26.2289382742105,40.8826164627426,41.3987464385351)) ;
#15567=CARTESIAN_POINT('Ctrl Pts',(26.1181234593003,41.7909815729259,39.5588568551441)) ;
#15568=CARTESIAN_POINT('Ctrl Pts',(26.0073086443903,40.7429446389034,37.7947878549628)) ;
#15569=CARTESIAN_POINT('Ctrl Pts',(25.8964938294801,38.6926836932656,37.7126239501739)) ;
#15570=CARTESIAN_POINT('Ctrl Pts',(25.78567901457,37.5068447404287,39.3871707038959)) ;
#15571=CARTESIAN_POINT('Ctrl Pts',(25.6748641996598,38.2650667150938,41.2938485187352)) ;
#15572=CARTESIAN_POINT('Ctrl Pts',(25.5640493847497,40.2770316250618,41.6967356661122)) ;
#15573=CARTESIAN_POINT('Ctrl Pts',(25.4532345698395,41.7109598287124,40.2290263082214)) ;
#15574=CARTESIAN_POINT('Ctrl Pts',(25.3424197549294,41.2613412358943,38.2269863552092)) ;
#15575=CARTESIAN_POINT('Ctrl Pts',(25.2316049400193,39.3375280081377,37.5133593397636)) ;
#15576=CARTESIAN_POINT('Ctrl Pts',(25.1207901251091,37.6910426930908,38.7378620795726)) ;
#15577=CARTESIAN_POINT('Ctrl Pts',(25.009975310199,37.820916543927,40.7856544604875)) ;
#15578=CARTESIAN_POINT('Ctrl Pts',(24.8991604952888,39.6089068046413,41.7923379658934)) ;
#15579=CARTESIAN_POINT('Ctrl Pts',(24.7883456803787,41.4271500156042,40.8413845084351)) ;
#15580=CARTESIAN_POINT('Ctrl Pts',(24.6775308654685,41.6202391262972,38.7985831358596)) ;
#15581=CARTESIAN_POINT('Ctrl Pts',(24.5667160505584,40.0123774813045,37.5237883354991)) ;
#15582=CARTESIAN_POINT('Ctrl Pts',(24.4559012356483,38.0674316785221,38.177628282813)) ;
#15583=CARTESIAN_POINT('Ctrl Pts',(24.3450864207381,37.5561642734705,40.1648188858998)) ;
#15584=CARTESIAN_POINT('Ctrl Pts',(24.234271605828,38.9440551656044,41.6761361007812)) ;
#15585=CARTESIAN_POINT('Ctrl Pts',(24.1234567909178,40.9675086190306,41.3356115432495)) ;
#15586=CARTESIAN_POINT('Ctrl Pts',(24.0126419760077,41.7842853265972,39.4532734592589)) ;
#15587=CARTESIAN_POINT('Ctrl Pts',(23.9018271610975,40.6507565414716,37.7428836365121)) ;
#15588=CARTESIAN_POINT('Ctrl Pts',(23.7910123461874,38.5989357652295,37.7616547485602)) ;
#15589=CARTESIAN_POINT('Ctrl Pts',(23.6801975312773,37.496889139361,39.4924967652901)) ;
#15590=CARTESIAN_POINT('Ctrl Pts',(23.5693827163671,38.3479674496463,41.3595764535251)) ;
#15591=CARTESIAN_POINT('Ctrl Pts',(23.458567901457,40.377312290517,41.6630239272456)) ;
#15592=CARTESIAN_POINT('Ctrl Pts',(23.3477530865469,41.7373205815539,40.1265675169364)) ;
#15593=CARTESIAN_POINT('Ctrl Pts',(23.2369382716367,41.1897821096561,38.1490634147404)) ;
#15594=CARTESIAN_POINT('Ctrl Pts',(23.1261234567266,39.2331995180799,37.5309166563505)) ;
#15595=CARTESIAN_POINT('Ctrl Pts',(23.0153086418164,37.6489299968938,38.8349147149)) ;
#15596=CARTESIAN_POINT('Ctrl Pts',(22.9044938269063,37.8793608566794,40.87384150881)) ;
#15597=CARTESIAN_POINT('Ctrl Pts',(22.7936790119962,39.7146979031575,41.7913701346181)) ;
#15598=CARTESIAN_POINT('Ctrl Pts',(22.682864197086,41.4839711200533,40.7521429524774)) ;
#15599=CARTESIAN_POINT('Ctrl Pts',(22.5720493821759,41.5763578528978,38.7023172181142)) ;
#15600=CARTESIAN_POINT('Ctrl Pts',(22.4612345672657,39.9077452327537,37.5081426982832)) ;
#15601=CARTESIAN_POINT('Ctrl Pts',(22.3504197523556,37.9973101701995,38.2568473925287)) ;
#15602=CARTESIAN_POINT('Ctrl Pts',(22.2396049374455,37.5843951454828,40.2667782411066)) ;
#15603=CARTESIAN_POINT('Ctrl Pts',(22.1287901225353,39.0449358259243,41.708007519952)) ;
#15604=CARTESIAN_POINT('Ctrl Pts',(22.0179753076252,41.0491929397452,41.2683778845173)) ;
#15605=CARTESIAN_POINT('Ctrl Pts',(21.907160492715,41.7724044249507,39.3481471997548)) ;
#15606=CARTESIAN_POINT('Ctrl Pts',(21.7963456778049,40.5561272102548,37.6955761496225)) ;
#15607=CARTESIAN_POINT('Ctrl Pts',(21.6855308628947,38.5077128143823,37.8152370266596)) ;
#15608=CARTESIAN_POINT('Ctrl Pts',(21.5747160479846,37.4921255089646,39.5981847602763)) ;
#15609=CARTESIAN_POINT('Ctrl Pts',(21.4639012330745,38.4340008920765,41.421148116405)) ;
#15610=CARTESIAN_POINT('Ctrl Pts',(21.3530864181644,40.4758127749028,41.6244200411428)) ;
#15611=CARTESIAN_POINT('Ctrl Pts',(21.2422716032542,41.7586119619704,40.0229381588904)) ;
#15612=CARTESIAN_POINT('Ctrl Pts',(21.1314567883441,41.1144739142077,38.0747503629435)) ;
#15613=CARTESIAN_POINT('Ctrl Pts',(21.0206419734339,39.1298673235717,37.5535914210342)) ;
#15614=CARTESIAN_POINT('Ctrl Pts',(20.9098271585238,37.6116284246838,38.9339058408569)) ;
#15615=CARTESIAN_POINT('Ctrl Pts',(20.7990123436136,37.9420977417654,40.9590778810945)) ;
#15616=CARTESIAN_POINT('Ctrl Pts',(20.6881975287035,39.8202612437552,41.7851396633712)) ;
#15617=CARTESIAN_POINT('Ctrl Pts',(20.5773827137933,41.5364385417934,40.6603363062026)) ;
#15618=CARTESIAN_POINT('Ctrl Pts',(20.4665678988832,41.5275871006961,38.6080832397749)) ;
#15619=CARTESIAN_POINT('Ctrl Pts',(20.355753083973,39.8028859189084,37.4981475758365)) ;
#15620=CARTESIAN_POINT('Ctrl Pts',(20.2449382690629,37.9303364491143,38.3384395917731)) ;
#15621=CARTESIAN_POINT('Ctrl Pts',(20.1341234541528,37.6193071118685,40.3692980530295)) ;
#15622=CARTESIAN_POINT('Ctrl Pts',(20.0602469108794,38.6354252274314,41.2754701889866)) ;
#15623=CARTESIAN_POINT('Ctrl Pts',(20.0233086392427,39.2230402024682,41.41442427281)) ;
#15624=CARTESIAN_POINT('Ctrl Pts',(29.4766913607574,41.0163835983161,38.6613645246497)) ;
#15625=CARTESIAN_POINT('Ctrl Pts',(29.4397530891207,40.6912019270331,38.205722781585)) ;
#15626=CARTESIAN_POINT('Ctrl Pts',(29.3658765458472,39.5573727440571,37.6511667051229)) ;
#15627=CARTESIAN_POINT('Ctrl Pts',(29.2550617309371,37.9233302969426,38.6297990599812)) ;
#15628=CARTESIAN_POINT('Ctrl Pts',(29.144246916027,37.8583337348028,40.531431551029)) ;
#15629=CARTESIAN_POINT('Ctrl Pts',(29.0334321011168,39.4153604190877,41.6227419535296)) ;
#15630=CARTESIAN_POINT('Ctrl Pts',(28.9226172862066,41.1798626656718,40.9111583134396)) ;
#15631=CARTESIAN_POINT('Ctrl Pts',(28.8118024712965,41.5438468306211,39.0440337310553)) ;
#15632=CARTESIAN_POINT('Ctrl Pts',(28.7009876563864,40.1766838851298,37.7215309896254)) ;
#15633=CARTESIAN_POINT('Ctrl Pts',(28.5901728414763,38.3227185907092,38.1475874632089)) ;
#15634=CARTESIAN_POINT('Ctrl Pts',(28.4793580265661,37.6700708308224,39.9343661214822)) ;
#15635=CARTESIAN_POINT('Ctrl Pts',(28.368543211656,38.8128442095042,41.4550749807441)) ;
#15636=CARTESIAN_POINT('Ctrl Pts',(28.2577283967458,40.7106561407708,41.325210927468)) ;
#15637=CARTESIAN_POINT('Ctrl Pts',(28.1469135818357,41.6356329537562,39.6629998734859)) ;
#15638=CARTESIAN_POINT('Ctrl Pts',(28.0360987669255,40.7456477854244,37.981794429887)) ;
#15639=CARTESIAN_POINT('Ctrl Pts',(27.9252839520154,38.8509755524015,37.8122345667194)) ;
#15640=CARTESIAN_POINT('Ctrl Pts',(27.8144691371052,37.6766105727388,39.3086958916275)) ;
#15641=CARTESIAN_POINT('Ctrl Pts',(27.7036543221951,38.291743884686,41.1087349657866)) ;
#15642=CARTESIAN_POINT('Ctrl Pts',(27.592839507285,40.1363323358952,41.57351881921)) ;
#15643=CARTESIAN_POINT('Ctrl Pts',(27.4820246923748,41.5309826577121,40.2798880582278)) ;
#15644=CARTESIAN_POINT('Ctrl Pts',(27.3712098774647,41.2059452256123,38.4056199917881)) ;
#15645=CARTESIAN_POINT('Ctrl Pts',(27.2603950625546,39.4571480445315,37.6571290842533)) ;
#15646=CARTESIAN_POINT('Ctrl Pts',(27.1495802476444,37.8767715508238,38.7158737601958)) ;
#15647=CARTESIAN_POINT('Ctrl Pts',(27.0387654327343,37.9036586515114,40.6179271890742)) ;
#15648=CARTESIAN_POINT('Ctrl Pts',(26.9279506178242,39.5133301821237,41.6315778866856)) ;
#15649=CARTESIAN_POINT('Ctrl Pts',(26.817135802914,41.2402717409236,40.8339545313929)) ;
#15650=CARTESIAN_POINT('Ctrl Pts',(26.7063209880039,41.5122012428404,38.9512478329077)) ;
#15651=CARTESIAN_POINT('Ctrl Pts',(26.5955061730937,40.0815423379706,37.6975551809767)) ;
#15652=CARTESIAN_POINT('Ctrl Pts',(26.4846913581836,38.2508286065723,38.2142924451189)) ;
#15653=CARTESIAN_POINT('Ctrl Pts',(26.3738765432735,37.686820798523,40.030999730094)) ;
#15654=CARTESIAN_POINT('Ctrl Pts',(26.2630617283633,38.9030159513479,41.4936683587175)) ;
#15655=CARTESIAN_POINT('Ctrl Pts',(26.1522469134532,40.7921375363501,41.2706217181728)) ;
#15656=CARTESIAN_POINT('Ctrl Pts',(26.041432098543,41.6342477739409,39.564931091308)) ;
#15657=CARTESIAN_POINT('Ctrl Pts',(25.9306172836329,40.6626531787504,37.9295308010329)) ;
#15658=CARTESIAN_POINT('Ctrl Pts',(25.8198024687227,38.7619353806986,37.8533598158118)) ;
#15659=CARTESIAN_POINT('Ctrl Pts',(25.7089876538126,37.6625898519865,39.4057674862797)) ;
#15660=CARTESIAN_POINT('Ctrl Pts',(25.5981728389024,38.3655081830341,41.173374904997)) ;
#15661=CARTESIAN_POINT('Ctrl Pts',(25.4873580239923,40.2307232043552,41.546876030917)) ;
#15662=CARTESIAN_POINT('Ctrl Pts',(25.3765432090821,41.5600627031181,40.1862193277566)) ;
#15663=CARTESIAN_POINT('Ctrl Pts',(25.2657283941721,41.1432386576117,38.3302053510005)) ;
#15664=CARTESIAN_POINT('Ctrl Pts',(25.1549135792619,39.359745658877,37.6686292856154)) ;
#15665=CARTESIAN_POINT('Ctrl Pts',(25.0440987643518,37.8333526652442,38.803818519098)) ;
#15666=CARTESIAN_POINT('Ctrl Pts',(24.9332839494416,37.9537537002008,40.7022478060632)) ;
#15667=CARTESIAN_POINT('Ctrl Pts',(24.8224691345315,39.6113304679353,41.6355052335146)) ;
#15668=CARTESIAN_POINT('Ctrl Pts',(24.7116543196213,41.2969535783092,40.7539129827547)) ;
#15669=CARTESIAN_POINT('Ctrl Pts',(24.6008395047112,41.4759590410456,38.8601106670057)) ;
#15670=CARTESIAN_POINT('Ctrl Pts',(24.490024689801,39.9853725613369,37.6782976050809)) ;
#15671=CARTESIAN_POINT('Ctrl Pts',(24.3792098748909,38.1822883678541,38.2844473869324)) ;
#15672=CARTESIAN_POINT('Ctrl Pts',(24.2683950599807,37.7083120877066,40.1266951044458)) ;
#15673=CARTESIAN_POINT('Ctrl Pts',(24.1575802450706,38.994972171656,41.5277789688869)) ;
#15674=CARTESIAN_POINT('Ctrl Pts',(24.0467654301605,40.870837778246,41.2120917932856)) ;
#15675=CARTESIAN_POINT('Ctrl Pts',(23.9359506152503,41.6280399423943,39.4670487997076)) ;
#15676=CARTESIAN_POINT('Ctrl Pts',(23.8251358003402,40.5771891513884,37.8814124032197)) ;
#15677=CARTESIAN_POINT('Ctrl Pts',(23.71432098543,38.6750252945812,37.8988143767757)) ;
#15678=CARTESIAN_POINT('Ctrl Pts',(23.6035061705199,37.6533603984479,39.5034112130047)) ;
#15679=CARTESIAN_POINT('Ctrl Pts',(23.4926913556098,38.4423622546929,41.2343087367368)) ;
#15680=CARTESIAN_POINT('Ctrl Pts',(23.3818765406997,40.3236895392195,41.5156231788333)) ;
#15681=CARTESIAN_POINT('Ctrl Pts',(23.2710617257895,41.5845007397505,40.0912337364948)) ;
#15682=CARTESIAN_POINT('Ctrl Pts',(23.1602469108794,41.0768989533203,38.2579660001312)) ;
#15683=CARTESIAN_POINT('Ctrl Pts',(23.0494320959692,39.2630267420392,37.6849059962426)) ;
#15684=CARTESIAN_POINT('Ctrl Pts',(22.9386172810591,37.7943116098333,38.8937922718084)) ;
#15685=CARTESIAN_POINT('Ctrl Pts',(22.827802466149,38.0079351670427,40.7840026152063)) ;
#15686=CARTESIAN_POINT('Ctrl Pts',(22.7169876512388,39.7094053126292,41.6346079944903)) ;
#15687=CARTESIAN_POINT('Ctrl Pts',(22.6061728363287,41.3496302313767,40.6711805802791)) ;
#15688=CARTESIAN_POINT('Ctrl Pts',(22.4953580214185,41.435278405964,38.7708662498041)) ;
#15689=CARTESIAN_POINT('Ctrl Pts',(22.3845432065084,39.8883720417231,37.663793138622)) ;
#15690=CARTESIAN_POINT('Ctrl Pts',(22.2737283915983,38.117281423651,38.357888366288)) ;
#15691=CARTESIAN_POINT('Ctrl Pts',(22.1629135766881,37.7344838396499,40.2212176877939)) ;
#15692=CARTESIAN_POINT('Ctrl Pts',(22.0520987617779,39.088494738604,41.5573257316031)) ;
#15693=CARTESIAN_POINT('Ctrl Pts',(21.9412839468678,40.9465641595803,41.1497620629884)) ;
#15694=CARTESIAN_POINT('Ctrl Pts',(21.8304691319577,41.6170256169913,39.3695903016042)) ;
#15695=CARTESIAN_POINT('Ctrl Pts',(21.7196543170475,40.4894619503976,37.8375554578374)) ;
#15696=CARTESIAN_POINT('Ctrl Pts',(21.6088395021374,38.5904560173703,37.9484884389288)) ;
#15697=CARTESIAN_POINT('Ctrl Pts',(21.4980246872273,37.6489442205477,39.6013904743948)) ;
#15698=CARTESIAN_POINT('Ctrl Pts',(21.3872098723171,38.5221205389264,41.2913894491898)) ;
#15699=CARTESIAN_POINT('Ctrl Pts',(21.276395057407,40.4150055369158,41.479835005847)) ;
#15700=CARTESIAN_POINT('Ctrl Pts',(21.1655802424968,41.6042391568477,39.9951629579641)) ;
#15701=CARTESIAN_POINT('Ctrl Pts',(21.0547654275867,41.0070836316498,38.1890732377351)) ;
#15702=CARTESIAN_POINT('Ctrl Pts',(20.9439506126765,39.167231452356,37.7059268955056)) ;
#15703=CARTESIAN_POINT('Ctrl Pts',(20.8331357977664,37.7597307617974,38.9855631243703)) ;
#15704=CARTESIAN_POINT('Ctrl Pts',(20.7223209828563,38.0660961120341,40.8630219664685)) ;
#15705=CARTESIAN_POINT('Ctrl Pts',(20.6115061679461,39.8072690117465,41.6288319650465)) ;
#15706=CARTESIAN_POINT('Ctrl Pts',(20.500691353036,41.3982707532242,40.5860701815637)) ;
#15707=CARTESIAN_POINT('Ctrl Pts',(20.3898765381259,41.3900649237819,38.6835055652085)) ;
#15708=CARTESIAN_POINT('Ctrl Pts',(20.2790617232157,39.7911610186378,37.6545270463381)) ;
#15709=CARTESIAN_POINT('Ctrl Pts',(20.1682469083056,38.0551926715147,38.4335293453624)) ;
#15710=CARTESIAN_POINT('Ctrl Pts',(20.0574320933955,37.7668493763468,40.3162598489341)) ;
#15711=CARTESIAN_POINT('Ctrl Pts',(19.983555550122,38.7088532667698,41.1563370647523)) ;
#15712=CARTESIAN_POINT('Ctrl Pts',(19.9466172784853,39.2536084326088,41.2851560332826)) ;
#15713=CARTESIAN_POINT('Ctrl Pts',(29.4,40.9082616204539,38.7385288450808)) ;
#15714=CARTESIAN_POINT('Ctrl Pts',(29.3630617283633,40.6086643314031,38.3187357169443)) ;
#15715=CARTESIAN_POINT('Ctrl Pts',(29.2891851850898,39.5640416497925,37.8078105578506)) ;
#15716=CARTESIAN_POINT('Ctrl Pts',(29.1783703701797,38.0585610812911,38.709446862677)) ;
#15717=CARTESIAN_POINT('Ctrl Pts',(29.0675555552696,37.9986782664391,40.4614642406582)) ;
#15718=CARTESIAN_POINT('Ctrl Pts',(28.9567407403595,39.4332024564126,41.4669134002374)) ;
#15719=CARTESIAN_POINT('Ctrl Pts',(28.8459259254493,41.0588786131123,40.8113151659867)) ;
#15720=CARTESIAN_POINT('Ctrl Pts',(28.7351111105392,41.3942255244127,39.0910907111602)) ;
#15721=CARTESIAN_POINT('Ctrl Pts',(28.624296295629,40.1346271265577,37.8726387777184)) ;
#15722=CARTESIAN_POINT('Ctrl Pts',(28.5134814807189,38.4265266238107,38.2651743224326)) ;
#15723=CARTESIAN_POINT('Ctrl Pts',(28.4026666658087,37.8252273599387,39.911374245203)) ;
#15724=CARTESIAN_POINT('Ctrl Pts',(28.2918518508986,38.8780905330125,41.3124379948074)) ;
#15725=CARTESIAN_POINT('Ctrl Pts',(28.1810370359884,40.6265879421449,41.1927912811621)) ;
#15726=CARTESIAN_POINT('Ctrl Pts',(28.0702222210783,41.4787901727068,39.6613583328092)) ;
#15727=CARTESIAN_POINT('Ctrl Pts',(27.9594074061682,40.6588265422981,38.1124254201628)) ;
#15728=CARTESIAN_POINT('Ctrl Pts',(27.848592591258,38.9132218087539,37.956206051659)) ;
#15729=CARTESIAN_POINT('Ctrl Pts',(27.7377777763479,37.8312525732956,39.3349299949331)) ;
#15730=CARTESIAN_POINT('Ctrl Pts',(27.6269629614378,38.3979889208182,40.9933470412438)) ;
#15731=CARTESIAN_POINT('Ctrl Pts',(27.5161481465276,40.0974503240892,41.4215630041264)) ;
#15732=CARTESIAN_POINT('Ctrl Pts',(27.4053333316175,41.3823734685628,40.2297114846548)) ;
#15733=CARTESIAN_POINT('Ctrl Pts',(27.2945185167073,41.0829090703606,38.5029055750713)) ;
#15734=CARTESIAN_POINT('Ctrl Pts',(27.1837037017972,39.4717023486403,37.8133038337068)) ;
#15735=CARTESIAN_POINT('Ctrl Pts',(27.0728888868871,38.0156654467869,38.7887494467938)) ;
#15736=CARTESIAN_POINT('Ctrl Pts',(26.9620740719769,38.0404371457719,40.5411546443971)) ;
#15737=CARTESIAN_POINT('Ctrl Pts',(26.8512592570668,39.5234642331564,41.4750541469447)) ;
#15738=CARTESIAN_POINT('Ctrl Pts',(26.7404444421566,41.1145348716835,40.7401855610665)) ;
#15739=CARTESIAN_POINT('Ctrl Pts',(26.6296296272465,41.3650697227584,39.0056049473486)) ;
#15740=CARTESIAN_POINT('Ctrl Pts',(26.5188148123364,40.0469710495945,37.8505493184767)) ;
#15741=CARTESIAN_POINT('Ctrl Pts',(26.4079999974262,38.3602927420783,38.3266311433769)) ;
#15742=CARTESIAN_POINT('Ctrl Pts',(26.2971851825161,37.8406594871401,40.0004049924068)) ;
#15743=CARTESIAN_POINT('Ctrl Pts',(26.1863703676059,38.9611678150092,41.3479949540004)) ;
#15744=CARTESIAN_POINT('Ctrl Pts',(26.0755555526958,40.7016586099574,41.1424969978105)) ;
#15745=CARTESIAN_POINT('Ctrl Pts',(25.9647407377856,41.477513974956,39.571005327472)) ;
#15746=CARTESIAN_POINT('Ctrl Pts',(25.8539259228755,40.5823617185973,38.064273747103)) ;
#15747=CARTESIAN_POINT('Ctrl Pts',(25.7431111079654,38.8311870681316,37.9940956814497)) ;
#15748=CARTESIAN_POINT('Ctrl Pts',(25.6322962930552,37.8183349635443,39.4243642686637)) ;
#15749=CARTESIAN_POINT('Ctrl Pts',(25.5214814781451,38.4659496509744,41.0529012912587)) ;
#15750=CARTESIAN_POINT('Ctrl Pts',(25.410666663235,40.1844147836487,41.3970163957218)) ;
#15751=CARTESIAN_POINT('Ctrl Pts',(25.2998518483248,41.4091655775236,40.1434123472918)) ;
#15752=CARTESIAN_POINT('Ctrl Pts',(25.1890370334147,41.0251360793291,38.4334243467918)) ;
#15753=CARTESIAN_POINT('Ctrl Pts',(25.0782222185045,39.3819633096162,37.8238992314671)) ;
#15754=CARTESIAN_POINT('Ctrl Pts',(24.9674074035944,37.9756626373976,38.8697749586234)) ;
#15755=CARTESIAN_POINT('Ctrl Pts',(24.8565925886842,38.0865908564746,40.6188411516388)) ;
#15756=CARTESIAN_POINT('Ctrl Pts',(24.7457777737741,39.6137541312294,41.4786725011358)) ;
#15757=CARTESIAN_POINT('Ctrl Pts',(24.634962958864,41.1667571410141,40.6664414570744)) ;
#15758=CARTESIAN_POINT('Ctrl Pts',(24.5241481439538,41.3316789557939,38.9216381981518)) ;
#15759=CARTESIAN_POINT('Ctrl Pts',(24.4133333290437,39.9583676413693,37.8328068746627)) ;
#15760=CARTESIAN_POINT('Ctrl Pts',(24.3025185141336,38.2971450571862,38.3912664910517)) ;
#15761=CARTESIAN_POINT('Ctrl Pts',(24.1917036992234,37.8604599019426,40.0885713229918)) ;
#15762=CARTESIAN_POINT('Ctrl Pts',(24.0808888843133,39.0458891777078,41.3794218369926)) ;
#15763=CARTESIAN_POINT('Ctrl Pts',(23.9700740694031,40.7741669374613,41.0885720433216)) ;
#15764=CARTESIAN_POINT('Ctrl Pts',(23.859259254493,41.4717945581916,39.4808241401565)) ;
#15765=CARTESIAN_POINT('Ctrl Pts',(23.7484444395829,40.5036217613051,38.0199411699272)) ;
#15766=CARTESIAN_POINT('Ctrl Pts',(23.6376296246727,38.7511148239329,38.0359740049913)) ;
#15767=CARTESIAN_POINT('Ctrl Pts',(23.5268148097626,37.8098316575348,39.5143256607193)) ;
#15768=CARTESIAN_POINT('Ctrl Pts',(23.4159999948524,38.5367570597397,41.1090410199485)) ;
#15769=CARTESIAN_POINT('Ctrl Pts',(23.3051851799423,40.2700667879219,41.368222430421)) ;
#15770=CARTESIAN_POINT('Ctrl Pts',(23.1943703650321,41.4316808979472,40.0558999560533)) ;
#15771=CARTESIAN_POINT('Ctrl Pts',(23.083555550122,40.9640157969843,38.366868585522)) ;
#15772=CARTESIAN_POINT('Ctrl Pts',(22.9727407352119,39.2928539659985,37.8388953361349)) ;
#15773=CARTESIAN_POINT('Ctrl Pts',(22.8619259203017,37.9396932227727,38.9526698287169)) ;
#15774=CARTESIAN_POINT('Ctrl Pts',(22.7511111053916,38.136509477406,40.6941637216025)) ;
#15775=CARTESIAN_POINT('Ctrl Pts',(22.6402962904815,39.7041127221009,41.4778458543625)) ;
#15776=CARTESIAN_POINT('Ctrl Pts',(22.5294814755713,41.2152893427001,40.5902182080807)) ;
#15777=CARTESIAN_POINT('Ctrl Pts',(22.4186666606612,41.2941989590302,38.8394152814942)) ;
#15778=CARTESIAN_POINT('Ctrl Pts',(22.307851845751,39.8689988506925,37.8194435789608)) ;
#15779=CARTESIAN_POINT('Ctrl Pts',(22.1970370308409,38.2372526771025,38.4589293400473)) ;
#15780=CARTESIAN_POINT('Ctrl Pts',(22.0862222159307,37.884572533817,40.1756571344811)) ;
#15781=CARTESIAN_POINT('Ctrl Pts',(21.9754074010206,39.1320536512838,41.4066439432543)) ;
#15782=CARTESIAN_POINT('Ctrl Pts',(21.8645925861105,40.8439353794152,41.0311462414594)) ;
#15783=CARTESIAN_POINT('Ctrl Pts',(21.7537777712003,41.4616468090319,39.3910334034537)) ;
#15784=CARTESIAN_POINT('Ctrl Pts',(21.6429629562902,40.4227966905405,37.9795347660523)) ;
#15785=CARTESIAN_POINT('Ctrl Pts',(21.53214814138,38.6731992203584,38.0817398511981)) ;
#15786=CARTESIAN_POINT('Ctrl Pts',(21.4213333264699,37.8057629321309,39.6045961885133)) ;
#15787=CARTESIAN_POINT('Ctrl Pts',(21.3105185115597,38.6102401857762,41.1616307819746)) ;
#15788=CARTESIAN_POINT('Ctrl Pts',(21.1997036966497,40.3541982989288,41.3352499705511)) ;
#15789=CARTESIAN_POINT('Ctrl Pts',(21.0888888817395,41.4498663517249,39.9673877570378)) ;
#15790=CARTESIAN_POINT('Ctrl Pts',(20.9780740668294,40.8996933490919,38.3033961125266)) ;
#15791=CARTESIAN_POINT('Ctrl Pts',(20.8672592519192,39.2045955811405,37.8582623699771)) ;
#15792=CARTESIAN_POINT('Ctrl Pts',(20.7564444370091,37.907833098911,39.0372204078837)) ;
#15793=CARTESIAN_POINT('Ctrl Pts',(20.6456296220989,38.1900944823029,40.7669660518425)) ;
#15794=CARTESIAN_POINT('Ctrl Pts',(20.5348148071888,39.7942767797378,41.4725242667218)) ;
#15795=CARTESIAN_POINT('Ctrl Pts',(20.4239999922786,41.260102964655,40.5118040569248)) ;
#15796=CARTESIAN_POINT('Ctrl Pts',(20.3131851773685,41.2525427468677,38.758927890642)) ;
#15797=CARTESIAN_POINT('Ctrl Pts',(20.2023703624584,39.7794361183673,37.8109065168399)) ;
#15798=CARTESIAN_POINT('Ctrl Pts',(20.0915555475482,38.1800488939151,38.5286190989517)) ;
#15799=CARTESIAN_POINT('Ctrl Pts',(19.9807407326381,37.9143916408252,40.2632216448386)) ;
#15800=CARTESIAN_POINT('Ctrl Pts',(19.9068641893647,38.7822813061082,41.0372039405179)) ;
#15801=CARTESIAN_POINT('Ctrl Pts',(19.8699259177279,39.2841766627494,41.1558877937552)) ;
#15802=CARTESIAN_POINT('Origin',(29.4,39.642135623731,39.642135623731)) ;
#15803=CARTESIAN_POINT('',(29.6,39.642135623731,41.796135623731)) ;
#15804=CARTESIAN_POINT('Origin',(29.4,39.642135623731,41.796135623731)) ;
#15805=CARTESIAN_POINT('Origin',(29.6,39.642135623731,39.642135623731)) ;
#15806=CARTESIAN_POINT('Origin',(29.6,39.642135623731,39.642135623731)) ;
#15807=CARTESIAN_POINT('Origin',(20.1,39.642135623731,39.642135623731)) ;
#15808=CARTESIAN_POINT('Origin',(29.6,39.642135623731,39.642135623731)) ;
#15809=CARTESIAN_POINT('',(29.6,39.642135623731,42.9421356237309)) ;
#15810=CARTESIAN_POINT('Origin',(29.6,39.642135623731,39.642135623731)) ;
#15811=CARTESIAN_POINT('Origin',(19.85,39.642135623731,39.642135623731)) ;
#15812=CARTESIAN_POINT('',(19.6,39.642135623731,41.096135623731)) ;
#15813=CARTESIAN_POINT('',(19.85,39.642135623731,41.346135623731)) ;
#15814=CARTESIAN_POINT('Origin',(19.6,39.642135623731,39.642135623731)) ;
#15815=CARTESIAN_POINT('Origin',(19.6,39.642135623731,39.642135623731)) ;
#15816=CARTESIAN_POINT('Origin',(33.6,42.9412415963219,40.2238570189152)) ;
#15817=CARTESIAN_POINT('',(33.35,42.9412415963219,40.2238570189152)) ;
#15818=CARTESIAN_POINT('',(33.2,43.0755441166495,40.321625226856)) ;
#15819=CARTESIAN_POINT('Ctrl Pts',(33.35,42.9412415963219,40.2238570189152)) ;
#15820=CARTESIAN_POINT('Ctrl Pts',(33.2770142912005,43.0069223909349,40.2716706680543)) ;
#15821=CARTESIAN_POINT('Ctrl Pts',(33.2,43.0755441166495,40.321625226856)) ;
#15822=CARTESIAN_POINT('',(30.2,42.9412415963219,40.2238570189152)) ;
#15823=CARTESIAN_POINT('',(33.6,42.9412415963219,40.2238570189152)) ;
#15824=CARTESIAN_POINT('',(30.2,43.0755441166495,40.321625226856)) ;
#15825=CARTESIAN_POINT('',(30.2,43.3462024860906,40.518656404528)) ;
#15826=CARTESIAN_POINT('',(29.6,43.0755441166495,40.321625226856)) ;
#15827=CARTESIAN_POINT('Origin',(30.2,43.1628233407496,40.2629278588902)) ;
#15828=CARTESIAN_POINT('',(30.2,43.1008833801193,40.1779191226171)) ;
#15829=CARTESIAN_POINT('Origin',(30.2,39.642135623731,39.642135623731)) ;
#15830=CARTESIAN_POINT('',(30.2,42.9412415963219,40.2238570189152)) ;
#15831=CARTESIAN_POINT('Origin',(33.6,43.4226076842641,40.0853409932026)) ;
#15832=CARTESIAN_POINT('',(33.2,43.1008833801193,40.1779191226171)) ;
#15833=CARTESIAN_POINT('Ctrl Pts',(33.2,43.1008833801193,40.1779191226171)) ;
#15834=CARTESIAN_POINT('Ctrl Pts',(33.2770142911999,43.0193145854792,40.2013910404334)) ;
#15835=CARTESIAN_POINT('Ctrl Pts',(33.35,42.9412415963219,40.2238570189152)) ;
#15836=CARTESIAN_POINT('',(29.6,43.1008833801193,40.1779191226171)) ;
#15837=CARTESIAN_POINT('Origin',(29.6,39.642135623731,39.642135623731)) ;
#15838=CARTESIAN_POINT('',(33.2,43.1413750581413,39.7150971249983)) ;
#15839=CARTESIAN_POINT('Origin',(33.2,39.642135623731,39.642135623731)) ;
#15840=CARTESIAN_POINT('',(30.2,43.1413750581413,39.7150971249983)) ;
#15841=CARTESIAN_POINT('',(29.6,43.1413750581413,39.7150971249983)) ;
#15842=CARTESIAN_POINT('',(30.2,43.1413750581413,39.5691741224636)) ;
#15843=CARTESIAN_POINT('Origin',(30.2,39.642135623731,39.642135623731)) ;
#15844=CARTESIAN_POINT('',(33.2,43.1413750581413,39.5691741224636)) ;
#15845=CARTESIAN_POINT('',(29.6,43.1413750581413,39.5691741224636)) ;
#15846=CARTESIAN_POINT('',(33.2,43.1008833801193,39.1063521248448)) ;
#15847=CARTESIAN_POINT('Origin',(33.2,39.642135623731,39.642135623731)) ;
#15848=CARTESIAN_POINT('',(30.2,43.1008833801193,39.1063521248448)) ;
#15849=CARTESIAN_POINT('',(29.6,43.1008833801193,39.1063521248448)) ;
#15850=CARTESIAN_POINT('',(30.2,43.0755441166495,38.9626460206059)) ;
#15851=CARTESIAN_POINT('Origin',(30.2,39.642135623731,39.642135623731)) ;
#15852=CARTESIAN_POINT('',(33.2,43.0755441166495,38.9626460206059)) ;
#15853=CARTESIAN_POINT('',(29.6,43.0755441166495,38.9626460206059)) ;
#15854=CARTESIAN_POINT('',(33.2,42.9552994017302,38.5138866351854)) ;
#15855=CARTESIAN_POINT('Origin',(33.2,39.642135623731,39.642135623731)) ;
#15856=CARTESIAN_POINT('',(30.2,42.9552994017302,38.5138866351854)) ;
#15857=CARTESIAN_POINT('',(29.6,42.9552994017302,38.5138866351854)) ;
#15858=CARTESIAN_POINT('',(30.2,42.9053907954888,38.3767638665007)) ;
#15859=CARTESIAN_POINT('Origin',(30.2,39.642135623731,39.642135623731)) ;
#15860=CARTESIAN_POINT('',(33.2,42.9053907954888,38.3767638665007)) ;
#15861=CARTESIAN_POINT('',(29.6,42.9053907954888,38.3767638665007)) ;
#15862=CARTESIAN_POINT('',(33.2,42.7090466184883,37.9557024201215)) ;
#15863=CARTESIAN_POINT('Origin',(33.2,39.642135623731,39.642135623731)) ;
#15864=CARTESIAN_POINT('',(30.2,42.7090466184883,37.9557024201215)) ;
#15865=CARTESIAN_POINT('',(29.6,42.7090466184883,37.9557024201215)) ;
#15866=CARTESIAN_POINT('',(30.2,42.636085117221,37.82932939293)) ;
#15867=CARTESIAN_POINT('Origin',(30.2,39.642135623731,39.642135623731)) ;
#15868=CARTESIAN_POINT('',(33.2,42.636085117221,37.82932939293)) ;
#15869=CARTESIAN_POINT('',(29.6,42.636085117221,37.82932939293)) ;
#15870=CARTESIAN_POINT('',(33.2,42.3696072966026,37.4487596245729)) ;
#15871=CARTESIAN_POINT('Origin',(33.2,39.642135623731,39.642135623731)) ;
#15872=CARTESIAN_POINT('',(30.2,42.3696072966026,37.4487596245729)) ;
#15873=CARTESIAN_POINT('',(29.6,42.3696072966026,37.4487596245729)) ;
#15874=CARTESIAN_POINT('',(30.2,42.2758097986051,37.336976119358)) ;
#15875=CARTESIAN_POINT('Origin',(30.2,39.642135623731,39.642135623731)) ;
#15876=CARTESIAN_POINT('',(33.2,42.2758097986051,37.336976119358)) ;
#15877=CARTESIAN_POINT('',(29.6,42.2758097986051,37.336976119358)) ;
#15878=CARTESIAN_POINT('',(33.2,41.9472951281039,37.0084614488568)) ;
#15879=CARTESIAN_POINT('Origin',(33.2,39.642135623731,39.642135623731)) ;
#15880=CARTESIAN_POINT('',(30.2,41.9472951281039,37.0084614488568)) ;
#15881=CARTESIAN_POINT('',(29.6,41.9472951281039,37.0084614488568)) ;
#15882=CARTESIAN_POINT('',(30.2,41.835511622889,36.9146639508593)) ;
#15883=CARTESIAN_POINT('Origin',(30.2,39.642135623731,39.642135623731)) ;
#15884=CARTESIAN_POINT('',(33.2,41.835511622889,36.9146639508593)) ;
#15885=CARTESIAN_POINT('',(29.6,41.835511622889,36.9146639508593)) ;
#15886=CARTESIAN_POINT('',(33.2,41.4549418545319,36.6481861302409)) ;
#15887=CARTESIAN_POINT('Origin',(33.2,39.642135623731,39.642135623731)) ;
#15888=CARTESIAN_POINT('',(30.2,41.4549418545319,36.6481861302409)) ;
#15889=CARTESIAN_POINT('',(29.6,41.4549418545319,36.6481861302409)) ;
#15890=CARTESIAN_POINT('',(30.2,41.3285688273404,36.5752246289736)) ;
#15891=CARTESIAN_POINT('Origin',(30.2,39.642135623731,39.642135623731)) ;
#15892=CARTESIAN_POINT('',(33.2,41.3285688273404,36.5752246289736)) ;
#15893=CARTESIAN_POINT('',(29.6,41.3285688273404,36.5752246289736)) ;
#15894=CARTESIAN_POINT('',(33.2,40.9075073809612,36.3788804519731)) ;
#15895=CARTESIAN_POINT('Origin',(33.2,39.642135623731,39.642135623731)) ;
#15896=CARTESIAN_POINT('',(30.2,40.9075073809612,36.3788804519732)) ;
#15897=CARTESIAN_POINT('',(29.6,40.9075073809612,36.3788804519731)) ;
#15898=CARTESIAN_POINT('',(30.2,40.7703846122765,36.3289718457317)) ;
#15899=CARTESIAN_POINT('Origin',(30.2,39.642135623731,39.642135623731)) ;
#15900=CARTESIAN_POINT('',(33.2,40.7703846122765,36.3289718457317)) ;
#15901=CARTESIAN_POINT('',(29.6,40.7703846122765,36.3289718457317)) ;
#15902=CARTESIAN_POINT('',(33.2,40.321625226856,36.2087271308124)) ;
#15903=CARTESIAN_POINT('Origin',(33.2,39.642135623731,39.642135623731)) ;
#15904=CARTESIAN_POINT('',(30.2,40.321625226856,36.2087271308124)) ;
#15905=CARTESIAN_POINT('',(29.6,40.321625226856,36.2087271308124)) ;
#15906=CARTESIAN_POINT('',(30.2,40.1779191226171,36.1833878673426)) ;
#15907=CARTESIAN_POINT('Origin',(30.2,39.642135623731,39.642135623731)) ;
#15908=CARTESIAN_POINT('',(33.2,40.1779191226171,36.1833878673426)) ;
#15909=CARTESIAN_POINT('',(29.6,40.1779191226171,36.1833878673426)) ;
#15910=CARTESIAN_POINT('',(33.2,39.7150971249983,36.1428961893205)) ;
#15911=CARTESIAN_POINT('Origin',(33.2,39.642135623731,39.642135623731)) ;
#15912=CARTESIAN_POINT('',(30.2,39.7150971249983,36.1428961893206)) ;
#15913=CARTESIAN_POINT('',(29.6,39.7150971249983,36.1428961893205)) ;
#15914=CARTESIAN_POINT('',(30.2,39.5691741224637,36.1428961893205)) ;
#15915=CARTESIAN_POINT('Origin',(30.2,39.642135623731,39.642135623731)) ;
#15916=CARTESIAN_POINT('',(33.2,39.5691741224636,36.1428961893205)) ;
#15917=CARTESIAN_POINT('',(29.6,39.5691741224636,36.1428961893205)) ;
#15918=CARTESIAN_POINT('',(33.2,39.1063521248448,36.1833878673426)) ;
#15919=CARTESIAN_POINT('Origin',(33.2,39.642135623731,39.642135623731)) ;
#15920=CARTESIAN_POINT('',(30.2,39.1063521248448,36.1833878673426)) ;
#15921=CARTESIAN_POINT('',(29.6,39.1063521248448,36.1833878673426)) ;
#15922=CARTESIAN_POINT('',(30.2,38.9626460206059,36.2087271308124)) ;
#15923=CARTESIAN_POINT('Origin',(30.2,39.642135623731,39.642135623731)) ;
#15924=CARTESIAN_POINT('',(33.2,38.9626460206059,36.2087271308124)) ;
#15925=CARTESIAN_POINT('',(29.6,38.9626460206059,36.2087271308124)) ;
#15926=CARTESIAN_POINT('',(33.2,38.5138866351854,36.3289718457317)) ;
#15927=CARTESIAN_POINT('Origin',(33.2,39.642135623731,39.642135623731)) ;
#15928=CARTESIAN_POINT('',(30.2,38.5138866351854,36.3289718457317)) ;
#15929=CARTESIAN_POINT('',(29.6,38.5138866351854,36.3289718457317)) ;
#15930=CARTESIAN_POINT('',(30.2,38.3767638665007,36.3788804519731)) ;
#15931=CARTESIAN_POINT('Origin',(30.2,39.642135623731,39.642135623731)) ;
#15932=CARTESIAN_POINT('',(33.2,38.3767638665007,36.3788804519731)) ;
#15933=CARTESIAN_POINT('',(29.6,38.3767638665007,36.3788804519731)) ;
#15934=CARTESIAN_POINT('',(33.2,37.9557024201215,36.5752246289736)) ;
#15935=CARTESIAN_POINT('Origin',(33.2,39.642135623731,39.642135623731)) ;
#15936=CARTESIAN_POINT('',(30.2,37.9557024201215,36.5752246289736)) ;
#15937=CARTESIAN_POINT('',(29.6,37.9557024201215,36.5752246289736)) ;
#15938=CARTESIAN_POINT('',(30.2,37.82932939293,36.6481861302409)) ;
#15939=CARTESIAN_POINT('Origin',(30.2,39.642135623731,39.642135623731)) ;
#15940=CARTESIAN_POINT('',(33.2,37.82932939293,36.6481861302409)) ;
#15941=CARTESIAN_POINT('',(29.6,37.82932939293,36.6481861302409)) ;
#15942=CARTESIAN_POINT('',(33.2,37.4487596245729,36.9146639508593)) ;
#15943=CARTESIAN_POINT('Origin',(33.2,39.642135623731,39.642135623731)) ;
#15944=CARTESIAN_POINT('',(30.2,37.4487596245729,36.9146639508593)) ;
#15945=CARTESIAN_POINT('',(29.6,37.4487596245729,36.9146639508593)) ;
#15946=CARTESIAN_POINT('',(30.2,37.336976119358,37.0084614488568)) ;
#15947=CARTESIAN_POINT('Origin',(30.2,39.642135623731,39.642135623731)) ;
#15948=CARTESIAN_POINT('',(33.2,37.336976119358,37.0084614488568)) ;
#15949=CARTESIAN_POINT('',(29.6,37.336976119358,37.0084614488568)) ;
#15950=CARTESIAN_POINT('',(33.2,37.0084614488568,37.336976119358)) ;
#15951=CARTESIAN_POINT('Origin',(33.2,39.642135623731,39.642135623731)) ;
#15952=CARTESIAN_POINT('',(30.2,37.0084614488568,37.336976119358)) ;
#15953=CARTESIAN_POINT('',(29.6,37.0084614488568,37.336976119358)) ;
#15954=CARTESIAN_POINT('',(30.2,36.9146639508593,37.4487596245729)) ;
#15955=CARTESIAN_POINT('Origin',(30.2,39.642135623731,39.642135623731)) ;
#15956=CARTESIAN_POINT('',(33.2,36.9146639508593,37.4487596245729)) ;
#15957=CARTESIAN_POINT('',(29.6,36.9146639508593,37.4487596245729)) ;
#15958=CARTESIAN_POINT('',(33.2,36.6481861302409,37.82932939293)) ;
#15959=CARTESIAN_POINT('Origin',(33.2,39.642135623731,39.642135623731)) ;
#15960=CARTESIAN_POINT('',(30.2,36.6481861302409,37.82932939293)) ;
#15961=CARTESIAN_POINT('',(29.6,36.6481861302409,37.82932939293)) ;
#15962=CARTESIAN_POINT('',(30.2,36.5752246289736,37.9557024201215)) ;
#15963=CARTESIAN_POINT('Origin',(30.2,39.642135623731,39.642135623731)) ;
#15964=CARTESIAN_POINT('',(33.2,36.5752246289736,37.9557024201215)) ;
#15965=CARTESIAN_POINT('',(29.6,36.5752246289736,37.9557024201215)) ;
#15966=CARTESIAN_POINT('',(33.2,36.3788804519731,38.3767638665007)) ;
#15967=CARTESIAN_POINT('Origin',(33.2,39.642135623731,39.642135623731)) ;
#15968=CARTESIAN_POINT('',(30.2,36.3788804519731,38.3767638665007)) ;
#15969=CARTESIAN_POINT('',(29.6,36.3788804519731,38.3767638665007)) ;
#15970=CARTESIAN_POINT('',(30.2,36.3289718457317,38.5138866351854)) ;
#15971=CARTESIAN_POINT('Origin',(30.2,39.642135623731,39.642135623731)) ;
#15972=CARTESIAN_POINT('',(33.2,36.3289718457317,38.5138866351854)) ;
#15973=CARTESIAN_POINT('',(29.6,36.3289718457317,38.5138866351854)) ;
#15974=CARTESIAN_POINT('',(33.2,36.2087271308124,38.9626460206059)) ;
#15975=CARTESIAN_POINT('Origin',(33.2,39.642135623731,39.642135623731)) ;
#15976=CARTESIAN_POINT('',(30.2,36.2087271308124,38.9626460206059)) ;
#15977=CARTESIAN_POINT('',(29.6,36.2087271308124,38.9626460206059)) ;
#15978=CARTESIAN_POINT('',(30.2,36.1833878673426,39.1063521248448)) ;
#15979=CARTESIAN_POINT('Origin',(30.2,39.642135623731,39.642135623731)) ;
#15980=CARTESIAN_POINT('',(33.2,36.1833878673426,39.1063521248448)) ;
#15981=CARTESIAN_POINT('',(29.6,36.1833878673426,39.1063521248448)) ;
#15982=CARTESIAN_POINT('',(33.2,36.1428961893205,39.5691741224636)) ;
#15983=CARTESIAN_POINT('Origin',(33.2,39.642135623731,39.642135623731)) ;
#15984=CARTESIAN_POINT('',(30.2,36.1428961893205,39.5691741224636)) ;
#15985=CARTESIAN_POINT('',(29.6,36.1428961893205,39.5691741224636)) ;
#15986=CARTESIAN_POINT('',(30.2,36.1428961893206,39.7150971249983)) ;
#15987=CARTESIAN_POINT('Origin',(30.2,39.642135623731,39.642135623731)) ;
#15988=CARTESIAN_POINT('',(33.2,36.1428961893206,39.7150971249983)) ;
#15989=CARTESIAN_POINT('',(29.6,36.1428961893206,39.7150971249983)) ;
#15990=CARTESIAN_POINT('',(33.2,36.1833878673426,40.1779191226171)) ;
#15991=CARTESIAN_POINT('Origin',(33.2,39.642135623731,39.642135623731)) ;
#15992=CARTESIAN_POINT('',(30.2,36.1833878673426,40.1779191226171)) ;
#15993=CARTESIAN_POINT('',(29.6,36.1833878673426,40.1779191226171)) ;
#15994=CARTESIAN_POINT('',(30.2,36.2087271308124,40.321625226856)) ;
#15995=CARTESIAN_POINT('Origin',(30.2,39.642135623731,39.642135623731)) ;
#15996=CARTESIAN_POINT('',(33.2,36.2087271308124,40.321625226856)) ;
#15997=CARTESIAN_POINT('',(29.6,36.2087271308124,40.321625226856)) ;
#15998=CARTESIAN_POINT('',(33.2,36.3289718457317,40.7703846122765)) ;
#15999=CARTESIAN_POINT('Origin',(33.2,39.642135623731,39.642135623731)) ;
#16000=CARTESIAN_POINT('',(30.2,36.3289718457317,40.7703846122765)) ;
#16001=CARTESIAN_POINT('',(29.6,36.3289718457317,40.7703846122765)) ;
#16002=CARTESIAN_POINT('',(30.2,36.3788804519731,40.9075073809612)) ;
#16003=CARTESIAN_POINT('Origin',(30.2,39.642135623731,39.642135623731)) ;
#16004=CARTESIAN_POINT('',(33.2,36.3788804519731,40.9075073809612)) ;
#16005=CARTESIAN_POINT('',(29.6,36.3788804519731,40.9075073809612)) ;
#16006=CARTESIAN_POINT('',(33.2,36.5752246289736,41.3285688273404)) ;
#16007=CARTESIAN_POINT('Origin',(33.2,39.642135623731,39.642135623731)) ;
#16008=CARTESIAN_POINT('',(30.2,36.5752246289736,41.3285688273404)) ;
#16009=CARTESIAN_POINT('',(29.6,36.5752246289736,41.3285688273404)) ;
#16010=CARTESIAN_POINT('',(30.2,36.6481861302409,41.4549418545319)) ;
#16011=CARTESIAN_POINT('Origin',(30.2,39.642135623731,39.642135623731)) ;
#16012=CARTESIAN_POINT('',(33.2,36.6481861302409,41.4549418545319)) ;
#16013=CARTESIAN_POINT('',(29.6,36.6481861302409,41.4549418545319)) ;
#16014=CARTESIAN_POINT('',(33.2,36.9146639508593,41.835511622889)) ;
#16015=CARTESIAN_POINT('Origin',(33.2,39.642135623731,39.642135623731)) ;
#16016=CARTESIAN_POINT('',(30.2,36.9146639508593,41.835511622889)) ;
#16017=CARTESIAN_POINT('',(29.6,36.9146639508593,41.835511622889)) ;
#16018=CARTESIAN_POINT('',(30.2,37.0084614488568,41.9472951281039)) ;
#16019=CARTESIAN_POINT('Origin',(30.2,39.642135623731,39.642135623731)) ;
#16020=CARTESIAN_POINT('',(33.2,37.0084614488568,41.9472951281039)) ;
#16021=CARTESIAN_POINT('',(29.6,37.0084614488568,41.9472951281039)) ;
#16022=CARTESIAN_POINT('',(33.2,37.336976119358,42.2758097986051)) ;
#16023=CARTESIAN_POINT('Origin',(33.2,39.642135623731,39.642135623731)) ;
#16024=CARTESIAN_POINT('',(30.2,37.336976119358,42.2758097986051)) ;
#16025=CARTESIAN_POINT('',(29.6,37.336976119358,42.2758097986051)) ;
#16026=CARTESIAN_POINT('',(30.2,37.4487596245729,42.3696072966026)) ;
#16027=CARTESIAN_POINT('Origin',(30.2,39.642135623731,39.642135623731)) ;
#16028=CARTESIAN_POINT('',(33.2,37.4487596245729,42.3696072966026)) ;
#16029=CARTESIAN_POINT('',(29.6,37.4487596245729,42.3696072966026)) ;
#16030=CARTESIAN_POINT('',(33.2,37.82932939293,42.636085117221)) ;
#16031=CARTESIAN_POINT('Origin',(33.2,39.642135623731,39.642135623731)) ;
#16032=CARTESIAN_POINT('',(30.2,37.82932939293,42.636085117221)) ;
#16033=CARTESIAN_POINT('',(29.6,37.82932939293,42.636085117221)) ;
#16034=CARTESIAN_POINT('',(30.2,37.9557024201215,42.7090466184883)) ;
#16035=CARTESIAN_POINT('Origin',(30.2,39.642135623731,39.642135623731)) ;
#16036=CARTESIAN_POINT('',(33.2,37.9557024201215,42.7090466184883)) ;
#16037=CARTESIAN_POINT('',(29.6,37.9557024201215,42.7090466184883)) ;
#16038=CARTESIAN_POINT('',(33.2,38.3767638665007,42.9053907954887)) ;
#16039=CARTESIAN_POINT('Origin',(33.2,39.642135623731,39.642135623731)) ;
#16040=CARTESIAN_POINT('',(30.2,38.3767638665007,42.9053907954887)) ;
#16041=CARTESIAN_POINT('',(29.6,38.3767638665007,42.9053907954887)) ;
#16042=CARTESIAN_POINT('',(30.2,38.5138866351854,42.9552994017302)) ;
#16043=CARTESIAN_POINT('Origin',(30.2,39.642135623731,39.642135623731)) ;
#16044=CARTESIAN_POINT('',(33.2,38.5138866351854,42.9552994017302)) ;
#16045=CARTESIAN_POINT('',(29.6,38.5138866351854,42.9552994017302)) ;
#16046=CARTESIAN_POINT('',(33.2,38.9626460206059,43.0755441166495)) ;
#16047=CARTESIAN_POINT('Origin',(33.2,39.642135623731,39.642135623731)) ;
#16048=CARTESIAN_POINT('',(30.2,38.9626460206059,43.0755441166495)) ;
#16049=CARTESIAN_POINT('',(29.6,38.9626460206059,43.0755441166495)) ;
#16050=CARTESIAN_POINT('',(30.2,39.1063521248448,43.1008833801193)) ;
#16051=CARTESIAN_POINT('Origin',(30.2,39.642135623731,39.642135623731)) ;
#16052=CARTESIAN_POINT('',(33.2,39.1063521248448,43.1008833801193)) ;
#16053=CARTESIAN_POINT('',(29.6,39.1063521248448,43.1008833801193)) ;
#16054=CARTESIAN_POINT('',(33.2,39.5691741224636,43.1413750581413)) ;
#16055=CARTESIAN_POINT('Origin',(33.2,39.642135623731,39.642135623731)) ;
#16056=CARTESIAN_POINT('',(30.2,39.5691741224636,43.1413750581413)) ;
#16057=CARTESIAN_POINT('',(29.6,39.5691741224636,43.1413750581413)) ;
#16058=CARTESIAN_POINT('',(30.2,39.642135623731,43.142135623731)) ;
#16059=CARTESIAN_POINT('Origin',(30.2,39.642135623731,39.642135623731)) ;
#16060=CARTESIAN_POINT('',(29.8,39.642135623731,43.142135623731)) ;
#16061=CARTESIAN_POINT('',(29.6,39.642135623731,43.142135623731)) ;
#16062=CARTESIAN_POINT('Origin',(29.8,39.642135623731,39.642135623731)) ;
#16063=CARTESIAN_POINT('',(30.2,39.7150971249983,43.1413750581413)) ;
#16064=CARTESIAN_POINT('Origin',(30.2,39.642135623731,39.642135623731)) ;
#16065=CARTESIAN_POINT('',(33.2,39.7150971249983,43.1413750581414)) ;
#16066=CARTESIAN_POINT('',(29.6,39.7150971249983,43.1413750581414)) ;
#16067=CARTESIAN_POINT('',(33.2,40.1779191226171,43.1008833801193)) ;
#16068=CARTESIAN_POINT('Origin',(33.2,39.642135623731,39.642135623731)) ;
#16069=CARTESIAN_POINT('',(30.2,40.1779191226171,43.1008833801193)) ;
#16070=CARTESIAN_POINT('',(29.6,40.1779191226171,43.1008833801193)) ;
#16071=CARTESIAN_POINT('',(30.2,40.321625226856,43.0755441166495)) ;
#16072=CARTESIAN_POINT('Origin',(30.2,39.642135623731,39.642135623731)) ;
#16073=CARTESIAN_POINT('',(33.2,40.321625226856,43.0755441166495)) ;
#16074=CARTESIAN_POINT('',(29.6,40.321625226856,43.0755441166495)) ;
#16075=CARTESIAN_POINT('',(33.2,40.7703846122765,42.9552994017302)) ;
#16076=CARTESIAN_POINT('Origin',(33.2,39.642135623731,39.642135623731)) ;
#16077=CARTESIAN_POINT('',(30.2,40.7703846122765,42.9552994017302)) ;
#16078=CARTESIAN_POINT('',(29.6,40.7703846122765,42.9552994017302)) ;
#16079=CARTESIAN_POINT('',(30.2,40.9075073809612,42.9053907954888)) ;
#16080=CARTESIAN_POINT('Origin',(30.2,39.642135623731,39.642135623731)) ;
#16081=CARTESIAN_POINT('',(33.2,40.9075073809612,42.9053907954888)) ;
#16082=CARTESIAN_POINT('',(29.6,40.9075073809612,42.9053907954888)) ;
#16083=CARTESIAN_POINT('',(33.2,41.3285688273404,42.7090466184883)) ;
#16084=CARTESIAN_POINT('Origin',(33.2,39.642135623731,39.642135623731)) ;
#16085=CARTESIAN_POINT('',(30.2,41.3285688273404,42.7090466184883)) ;
#16086=CARTESIAN_POINT('',(29.6,41.3285688273404,42.7090466184883)) ;
#16087=CARTESIAN_POINT('',(30.2,41.4549418545319,42.636085117221)) ;
#16088=CARTESIAN_POINT('Origin',(30.2,39.642135623731,39.642135623731)) ;
#16089=CARTESIAN_POINT('',(33.2,41.4549418545319,42.636085117221)) ;
#16090=CARTESIAN_POINT('',(29.6,41.4549418545319,42.636085117221)) ;
#16091=CARTESIAN_POINT('',(33.2,41.8355116228891,42.3696072966026)) ;
#16092=CARTESIAN_POINT('Origin',(33.2,39.642135623731,39.642135623731)) ;
#16093=CARTESIAN_POINT('',(30.2,41.835511622889,42.3696072966026)) ;
#16094=CARTESIAN_POINT('',(29.6,41.8355116228891,42.3696072966026)) ;
#16095=CARTESIAN_POINT('',(30.2,41.9472951281039,42.2758097986051)) ;
#16096=CARTESIAN_POINT('Origin',(30.2,39.642135623731,39.642135623731)) ;
#16097=CARTESIAN_POINT('',(33.2,41.9472951281039,42.2758097986051)) ;
#16098=CARTESIAN_POINT('',(29.6,41.9472951281039,42.2758097986051)) ;
#16099=CARTESIAN_POINT('',(33.2,42.2758097986051,41.9472951281039)) ;
#16100=CARTESIAN_POINT('Origin',(33.2,39.642135623731,39.642135623731)) ;
#16101=CARTESIAN_POINT('',(30.2,42.2758097986051,41.9472951281039)) ;
#16102=CARTESIAN_POINT('',(29.6,42.2758097986051,41.9472951281039)) ;
#16103=CARTESIAN_POINT('',(30.2,42.3696072966026,41.835511622889)) ;
#16104=CARTESIAN_POINT('Origin',(30.2,39.642135623731,39.642135623731)) ;
#16105=CARTESIAN_POINT('',(33.2,42.3696072966026,41.835511622889)) ;
#16106=CARTESIAN_POINT('',(29.6,42.3696072966026,41.835511622889)) ;
#16107=CARTESIAN_POINT('',(33.2,42.636085117221,41.4549418545319)) ;
#16108=CARTESIAN_POINT('Origin',(33.2,39.642135623731,39.642135623731)) ;
#16109=CARTESIAN_POINT('',(30.2,42.636085117221,41.4549418545319)) ;
#16110=CARTESIAN_POINT('',(29.6,42.636085117221,41.4549418545319)) ;
#16111=CARTESIAN_POINT('',(30.2,42.7090466184883,41.3285688273404)) ;
#16112=CARTESIAN_POINT('Origin',(30.2,39.642135623731,39.642135623731)) ;
#16113=CARTESIAN_POINT('',(33.2,42.7090466184883,41.3285688273404)) ;
#16114=CARTESIAN_POINT('',(29.6,42.7090466184883,41.3285688273404)) ;
#16115=CARTESIAN_POINT('',(33.2,42.9053907954888,40.9075073809612)) ;
#16116=CARTESIAN_POINT('Origin',(33.2,39.642135623731,39.642135623731)) ;
#16117=CARTESIAN_POINT('',(30.2,42.9053907954888,40.9075073809612)) ;
#16118=CARTESIAN_POINT('',(29.6,42.9053907954888,40.9075073809612)) ;
#16119=CARTESIAN_POINT('',(30.2,42.9552994017302,40.7703846122765)) ;
#16120=CARTESIAN_POINT('Origin',(30.2,39.642135623731,39.642135623731)) ;
#16121=CARTESIAN_POINT('',(33.2,42.9552994017302,40.7703846122765)) ;
#16122=CARTESIAN_POINT('',(29.6,42.9552994017302,40.7703846122765)) ;
#16123=CARTESIAN_POINT('Origin',(33.2,39.642135623731,39.642135623731)) ;
#16124=CARTESIAN_POINT('Origin',(33.6,42.7901059033638,40.7879031038719)) ;
#16125=CARTESIAN_POINT('',(33.35,42.7901059033638,40.7879031038719)) ;
#16126=CARTESIAN_POINT('Ctrl Pts',(33.35,42.7901059033638,40.7879031038719)) ;
#16127=CARTESIAN_POINT('Ctrl Pts',(33.2770142912003,42.8464861060822,40.8463957065364)) ;
#16128=CARTESIAN_POINT('Ctrl Pts',(33.2,42.9053907954888,40.9075073809612)) ;
#16129=CARTESIAN_POINT('',(30.2,42.7901059033638,40.7879031038719)) ;
#16130=CARTESIAN_POINT('',(33.6,42.7901059033638,40.7879031038719)) ;
#16131=CARTESIAN_POINT('',(30.2,43.1377231511858,41.1485445449414)) ;
#16132=CARTESIAN_POINT('Origin',(30.2,43.0015367430406,40.8648576361202)) ;
#16133=CARTESIAN_POINT('',(30.2,42.7901059033638,40.7879031038719)) ;
#16134=CARTESIAN_POINT('Origin',(33.6,43.288212014249,40.7350797917956)) ;
#16135=CARTESIAN_POINT('Ctrl Pts',(33.2,42.9552994017302,40.7703846122765)) ;
#16136=CARTESIAN_POINT('Ctrl Pts',(33.2770142912003,42.8708939646091,40.7793356663763)) ;
#16137=CARTESIAN_POINT('Ctrl Pts',(33.35,42.7901059033638,40.7879031038719)) ;
#16138=CARTESIAN_POINT('Origin',(33.6,42.5433207264088,41.3171356237309)) ;
#16139=CARTESIAN_POINT('',(33.35,42.5433207264088,41.3171356237309)) ;
#16140=CARTESIAN_POINT('Ctrl Pts',(33.35,42.5433207264088,41.3171356237309)) ;
#16141=CARTESIAN_POINT('Ctrl Pts',(33.2770142912008,42.5886872533023,41.3845299117868)) ;
#16142=CARTESIAN_POINT('Ctrl Pts',(33.2,42.636085117221,41.4549418545319)) ;
#16143=CARTESIAN_POINT('',(30.2,42.5433207264088,41.3171356237309)) ;
#16144=CARTESIAN_POINT('',(33.6,42.5433207264088,41.3171356237309)) ;
#16145=CARTESIAN_POINT('',(30.2,42.8230321581118,41.7326612125635)) ;
#16146=CARTESIAN_POINT('Origin',(30.2,42.7381764422603,41.429635623731)) ;
#16147=CARTESIAN_POINT('',(30.2,42.5433207264088,41.3171356237309)) ;
#16148=CARTESIAN_POINT('Origin',(33.6,43.0430321581118,41.3516100348984)) ;
#16149=CARTESIAN_POINT('Ctrl Pts',(33.2,42.7090466184883,41.3285688273404)) ;
#16150=CARTESIAN_POINT('Ctrl Pts',(33.2770142912,42.6243691553829,41.3227270444743)) ;
#16151=CARTESIAN_POINT('Ctrl Pts',(33.35,42.5433207264088,41.3171356237309)) ;
#16152=CARTESIAN_POINT('Origin',(33.6,42.2083845081795,41.7954741161808)) ;
#16153=CARTESIAN_POINT('',(33.35,42.2083845081795,41.7954741161808)) ;
#16154=CARTESIAN_POINT('Ctrl Pts',(33.35,42.2083845081795,41.7954741161808)) ;
#16155=CARTESIAN_POINT('Ctrl Pts',(33.2770142912003,42.2413589202856,41.8697223482896)) ;
#16156=CARTESIAN_POINT('Ctrl Pts',(33.2,42.2758097986051,41.9472951281039)) ;
#16157=CARTESIAN_POINT('',(30.2,42.2083845081795,41.7954741161808)) ;
#16158=CARTESIAN_POINT('',(33.6,42.2083845081795,41.7954741161808)) ;
#16159=CARTESIAN_POINT('',(30.2,42.411691233452,42.253258318026)) ;
#16160=CARTESIAN_POINT('Origin',(30.2,42.3807445078813,41.9401013283603)) ;
#16161=CARTESIAN_POINT('',(30.2,42.2083845081795,41.7954741161808)) ;
#16162=CARTESIAN_POINT('Origin',(33.6,42.6945177817141,41.9161987630536)) ;
#16163=CARTESIAN_POINT('Ctrl Pts',(33.2,42.3696072966026,41.8355116228891)) ;
#16164=CARTESIAN_POINT('Ctrl Pts',(33.2770142912001,42.2872306893798,41.8150545026733)) ;
#16165=CARTESIAN_POINT('Ctrl Pts',(33.35,42.2083845081795,41.7954741161808)) ;
#16166=CARTESIAN_POINT('Origin',(33.6,41.7954741161809,42.2083845081795)) ;
#16167=CARTESIAN_POINT('',(33.35,41.7954741161809,42.2083845081795)) ;
#16168=CARTESIAN_POINT('Ctrl Pts',(33.35,41.7954741161809,42.2083845081795)) ;
#16169=CARTESIAN_POINT('Ctrl Pts',(33.2770142912002,41.8150545026733,42.2872306893797)) ;
#16170=CARTESIAN_POINT('Ctrl Pts',(33.2,41.8355116228891,42.3696072966026)) ;
#16171=CARTESIAN_POINT('',(30.2,41.7954741161809,42.2083845081795)) ;
#16172=CARTESIAN_POINT('',(33.6,41.7954741161809,42.2083845081795)) ;
#16173=CARTESIAN_POINT('',(30.2,41.9161987630536,42.6945177817141)) ;
#16174=CARTESIAN_POINT('Origin',(30.2,41.9401013283603,42.3807445078813)) ;
#16175=CARTESIAN_POINT('',(30.2,41.7954741161809,42.2083845081795)) ;
#16176=CARTESIAN_POINT('Origin',(33.6,42.253258318026,42.411691233452)) ;
#16177=CARTESIAN_POINT('Ctrl Pts',(33.2,41.9472951281039,42.2758097986051)) ;
#16178=CARTESIAN_POINT('Ctrl Pts',(33.2770142912005,41.8697223482895,42.2413589202856)) ;
#16179=CARTESIAN_POINT('Ctrl Pts',(33.35,41.7954741161809,42.2083845081795)) ;
#16180=CARTESIAN_POINT('Origin',(33.6,41.3171356237309,42.5433207264088)) ;
#16181=CARTESIAN_POINT('',(33.35,41.3171356237309,42.5433207264088)) ;
#16182=CARTESIAN_POINT('Ctrl Pts',(33.35,41.3171356237309,42.5433207264088)) ;
#16183=CARTESIAN_POINT('Ctrl Pts',(33.2770142912002,41.3227270444743,42.6243691553827)) ;
#16184=CARTESIAN_POINT('Ctrl Pts',(33.2,41.3285688273404,42.7090466184883)) ;
#16185=CARTESIAN_POINT('',(30.2,41.3171356237309,42.5433207264088)) ;
#16186=CARTESIAN_POINT('',(33.6,41.3171356237309,42.5433207264088)) ;
#16187=CARTESIAN_POINT('',(30.2,41.3516100348984,43.0430321581118)) ;
#16188=CARTESIAN_POINT('Origin',(30.2,41.429635623731,42.7381764422603)) ;
#16189=CARTESIAN_POINT('',(30.2,41.3171356237309,42.5433207264088)) ;
#16190=CARTESIAN_POINT('Origin',(33.6,41.7326612125635,42.8230321581118)) ;
#16191=CARTESIAN_POINT('Ctrl Pts',(33.2,41.4549418545319,42.636085117221)) ;
#16192=CARTESIAN_POINT('Ctrl Pts',(33.2770142912003,41.3845299117873,42.5886872533027)) ;
#16193=CARTESIAN_POINT('Ctrl Pts',(33.35,41.3171356237309,42.5433207264088)) ;
#16194=CARTESIAN_POINT('Origin',(33.6,40.7879031038719,42.7901059033638)) ;
#16195=CARTESIAN_POINT('',(33.35,40.7879031038719,42.7901059033638)) ;
#16196=CARTESIAN_POINT('Ctrl Pts',(33.35,40.7879031038719,42.7901059033638)) ;
#16197=CARTESIAN_POINT('Ctrl Pts',(33.2770142912004,40.7793356663763,42.8708939646091)) ;
#16198=CARTESIAN_POINT('Ctrl Pts',(33.2,40.7703846122765,42.9552994017302)) ;
#16199=CARTESIAN_POINT('',(30.2,40.7879031038719,42.7901059033638)) ;
#16200=CARTESIAN_POINT('',(33.6,40.7879031038719,42.7901059033638)) ;
#16201=CARTESIAN_POINT('',(30.2,40.7350797917956,43.288212014249)) ;
#16202=CARTESIAN_POINT('Origin',(30.2,40.8648576361202,43.0015367430406)) ;
#16203=CARTESIAN_POINT('',(30.2,40.7879031038719,42.7901059033638)) ;
#16204=CARTESIAN_POINT('Origin',(33.6,41.1485445449414,43.1377231511858)) ;
#16205=CARTESIAN_POINT('Ctrl Pts',(33.2,40.9075073809612,42.9053907954888)) ;
#16206=CARTESIAN_POINT('Ctrl Pts',(33.2770142912005,40.8463957065363,42.846486106082)) ;
#16207=CARTESIAN_POINT('Ctrl Pts',(33.35,40.7879031038719,42.7901059033638)) ;
#16208=CARTESIAN_POINT('Origin',(33.6,40.2238570189152,42.9412415963218)) ;
#16209=CARTESIAN_POINT('',(33.35,40.2238570189152,42.9412415963218)) ;
#16210=CARTESIAN_POINT('Ctrl Pts',(33.35,40.2238570189152,42.9412415963218)) ;
#16211=CARTESIAN_POINT('Ctrl Pts',(33.2770142912001,40.2013910404334,43.019314585479)) ;
#16212=CARTESIAN_POINT('Ctrl Pts',(33.2,40.1779191226171,43.1008833801193)) ;
#16213=CARTESIAN_POINT('',(30.2,40.2238570189152,42.9412415963218)) ;
#16214=CARTESIAN_POINT('',(33.6,40.2238570189152,42.9412415963218)) ;
#16215=CARTESIAN_POINT('',(30.2,40.0853409932026,43.4226076842641)) ;
#16216=CARTESIAN_POINT('Origin',(30.2,40.2629278588902,43.1628233407496)) ;
#16217=CARTESIAN_POINT('',(30.2,40.2238570189152,42.9412415963218)) ;
#16218=CARTESIAN_POINT('Origin',(33.6,40.518656404528,43.3462024860906)) ;
#16219=CARTESIAN_POINT('Ctrl Pts',(33.2,40.321625226856,43.0755441166495)) ;
#16220=CARTESIAN_POINT('Ctrl Pts',(33.2770142912007,40.2716706680542,43.0069223909347)) ;
#16221=CARTESIAN_POINT('Ctrl Pts',(33.35,40.2238570189152,42.9412415963218)) ;
#16222=CARTESIAN_POINT('Origin',(33.6,39.642135623731,42.992135623731)) ;
#16223=CARTESIAN_POINT('',(33.35,39.642135623731,42.992135623731)) ;
#16224=CARTESIAN_POINT('Ctrl Pts',(33.35,39.642135623731,42.992135623731)) ;
#16225=CARTESIAN_POINT('Ctrl Pts',(33.2770142912005,39.6064537216512,43.0651213325304)) ;
#16226=CARTESIAN_POINT('Ctrl Pts',(33.2,39.5691741224636,43.1413750581414)) ;
#16227=CARTESIAN_POINT('',(30.2,39.642135623731,42.992135623731)) ;
#16228=CARTESIAN_POINT('',(33.6,39.642135623731,42.992135623731)) ;
#16229=CARTESIAN_POINT('',(30.2,39.422135623731,43.4421356237309)) ;
#16230=CARTESIAN_POINT('Origin',(30.2,39.642135623731,43.2171356237309)) ;
#16231=CARTESIAN_POINT('',(30.2,39.642135623731,42.992135623731)) ;
#16232=CARTESIAN_POINT('Origin',(33.6,39.8621356237309,43.4421356237309)) ;
#16233=CARTESIAN_POINT('Ctrl Pts',(33.2,39.7150971249983,43.1413750581414)) ;
#16234=CARTESIAN_POINT('Ctrl Pts',(33.2770142912006,39.6778175258107,43.0651213325304)) ;
#16235=CARTESIAN_POINT('Ctrl Pts',(33.35,39.642135623731,42.992135623731)) ;
#16236=CARTESIAN_POINT('Origin',(33.6,39.0604142285467,42.9412415963219)) ;
#16237=CARTESIAN_POINT('',(33.35,39.0604142285467,42.9412415963219)) ;
#16238=CARTESIAN_POINT('Ctrl Pts',(33.35,39.0604142285467,42.9412415963219)) ;
#16239=CARTESIAN_POINT('Ctrl Pts',(33.2770142912007,39.0126005794078,43.0069223909346)) ;
#16240=CARTESIAN_POINT('Ctrl Pts',(33.2,38.9626460206059,43.0755441166495)) ;
#16241=CARTESIAN_POINT('',(30.2,39.0604142285467,42.9412415963219)) ;
#16242=CARTESIAN_POINT('',(33.6,39.0604142285467,42.9412415963219)) ;
#16243=CARTESIAN_POINT('',(30.2,38.7656148429339,43.3462024860906)) ;
#16244=CARTESIAN_POINT('Origin',(30.2,39.0213433885717,43.1628233407496)) ;
#16245=CARTESIAN_POINT('',(30.2,39.0604142285467,42.9412415963219)) ;
#16246=CARTESIAN_POINT('Origin',(33.6,39.1989302542593,43.4226076842641)) ;
#16247=CARTESIAN_POINT('Ctrl Pts',(33.2,39.1063521248448,43.1008833801193)) ;
#16248=CARTESIAN_POINT('Ctrl Pts',(33.2770142912004,39.0828802070284,43.0193145854787)) ;
#16249=CARTESIAN_POINT('Ctrl Pts',(33.35,39.0604142285467,42.9412415963219)) ;
#16250=CARTESIAN_POINT('Origin',(33.6,38.4963681435899,42.7901059033638)) ;
#16251=CARTESIAN_POINT('',(33.35,38.4963681435899,42.7901059033638)) ;
#16252=CARTESIAN_POINT('Ctrl Pts',(33.35,38.4963681435899,42.7901059033638)) ;
#16253=CARTESIAN_POINT('Ctrl Pts',(33.2770142912005,38.4378755409257,42.846486106082)) ;
#16254=CARTESIAN_POINT('Ctrl Pts',(33.2,38.3767638665007,42.9053907954888)) ;
#16255=CARTESIAN_POINT('',(30.2,38.4963681435899,42.7901059033638)) ;
#16256=CARTESIAN_POINT('',(33.6,38.4963681435899,42.7901059033638)) ;
#16257=CARTESIAN_POINT('',(30.2,38.1357267025205,43.1377231511858)) ;
#16258=CARTESIAN_POINT('Origin',(30.2,38.4194136113417,43.0015367430406)) ;
#16259=CARTESIAN_POINT('',(30.2,38.4963681435899,42.7901059033638)) ;
#16260=CARTESIAN_POINT('Origin',(33.6,38.5491914556663,43.288212014249)) ;
#16261=CARTESIAN_POINT('Ctrl Pts',(33.2,38.5138866351854,42.9552994017302)) ;
#16262=CARTESIAN_POINT('Ctrl Pts',(33.2770142912004,38.5049355810856,42.870893964609)) ;
#16263=CARTESIAN_POINT('Ctrl Pts',(33.35,38.4963681435899,42.7901059033637)) ;
#16264=CARTESIAN_POINT('Origin',(33.6,37.967135623731,42.5433207264088)) ;
#16265=CARTESIAN_POINT('',(33.35,37.967135623731,42.5433207264088)) ;
#16266=CARTESIAN_POINT('Ctrl Pts',(33.35,37.967135623731,42.5433207264088)) ;
#16267=CARTESIAN_POINT('Ctrl Pts',(33.2770142912002,37.8997413356745,42.5886872533027)) ;
#16268=CARTESIAN_POINT('Ctrl Pts',(33.2,37.82932939293,42.636085117221)) ;
#16269=CARTESIAN_POINT('',(30.2,37.967135623731,42.5433207264088)) ;
#16270=CARTESIAN_POINT('',(33.6,37.967135623731,42.5433207264088)) ;
#16271=CARTESIAN_POINT('',(30.2,37.5516100348984,42.8230321581118)) ;
#16272=CARTESIAN_POINT('Origin',(30.2,37.854635623731,42.7381764422603)) ;
#16273=CARTESIAN_POINT('',(30.2,37.967135623731,42.5433207264088)) ;
#16274=CARTESIAN_POINT('Origin',(33.6,37.9326612125635,43.0430321581118)) ;
#16275=CARTESIAN_POINT('Ctrl Pts',(33.2,37.9557024201215,42.7090466184883)) ;
#16276=CARTESIAN_POINT('Ctrl Pts',(33.2770142912003,37.9615442029876,42.6243691553826)) ;
#16277=CARTESIAN_POINT('Ctrl Pts',(33.35,37.967135623731,42.5433207264088)) ;
#16278=CARTESIAN_POINT('Origin',(33.6,37.488797131281,42.2083845081795)) ;
#16279=CARTESIAN_POINT('',(33.35,37.488797131281,42.2083845081795)) ;
#16280=CARTESIAN_POINT('Ctrl Pts',(33.35,37.488797131281,42.2083845081795)) ;
#16281=CARTESIAN_POINT('Ctrl Pts',(33.2770142912006,37.4145488991726,42.2413589202855)) ;
#16282=CARTESIAN_POINT('Ctrl Pts',(33.2,37.336976119358,42.2758097986051)) ;
#16283=CARTESIAN_POINT('',(30.2,37.488797131281,42.2083845081795)) ;
#16284=CARTESIAN_POINT('',(33.6,37.488797131281,42.2083845081795)) ;
#16285=CARTESIAN_POINT('',(30.2,37.0310129294359,42.411691233452)) ;
#16286=CARTESIAN_POINT('Origin',(30.2,37.3441699191016,42.3807445078813)) ;
#16287=CARTESIAN_POINT('',(30.2,37.488797131281,42.2083845081795)) ;
#16288=CARTESIAN_POINT('Origin',(33.6,37.3680724844083,42.6945177817141)) ;
#16289=CARTESIAN_POINT('Ctrl Pts',(33.2,37.4487596245728,42.3696072966026)) ;
#16290=CARTESIAN_POINT('Ctrl Pts',(33.2770142912007,37.4692167447887,42.2872306893791)) ;
#16291=CARTESIAN_POINT('Ctrl Pts',(33.35,37.488797131281,42.2083845081795)) ;
#16292=CARTESIAN_POINT('Origin',(33.6,37.0758867392824,41.7954741161808)) ;
#16293=CARTESIAN_POINT('',(33.35,37.0758867392824,41.7954741161808)) ;
#16294=CARTESIAN_POINT('Ctrl Pts',(33.35,37.0758867392824,41.7954741161808)) ;
#16295=CARTESIAN_POINT('Ctrl Pts',(33.2770142912004,36.9970405580823,41.8150545026733)) ;
#16296=CARTESIAN_POINT('Ctrl Pts',(33.2,36.9146639508593,41.835511622889)) ;
#16297=CARTESIAN_POINT('',(30.2,37.0758867392824,41.7954741161808)) ;
#16298=CARTESIAN_POINT('',(33.6,37.0758867392824,41.7954741161808)) ;
#16299=CARTESIAN_POINT('',(30.2,36.5897534657478,41.9161987630536)) ;
#16300=CARTESIAN_POINT('Origin',(30.2,36.9035267395806,41.9401013283603)) ;
#16301=CARTESIAN_POINT('',(30.2,37.0758867392824,41.7954741161808)) ;
#16302=CARTESIAN_POINT('Origin',(33.6,36.8725800140099,42.253258318026)) ;
#16303=CARTESIAN_POINT('Ctrl Pts',(33.2,37.0084614488568,41.9472951281039)) ;
#16304=CARTESIAN_POINT('Ctrl Pts',(33.2770142912006,37.0429123271764,41.8697223482894)) ;
#16305=CARTESIAN_POINT('Ctrl Pts',(33.35,37.0758867392824,41.7954741161808)) ;
#16306=CARTESIAN_POINT('Origin',(33.6,36.7409505210531,41.3171356237309)) ;
#16307=CARTESIAN_POINT('',(33.35,36.7409505210531,41.3171356237309)) ;
#16308=CARTESIAN_POINT('Ctrl Pts',(33.35,36.7409505210531,41.3171356237309)) ;
#16309=CARTESIAN_POINT('Ctrl Pts',(33.2770142912004,36.6599020920795,41.3227270444743)) ;
#16310=CARTESIAN_POINT('Ctrl Pts',(33.2,36.5752246289736,41.3285688273404)) ;
#16311=CARTESIAN_POINT('',(30.2,36.7409505210531,41.3171356237309)) ;
#16312=CARTESIAN_POINT('',(33.6,36.7409505210531,41.3171356237309)) ;
#16313=CARTESIAN_POINT('',(30.2,36.2412390893501,41.3516100348984)) ;
#16314=CARTESIAN_POINT('Origin',(30.2,36.5460948052016,41.4296356237309)) ;
#16315=CARTESIAN_POINT('',(30.2,36.7409505210531,41.3171356237309)) ;
#16316=CARTESIAN_POINT('Origin',(33.6,36.4612390893501,41.7326612125635)) ;
#16317=CARTESIAN_POINT('Ctrl Pts',(33.2,36.6481861302409,41.4549418545319)) ;
#16318=CARTESIAN_POINT('Ctrl Pts',(33.2770142912004,36.6955839941593,41.3845299117872)) ;
#16319=CARTESIAN_POINT('Ctrl Pts',(33.35,36.7409505210531,41.3171356237309)) ;
#16320=CARTESIAN_POINT('Origin',(33.6,36.4941653440982,40.7879031038719)) ;
#16321=CARTESIAN_POINT('',(33.35,36.4941653440982,40.7879031038719)) ;
#16322=CARTESIAN_POINT('Ctrl Pts',(33.35,36.4941653440982,40.7879031038719)) ;
#16323=CARTESIAN_POINT('Ctrl Pts',(33.2770142912004,36.4133772828529,40.7793356663763)) ;
#16324=CARTESIAN_POINT('Ctrl Pts',(33.2,36.3289718457317,40.7703846122765)) ;
#16325=CARTESIAN_POINT('',(30.2,36.4941653440982,40.7879031038719)) ;
#16326=CARTESIAN_POINT('',(33.6,36.4941653440982,40.7879031038719)) ;
#16327=CARTESIAN_POINT('',(30.2,35.9960592332129,40.7350797917956)) ;
#16328=CARTESIAN_POINT('Origin',(30.2,36.2827345044213,40.8648576361202)) ;
#16329=CARTESIAN_POINT('',(30.2,36.4941653440982,40.7879031038719)) ;
#16330=CARTESIAN_POINT('Origin',(33.6,36.1465480962761,41.1485445449414)) ;
#16331=CARTESIAN_POINT('Ctrl Pts',(33.2,36.3788804519731,40.9075073809612)) ;
#16332=CARTESIAN_POINT('Ctrl Pts',(33.2770142912005,36.4377851413799,40.8463957065362)) ;
#16333=CARTESIAN_POINT('Ctrl Pts',(33.35,36.4941653440982,40.7879031038719)) ;
#16334=CARTESIAN_POINT('Origin',(33.6,36.34302965114,40.2238570189152)) ;
#16335=CARTESIAN_POINT('',(33.35,36.34302965114,40.2238570189152)) ;
#16336=CARTESIAN_POINT('Ctrl Pts',(33.35,36.34302965114,40.2238570189152)) ;
#16337=CARTESIAN_POINT('Ctrl Pts',(33.2770142912004,36.2649566619833,40.2013910404335)) ;
#16338=CARTESIAN_POINT('Ctrl Pts',(33.2,36.1833878673426,40.1779191226171)) ;
#16339=CARTESIAN_POINT('',(30.2,36.34302965114,40.2238570189152)) ;
#16340=CARTESIAN_POINT('',(33.6,36.34302965114,40.2238570189152)) ;
#16341=CARTESIAN_POINT('',(30.2,35.8616635631979,40.0853409932026)) ;
#16342=CARTESIAN_POINT('Origin',(30.2,36.1214479067123,40.2629278588902)) ;
#16343=CARTESIAN_POINT('',(30.2,36.34302965114,40.2238570189152)) ;
#16344=CARTESIAN_POINT('Origin',(33.6,35.9380687613713,40.518656404528)) ;
#16345=CARTESIAN_POINT('Ctrl Pts',(33.2,36.2087271308124,40.321625226856)) ;
#16346=CARTESIAN_POINT('Ctrl Pts',(33.2770142912008,36.2773488565273,40.2716706680541)) ;
#16347=CARTESIAN_POINT('Ctrl Pts',(33.35,36.34302965114,40.2238570189152)) ;
#16348=CARTESIAN_POINT('Origin',(33.6,36.2921356237309,39.642135623731)) ;
#16349=CARTESIAN_POINT('',(33.35,36.2921356237309,39.642135623731)) ;
#16350=CARTESIAN_POINT('Ctrl Pts',(33.35,36.2921356237309,39.642135623731)) ;
#16351=CARTESIAN_POINT('Ctrl Pts',(33.2770142912004,36.2191499149313,39.6064537216511)) ;
#16352=CARTESIAN_POINT('Ctrl Pts',(33.2,36.1428961893205,39.5691741224637)) ;
#16353=CARTESIAN_POINT('',(30.2,36.2921356237309,39.642135623731)) ;
#16354=CARTESIAN_POINT('',(33.6,36.2921356237309,39.642135623731)) ;
#16355=CARTESIAN_POINT('',(30.2,35.842135623731,39.422135623731)) ;
#16356=CARTESIAN_POINT('Origin',(30.2,36.067135623731,39.642135623731)) ;
#16357=CARTESIAN_POINT('',(30.2,36.2921356237309,39.642135623731)) ;
#16358=CARTESIAN_POINT('Origin',(33.6,35.842135623731,39.862135623731)) ;
#16359=CARTESIAN_POINT('Ctrl Pts',(33.2,36.1428961893205,39.7150971249983)) ;
#16360=CARTESIAN_POINT('Ctrl Pts',(33.2770142912002,36.2191499149312,39.6778175258108)) ;
#16361=CARTESIAN_POINT('Ctrl Pts',(33.35,36.2921356237309,39.642135623731)) ;
#16362=CARTESIAN_POINT('Origin',(33.6,36.34302965114,39.0604142285467)) ;
#16363=CARTESIAN_POINT('',(33.35,36.34302965114,39.0604142285467)) ;
#16364=CARTESIAN_POINT('Ctrl Pts',(33.35,36.34302965114,39.0604142285467)) ;
#16365=CARTESIAN_POINT('Ctrl Pts',(33.2770142912004,36.277348856527,39.0126005794075)) ;
#16366=CARTESIAN_POINT('Ctrl Pts',(33.2,36.2087271308124,38.9626460206059)) ;
#16367=CARTESIAN_POINT('',(30.2,36.34302965114,39.0604142285467)) ;
#16368=CARTESIAN_POINT('',(33.6,36.34302965114,39.0604142285467)) ;
#16369=CARTESIAN_POINT('',(30.2,35.9380687613713,38.7656148429339)) ;
#16370=CARTESIAN_POINT('Origin',(30.2,36.1214479067123,39.0213433885717)) ;
#16371=CARTESIAN_POINT('',(30.2,36.34302965114,39.0604142285467)) ;
#16372=CARTESIAN_POINT('Origin',(33.6,35.8616635631978,39.1989302542593)) ;
#16373=CARTESIAN_POINT('Ctrl Pts',(33.2,36.1833878673426,39.1063521248448)) ;
#16374=CARTESIAN_POINT('Ctrl Pts',(33.2770142912004,36.2649566619833,39.0828802070284)) ;
#16375=CARTESIAN_POINT('Ctrl Pts',(33.35,36.34302965114,39.0604142285467)) ;
#16376=CARTESIAN_POINT('Origin',(33.6,36.4941653440982,38.49636814359)) ;
#16377=CARTESIAN_POINT('',(33.35,36.4941653440982,38.49636814359)) ;
#16378=CARTESIAN_POINT('Ctrl Pts',(33.35,36.4941653440982,38.49636814359)) ;
#16379=CARTESIAN_POINT('Ctrl Pts',(33.2770142912005,36.4377851413798,38.4378755409256)) ;
#16380=CARTESIAN_POINT('Ctrl Pts',(33.2,36.3788804519731,38.3767638665007)) ;
#16381=CARTESIAN_POINT('',(30.2,36.4941653440982,38.49636814359)) ;
#16382=CARTESIAN_POINT('',(33.6,36.4941653440982,38.49636814359)) ;
#16383=CARTESIAN_POINT('',(30.2,36.1465480962762,38.1357267025205)) ;
#16384=CARTESIAN_POINT('Origin',(30.2,36.2827345044213,38.4194136113417)) ;
#16385=CARTESIAN_POINT('',(30.2,36.4941653440982,38.49636814359)) ;
#16386=CARTESIAN_POINT('Origin',(33.6,35.9960592332129,38.5491914556663)) ;
#16387=CARTESIAN_POINT('Ctrl Pts',(33.2,36.3289718457317,38.5138866351854)) ;
#16388=CARTESIAN_POINT('Ctrl Pts',(33.2770142912004,36.4133772828529,38.5049355810856)) ;
#16389=CARTESIAN_POINT('Ctrl Pts',(33.35,36.4941653440982,38.49636814359)) ;
#16390=CARTESIAN_POINT('Origin',(33.6,36.7409505210531,37.9671356237309)) ;
#16391=CARTESIAN_POINT('',(33.35,36.7409505210531,37.9671356237309)) ;
#16392=CARTESIAN_POINT('Ctrl Pts',(33.35,36.7409505210531,37.9671356237309)) ;
#16393=CARTESIAN_POINT('Ctrl Pts',(33.2770142912005,36.6955839941594,37.8997413356748)) ;
#16394=CARTESIAN_POINT('Ctrl Pts',(33.2,36.6481861302409,37.82932939293)) ;
#16395=CARTESIAN_POINT('',(30.2,36.7409505210531,37.9671356237309)) ;
#16396=CARTESIAN_POINT('',(33.6,36.7409505210531,37.9671356237309)) ;
#16397=CARTESIAN_POINT('',(30.2,36.4612390893501,37.5516100348984)) ;
#16398=CARTESIAN_POINT('Origin',(30.2,36.5460948052016,37.8546356237309)) ;
#16399=CARTESIAN_POINT('',(30.2,36.7409505210531,37.9671356237309)) ;
#16400=CARTESIAN_POINT('Origin',(33.6,36.2412390893501,37.9326612125635)) ;
#16401=CARTESIAN_POINT('Ctrl Pts',(33.2,36.5752246289736,37.9557024201215)) ;
#16402=CARTESIAN_POINT('Ctrl Pts',(33.2770142912003,36.6599020920794,37.9615442029876)) ;
#16403=CARTESIAN_POINT('Ctrl Pts',(33.35,36.7409505210531,37.9671356237309)) ;
#16404=CARTESIAN_POINT('Origin',(33.6,37.0758867392824,37.488797131281)) ;
#16405=CARTESIAN_POINT('',(33.35,37.0758867392824,37.488797131281)) ;
#16406=CARTESIAN_POINT('Ctrl Pts',(33.35,37.0758867392824,37.488797131281)) ;
#16407=CARTESIAN_POINT('Ctrl Pts',(33.2770142912006,37.0429123271764,37.4145488991725)) ;
#16408=CARTESIAN_POINT('Ctrl Pts',(33.2,37.0084614488568,37.336976119358)) ;
#16409=CARTESIAN_POINT('',(30.2,37.0758867392824,37.488797131281)) ;
#16410=CARTESIAN_POINT('',(33.6,37.0758867392824,37.488797131281)) ;
#16411=CARTESIAN_POINT('',(30.2,36.8725800140099,37.0310129294359)) ;
#16412=CARTESIAN_POINT('Origin',(30.2,36.9035267395806,37.3441699191016)) ;
#16413=CARTESIAN_POINT('',(30.2,37.0758867392824,37.488797131281)) ;
#16414=CARTESIAN_POINT('Origin',(33.6,36.5897534657478,37.3680724844083)) ;
#16415=CARTESIAN_POINT('Ctrl Pts',(33.2,36.9146639508593,37.4487596245728)) ;
#16416=CARTESIAN_POINT('Ctrl Pts',(33.2770142912007,36.9970405580828,37.4692167447887)) ;
#16417=CARTESIAN_POINT('Ctrl Pts',(33.35,37.0758867392824,37.488797131281)) ;
#16418=CARTESIAN_POINT('Origin',(33.6,37.488797131281,37.0758867392824)) ;
#16419=CARTESIAN_POINT('',(33.35,37.488797131281,37.0758867392824)) ;
#16420=CARTESIAN_POINT('Ctrl Pts',(33.35,37.488797131281,37.0758867392824)) ;
#16421=CARTESIAN_POINT('Ctrl Pts',(33.2770142912005,37.4692167447886,36.9970405580825)) ;
#16422=CARTESIAN_POINT('Ctrl Pts',(33.2,37.4487596245729,36.9146639508593)) ;
#16423=CARTESIAN_POINT('',(30.2,37.488797131281,37.0758867392824)) ;
#16424=CARTESIAN_POINT('',(33.6,37.488797131281,37.0758867392824)) ;
#16425=CARTESIAN_POINT('',(30.2,37.3680724844083,36.5897534657478)) ;
#16426=CARTESIAN_POINT('Origin',(30.2,37.3441699191016,36.9035267395806)) ;
#16427=CARTESIAN_POINT('',(30.2,37.488797131281,37.0758867392824)) ;
#16428=CARTESIAN_POINT('Origin',(33.6,37.0310129294359,36.8725800140099)) ;
#16429=CARTESIAN_POINT('Ctrl Pts',(33.2,37.336976119358,37.0084614488568)) ;
#16430=CARTESIAN_POINT('Ctrl Pts',(33.2770142912005,37.4145488991724,37.0429123271763)) ;
#16431=CARTESIAN_POINT('Ctrl Pts',(33.35,37.488797131281,37.0758867392824)) ;
#16432=CARTESIAN_POINT('Origin',(33.6,37.967135623731,36.7409505210531)) ;
#16433=CARTESIAN_POINT('',(33.35,37.967135623731,36.7409505210531)) ;
#16434=CARTESIAN_POINT('Ctrl Pts',(33.35,37.967135623731,36.7409505210531)) ;
#16435=CARTESIAN_POINT('Ctrl Pts',(33.2770142912002,37.9615442029876,36.6599020920793)) ;
#16436=CARTESIAN_POINT('Ctrl Pts',(33.2,37.9557024201215,36.5752246289736)) ;
#16437=CARTESIAN_POINT('',(30.2,37.967135623731,36.7409505210531)) ;
#16438=CARTESIAN_POINT('',(33.6,37.967135623731,36.7409505210531)) ;
#16439=CARTESIAN_POINT('',(30.2,37.9326612125635,36.2412390893501)) ;
#16440=CARTESIAN_POINT('Origin',(30.2,37.854635623731,36.5460948052016)) ;
#16441=CARTESIAN_POINT('',(30.2,37.967135623731,36.7409505210531)) ;
#16442=CARTESIAN_POINT('Origin',(33.6,37.5516100348984,36.4612390893501)) ;
#16443=CARTESIAN_POINT('Ctrl Pts',(33.2,37.82932939293,36.6481861302409)) ;
#16444=CARTESIAN_POINT('Ctrl Pts',(33.2770142912006,37.8997413356749,36.6955839941594)) ;
#16445=CARTESIAN_POINT('Ctrl Pts',(33.35,37.967135623731,36.7409505210531)) ;
#16446=CARTESIAN_POINT('Origin',(33.6,38.49636814359,36.4941653440981)) ;
#16447=CARTESIAN_POINT('',(33.35,38.49636814359,36.4941653440981)) ;
#16448=CARTESIAN_POINT('Ctrl Pts',(33.35,38.49636814359,36.4941653440981)) ;
#16449=CARTESIAN_POINT('Ctrl Pts',(33.2770142912006,38.5049355810856,36.4133772828531)) ;
#16450=CARTESIAN_POINT('Ctrl Pts',(33.2,38.5138866351854,36.3289718457317)) ;
#16451=CARTESIAN_POINT('',(30.2,38.49636814359,36.4941653440981)) ;
#16452=CARTESIAN_POINT('',(33.6,38.49636814359,36.4941653440981)) ;
#16453=CARTESIAN_POINT('',(30.2,38.5491914556663,35.9960592332129)) ;
#16454=CARTESIAN_POINT('Origin',(30.2,38.4194136113417,36.2827345044213)) ;
#16455=CARTESIAN_POINT('',(30.2,38.49636814359,36.4941653440981)) ;
#16456=CARTESIAN_POINT('Origin',(33.6,38.1357267025205,36.1465480962761)) ;
#16457=CARTESIAN_POINT('Ctrl Pts',(33.2,38.3767638665007,36.3788804519731)) ;
#16458=CARTESIAN_POINT('Ctrl Pts',(33.2770142912005,38.4378755409256,36.4377851413798)) ;
#16459=CARTESIAN_POINT('Ctrl Pts',(33.35,38.49636814359,36.4941653440981)) ;
#16460=CARTESIAN_POINT('Origin',(33.6,39.0604142285467,36.34302965114)) ;
#16461=CARTESIAN_POINT('',(33.35,39.0604142285467,36.34302965114)) ;
#16462=CARTESIAN_POINT('Ctrl Pts',(33.35,39.0604142285467,36.34302965114)) ;
#16463=CARTESIAN_POINT('Ctrl Pts',(33.2770142912002,39.0828802070284,36.2649566619831)) ;
#16464=CARTESIAN_POINT('Ctrl Pts',(33.2,39.1063521248448,36.1833878673426)) ;
#16465=CARTESIAN_POINT('',(30.2,39.0604142285467,36.34302965114)) ;
#16466=CARTESIAN_POINT('',(33.6,39.0604142285467,36.34302965114)) ;
#16467=CARTESIAN_POINT('',(30.2,39.1989302542593,35.8616635631978)) ;
#16468=CARTESIAN_POINT('Origin',(30.2,39.0213433885717,36.1214479067123)) ;
#16469=CARTESIAN_POINT('',(30.2,39.0604142285467,36.34302965114)) ;
#16470=CARTESIAN_POINT('Origin',(33.6,38.7656148429339,35.9380687613713)) ;
#16471=CARTESIAN_POINT('Ctrl Pts',(33.2,38.9626460206059,36.2087271308124)) ;
#16472=CARTESIAN_POINT('Ctrl Pts',(33.2770142912006,39.0126005794077,36.2773488565272)) ;
#16473=CARTESIAN_POINT('Ctrl Pts',(33.35,39.0604142285467,36.34302965114)) ;
#16474=CARTESIAN_POINT('Origin',(33.6,39.642135623731,36.2921356237309)) ;
#16475=CARTESIAN_POINT('',(33.35,39.642135623731,36.2921356237309)) ;
#16476=CARTESIAN_POINT('Ctrl Pts',(33.35,39.642135623731,36.2921356237309)) ;
#16477=CARTESIAN_POINT('Ctrl Pts',(33.2770142912005,39.6778175258107,36.2191499149314)) ;
#16478=CARTESIAN_POINT('Ctrl Pts',(33.2,39.7150971249983,36.1428961893205)) ;
#16479=CARTESIAN_POINT('',(30.2,39.642135623731,36.2921356237309)) ;
#16480=CARTESIAN_POINT('',(33.6,39.642135623731,36.2921356237309)) ;
#16481=CARTESIAN_POINT('',(30.2,39.8621356237309,35.8421356237309)) ;
#16482=CARTESIAN_POINT('Origin',(30.2,39.642135623731,36.0671356237309)) ;
#16483=CARTESIAN_POINT('',(30.2,39.642135623731,36.2921356237309)) ;
#16484=CARTESIAN_POINT('Origin',(33.6,39.422135623731,35.8421356237309)) ;
#16485=CARTESIAN_POINT('Ctrl Pts',(33.2,39.5691741224637,36.1428961893205)) ;
#16486=CARTESIAN_POINT('Ctrl Pts',(33.2770142912005,39.6064537216512,36.2191499149315)) ;
#16487=CARTESIAN_POINT('Ctrl Pts',(33.35,39.642135623731,36.2921356237309)) ;
#16488=CARTESIAN_POINT('Origin',(33.6,40.2238570189152,36.34302965114)) ;
#16489=CARTESIAN_POINT('',(33.35,40.2238570189152,36.34302965114)) ;
#16490=CARTESIAN_POINT('Ctrl Pts',(33.35,40.2238570189152,36.34302965114)) ;
#16491=CARTESIAN_POINT('Ctrl Pts',(33.2770142912005,40.2716706680543,36.277348856527)) ;
#16492=CARTESIAN_POINT('Ctrl Pts',(33.2,40.321625226856,36.2087271308124)) ;
#16493=CARTESIAN_POINT('',(30.2,40.2238570189152,36.34302965114)) ;
#16494=CARTESIAN_POINT('',(33.6,40.2238570189152,36.34302965114)) ;
#16495=CARTESIAN_POINT('',(30.2,40.518656404528,35.9380687613713)) ;
#16496=CARTESIAN_POINT('Origin',(30.2,40.2629278588902,36.1214479067123)) ;
#16497=CARTESIAN_POINT('',(30.2,40.2238570189152,36.34302965114)) ;
#16498=CARTESIAN_POINT('Origin',(33.6,40.0853409932026,35.8616635631978)) ;
#16499=CARTESIAN_POINT('Ctrl Pts',(33.2,40.1779191226171,36.1833878673426)) ;
#16500=CARTESIAN_POINT('Ctrl Pts',(33.2770142912004,40.2013910404335,36.2649566619833)) ;
#16501=CARTESIAN_POINT('Ctrl Pts',(33.35,40.2238570189152,36.34302965114)) ;
#16502=CARTESIAN_POINT('Origin',(33.6,40.7879031038719,36.4941653440982)) ;
#16503=CARTESIAN_POINT('',(33.35,40.7879031038719,36.4941653440982)) ;
#16504=CARTESIAN_POINT('Ctrl Pts',(33.35,40.7879031038719,36.4941653440982)) ;
#16505=CARTESIAN_POINT('Ctrl Pts',(33.2770142912003,40.8463957065363,36.4377851413798)) ;
#16506=CARTESIAN_POINT('Ctrl Pts',(33.2,40.9075073809612,36.3788804519731)) ;
#16507=CARTESIAN_POINT('',(30.2,40.7879031038719,36.4941653440982)) ;
#16508=CARTESIAN_POINT('',(33.6,40.7879031038719,36.4941653440982)) ;
#16509=CARTESIAN_POINT('',(30.2,41.1485445449414,36.1465480962762)) ;
#16510=CARTESIAN_POINT('Origin',(30.2,40.8648576361202,36.2827345044213)) ;
#16511=CARTESIAN_POINT('',(30.2,40.7879031038719,36.4941653440982)) ;
#16512=CARTESIAN_POINT('Origin',(33.6,40.7350797917956,35.9960592332129)) ;
#16513=CARTESIAN_POINT('Ctrl Pts',(33.2,40.7703846122765,36.3289718457317)) ;
#16514=CARTESIAN_POINT('Ctrl Pts',(33.2770142912004,40.7793356663763,36.4133772828528)) ;
#16515=CARTESIAN_POINT('Ctrl Pts',(33.35,40.7879031038719,36.4941653440982)) ;
#16516=CARTESIAN_POINT('Origin',(33.6,41.3171356237309,36.7409505210531)) ;
#16517=CARTESIAN_POINT('',(33.35,41.3171356237309,36.7409505210531)) ;
#16518=CARTESIAN_POINT('Ctrl Pts',(33.35,41.3171356237309,36.7409505210531)) ;
#16519=CARTESIAN_POINT('Ctrl Pts',(33.277014291201,41.3845299117866,36.6955839941597)) ;
#16520=CARTESIAN_POINT('Ctrl Pts',(33.2,41.4549418545319,36.6481861302409)) ;
#16521=CARTESIAN_POINT('',(30.2,41.3171356237309,36.7409505210531)) ;
#16522=CARTESIAN_POINT('',(33.6,41.3171356237309,36.7409505210531)) ;
#16523=CARTESIAN_POINT('',(30.2,41.7326612125635,36.4612390893501)) ;
#16524=CARTESIAN_POINT('Origin',(30.2,41.429635623731,36.5460948052016)) ;
#16525=CARTESIAN_POINT('',(30.2,41.3171356237309,36.7409505210531)) ;
#16526=CARTESIAN_POINT('Origin',(33.6,41.3516100348984,36.2412390893501)) ;
#16527=CARTESIAN_POINT('Ctrl Pts',(33.2,41.3285688273404,36.5752246289736)) ;
#16528=CARTESIAN_POINT('Ctrl Pts',(33.2770142912007,41.3227270444743,36.6599020920798)) ;
#16529=CARTESIAN_POINT('Ctrl Pts',(33.35,41.3171356237309,36.7409505210531)) ;
#16530=CARTESIAN_POINT('Origin',(33.6,41.7954741161808,37.0758867392824)) ;
#16531=CARTESIAN_POINT('',(33.35,41.7954741161808,37.0758867392824)) ;
#16532=CARTESIAN_POINT('Ctrl Pts',(33.35,41.7954741161808,37.0758867392824)) ;
#16533=CARTESIAN_POINT('Ctrl Pts',(33.2770142912011,41.8697223482889,37.0429123271766)) ;
#16534=CARTESIAN_POINT('Ctrl Pts',(33.2,41.9472951281039,37.0084614488568)) ;
#16535=CARTESIAN_POINT('',(30.2,41.7954741161808,37.0758867392824)) ;
#16536=CARTESIAN_POINT('',(33.6,41.7954741161808,37.0758867392824)) ;
#16537=CARTESIAN_POINT('',(30.2,42.253258318026,36.8725800140099)) ;
#16538=CARTESIAN_POINT('Origin',(30.2,41.9401013283603,36.9035267395806)) ;
#16539=CARTESIAN_POINT('',(30.2,41.7954741161808,37.0758867392824)) ;
#16540=CARTESIAN_POINT('Origin',(33.6,41.9161987630536,36.5897534657478)) ;
#16541=CARTESIAN_POINT('Ctrl Pts',(33.2,41.835511622889,36.9146639508593)) ;
#16542=CARTESIAN_POINT('Ctrl Pts',(33.2770142912009,41.8150545026731,36.9970405580829)) ;
#16543=CARTESIAN_POINT('Ctrl Pts',(33.35,41.7954741161808,37.0758867392824)) ;
#16544=CARTESIAN_POINT('Origin',(33.6,42.2083845081795,37.488797131281)) ;
#16545=CARTESIAN_POINT('',(33.35,42.2083845081795,37.488797131281)) ;
#16546=CARTESIAN_POINT('Ctrl Pts',(33.35,42.2083845081795,37.488797131281)) ;
#16547=CARTESIAN_POINT('Ctrl Pts',(33.2770142912011,42.2872306893787,37.4692167447888)) ;
#16548=CARTESIAN_POINT('Ctrl Pts',(33.2,42.3696072966026,37.4487596245728)) ;
#16549=CARTESIAN_POINT('',(30.2,42.2083845081795,37.488797131281)) ;
#16550=CARTESIAN_POINT('',(33.6,42.2083845081795,37.488797131281)) ;
#16551=CARTESIAN_POINT('',(30.2,42.6945177817141,37.3680724844083)) ;
#16552=CARTESIAN_POINT('Origin',(30.2,42.3807445078813,37.3441699191016)) ;
#16553=CARTESIAN_POINT('',(30.2,42.2083845081795,37.488797131281)) ;
#16554=CARTESIAN_POINT('Origin',(33.6,42.411691233452,37.0310129294359)) ;
#16555=CARTESIAN_POINT('Ctrl Pts',(33.2,42.2758097986051,37.336976119358)) ;
#16556=CARTESIAN_POINT('Ctrl Pts',(33.2770142912009,42.2413589202854,37.4145488991728)) ;
#16557=CARTESIAN_POINT('Ctrl Pts',(33.35,42.2083845081795,37.488797131281)) ;
#16558=CARTESIAN_POINT('Origin',(33.6,42.5433207264088,37.967135623731)) ;
#16559=CARTESIAN_POINT('',(33.35,42.5433207264088,37.967135623731)) ;
#16560=CARTESIAN_POINT('Ctrl Pts',(33.35,42.5433207264088,37.967135623731)) ;
#16561=CARTESIAN_POINT('Ctrl Pts',(33.2770142912005,42.6243691553823,37.9615442029876)) ;
#16562=CARTESIAN_POINT('Ctrl Pts',(33.2,42.7090466184883,37.9557024201215)) ;
#16563=CARTESIAN_POINT('',(30.2,42.5433207264088,37.967135623731)) ;
#16564=CARTESIAN_POINT('',(33.6,42.5433207264088,37.967135623731)) ;
#16565=CARTESIAN_POINT('',(30.2,43.0430321581118,37.9326612125635)) ;
#16566=CARTESIAN_POINT('Origin',(30.2,42.7381764422603,37.854635623731)) ;
#16567=CARTESIAN_POINT('',(30.2,42.5433207264088,37.967135623731)) ;
#16568=CARTESIAN_POINT('Origin',(33.6,42.8230321581118,37.5516100348984)) ;
#16569=CARTESIAN_POINT('Ctrl Pts',(33.2,42.636085117221,37.82932939293)) ;
#16570=CARTESIAN_POINT('Ctrl Pts',(33.2770142912006,42.5886872533024,37.8997413356749)) ;
#16571=CARTESIAN_POINT('Ctrl Pts',(33.35,42.5433207264088,37.967135623731)) ;
#16572=CARTESIAN_POINT('Origin',(33.6,42.7901059033638,38.49636814359)) ;
#16573=CARTESIAN_POINT('',(33.35,42.7901059033638,38.49636814359)) ;
#16574=CARTESIAN_POINT('Ctrl Pts',(33.35,42.7901059033638,38.49636814359)) ;
#16575=CARTESIAN_POINT('Ctrl Pts',(33.2770142912007,42.8708939646087,38.5049355810856)) ;
#16576=CARTESIAN_POINT('Ctrl Pts',(33.2,42.9552994017302,38.5138866351854)) ;
#16577=CARTESIAN_POINT('',(30.2,42.7901059033638,38.49636814359)) ;
#16578=CARTESIAN_POINT('',(33.6,42.7901059033638,38.49636814359)) ;
#16579=CARTESIAN_POINT('',(30.2,43.288212014249,38.5491914556663)) ;
#16580=CARTESIAN_POINT('Origin',(30.2,43.0015367430406,38.4194136113417)) ;
#16581=CARTESIAN_POINT('',(30.2,42.7901059033638,38.49636814359)) ;
#16582=CARTESIAN_POINT('Origin',(33.6,43.1377231511858,38.1357267025205)) ;
#16583=CARTESIAN_POINT('Ctrl Pts',(33.2,42.9053907954888,38.3767638665007)) ;
#16584=CARTESIAN_POINT('Ctrl Pts',(33.2770142912009,42.8464861060817,38.437875540926)) ;
#16585=CARTESIAN_POINT('Ctrl Pts',(33.35,42.7901059033638,38.49636814359)) ;
#16586=CARTESIAN_POINT('Origin',(33.6,42.9412415963219,39.0604142285467)) ;
#16587=CARTESIAN_POINT('',(33.35,42.9412415963219,39.0604142285467)) ;
#16588=CARTESIAN_POINT('Ctrl Pts',(33.35,42.9412415963219,39.0604142285467)) ;
#16589=CARTESIAN_POINT('Ctrl Pts',(33.2770142912008,43.0193145854782,39.0828802070282)) ;
#16590=CARTESIAN_POINT('Ctrl Pts',(33.2,43.1008833801193,39.1063521248448)) ;
#16591=CARTESIAN_POINT('',(30.2,42.9412415963219,39.0604142285467)) ;
#16592=CARTESIAN_POINT('',(33.6,42.9412415963219,39.0604142285467)) ;
#16593=CARTESIAN_POINT('',(30.2,43.4226076842641,39.1989302542593)) ;
#16594=CARTESIAN_POINT('Origin',(30.2,43.1628233407496,39.0213433885717)) ;
#16595=CARTESIAN_POINT('',(30.2,42.9412415963219,39.0604142285467)) ;
#16596=CARTESIAN_POINT('Origin',(33.6,43.3462024860906,38.7656148429339)) ;
#16597=CARTESIAN_POINT('Ctrl Pts',(33.2,43.0755441166495,38.9626460206059)) ;
#16598=CARTESIAN_POINT('Ctrl Pts',(33.2770142912008,43.0069223909346,39.0126005794078)) ;
#16599=CARTESIAN_POINT('Ctrl Pts',(33.35,42.9412415963219,39.0604142285467)) ;
#16600=CARTESIAN_POINT('Origin',(33.6,42.992135623731,39.642135623731)) ;
#16601=CARTESIAN_POINT('',(33.35,42.992135623731,39.642135623731)) ;
#16602=CARTESIAN_POINT('Ctrl Pts',(33.35,42.992135623731,39.642135623731)) ;
#16603=CARTESIAN_POINT('Ctrl Pts',(33.2770142912007,43.0651213325302,39.6778175258106)) ;
#16604=CARTESIAN_POINT('Ctrl Pts',(33.2,43.1413750581413,39.7150971249983)) ;
#16605=CARTESIAN_POINT('',(30.2,42.992135623731,39.642135623731)) ;
#16606=CARTESIAN_POINT('',(33.6,42.992135623731,39.642135623731)) ;
#16607=CARTESIAN_POINT('',(30.2,43.4421356237309,39.8621356237309)) ;
#16608=CARTESIAN_POINT('Origin',(30.2,43.2171356237309,39.642135623731)) ;
#16609=CARTESIAN_POINT('',(30.2,42.992135623731,39.642135623731)) ;
#16610=CARTESIAN_POINT('Origin',(33.6,43.4421356237309,39.422135623731)) ;
#16611=CARTESIAN_POINT('Ctrl Pts',(33.2,43.1413750581413,39.5691741224637)) ;
#16612=CARTESIAN_POINT('Ctrl Pts',(33.2770142912006,43.0651213325304,39.6064537216512)) ;
#16613=CARTESIAN_POINT('Ctrl Pts',(33.35,42.992135623731,39.642135623731)) ;
#16614=CARTESIAN_POINT('Origin',(29.8,39.642135623731,39.642135623731)) ;
#16615=CARTESIAN_POINT('Origin',(29.8,39.642135623731,42.9421356237309)) ;
#16616=CARTESIAN_POINT('Origin',(33.4,39.642135623731,39.642135623731)) ;
#16617=CARTESIAN_POINT('',(33.6,39.642135623731,42.742135623731)) ;
#16618=CARTESIAN_POINT('Origin',(33.6,39.642135623731,39.642135623731)) ;
#16619=CARTESIAN_POINT('',(33.4,39.642135623731,42.9421356237309)) ;
#16620=CARTESIAN_POINT('Origin',(33.6,39.642135623731,39.642135623731)) ;
#16621=CARTESIAN_POINT('',(33.6,37.6600848161621,39.6421356)) ;
#16622=CARTESIAN_POINT('Origin',(33.6,39.642135623731,39.6421356)) ;
#16623=CARTESIAN_POINT('Origin',(33.45,39.642135623731,39.6421356)) ;
#16624=CARTESIAN_POINT('',(33.3,38.8810214088786,41.142135623731)) ;
#16625=CARTESIAN_POINT('',(33.3500000205516,38.7761102199465,41.142135623731)) ;
#16626=CARTESIAN_POINT('Ctrl Pts',(33.3,38.8810214088786,41.142135623731)) ;
#16627=CARTESIAN_POINT('Ctrl Pts',(33.3233881136867,38.8293340343079,41.142135623731)) ;
#16628=CARTESIAN_POINT('Ctrl Pts',(33.3500000205516,38.7761102199465,41.142135623731)) ;
#16629=CARTESIAN_POINT('',(33.3,40.4032498385833,41.142135623731)) ;
#16630=CARTESIAN_POINT('Origin',(33.3,39.642135623731,39.6421356)) ;
#16631=CARTESIAN_POINT('',(33.3500000205516,40.5081610275154,41.142135623731)) ;
#16632=CARTESIAN_POINT('Ctrl Pts',(33.3500000205516,40.5081610275154,41.142135623731)) ;
#16633=CARTESIAN_POINT('Ctrl Pts',(33.3233881136867,40.454937213154,41.142135623731)) ;
#16634=CARTESIAN_POINT('Ctrl Pts',(33.3,40.4032498385833,41.142135623731)) ;
#16635=CARTESIAN_POINT('',(33.3,40.560616620565,41.0512798714278)) ;
#16636=CARTESIAN_POINT('Ctrl Pts',(33.3,40.5606166205651,41.0512798714278)) ;
#16637=CARTESIAN_POINT('Ctrl Pts',(33.3233881137737,40.5347729339775,41.0960424496522)) ;
#16638=CARTESIAN_POINT('Ctrl Pts',(33.3500000205516,40.5081610275154,41.142135623731)) ;
#16639=CARTESIAN_POINT('',(33.3,41.3217308588018,39.7329913404377)) ;
#16640=CARTESIAN_POINT('Origin',(33.3,39.642135623731,39.6421356)) ;
#16641=CARTESIAN_POINT('',(33.35,41.3741864312998,39.642135623731)) ;
#16642=CARTESIAN_POINT('Ctrl Pts',(33.35,41.3741864312998,39.642135623731)) ;
#16643=CARTESIAN_POINT('Ctrl Pts',(33.3233881047513,41.3475745354196,39.6882287794813)) ;
#16644=CARTESIAN_POINT('Ctrl Pts',(33.3,41.3217308588018,39.7329913404377)) ;
#16645=CARTESIAN_POINT('',(33.3,41.3217308616346,39.5512799119308)) ;
#16646=CARTESIAN_POINT('Ctrl Pts',(33.3,41.3217308616346,39.5512799119308)) ;
#16647=CARTESIAN_POINT('Ctrl Pts',(33.3233881049254,41.3475745368567,39.5960424704698)) ;
#16648=CARTESIAN_POINT('Ctrl Pts',(33.35,41.3741864312998,39.642135623731)) ;
#16649=CARTESIAN_POINT('',(33.3,40.560616576629,38.2329912999347)) ;
#16650=CARTESIAN_POINT('Origin',(33.3,39.642135623731,39.6421356)) ;
#16651=CARTESIAN_POINT('',(33.3499999794484,40.5081610275154,38.142135623731)) ;
#16652=CARTESIAN_POINT('Ctrl Pts',(33.3499999794484,40.5081610275154,38.142135623731)) ;
#16653=CARTESIAN_POINT('Ctrl Pts',(33.3233880959029,40.5347729113766,38.1882287586638)) ;
#16654=CARTESIAN_POINT('Ctrl Pts',(33.3,40.560616576629,38.2329912999347)) ;
#16655=CARTESIAN_POINT('',(33.3,40.4032499321209,38.142135623731)) ;
#16656=CARTESIAN_POINT('Ctrl Pts',(33.3,40.4032499321209,38.142135623731)) ;
#16657=CARTESIAN_POINT('Ctrl Pts',(33.3233880959899,40.45493726123,38.142135623731)) ;
#16658=CARTESIAN_POINT('Ctrl Pts',(33.3499999794484,40.5081610275154,38.142135623731)) ;
#16659=CARTESIAN_POINT('',(33.3,38.881021315341,38.142135623731)) ;
#16660=CARTESIAN_POINT('Origin',(33.3,39.642135623731,39.6421356)) ;
#16661=CARTESIAN_POINT('',(33.3499999794484,38.7761102199465,38.142135623731)) ;
#16662=CARTESIAN_POINT('Ctrl Pts',(33.3499999794484,38.7761102199465,38.142135623731)) ;
#16663=CARTESIAN_POINT('Ctrl Pts',(33.32338809599,38.8293339862319,38.142135623731)) ;
#16664=CARTESIAN_POINT('Ctrl Pts',(33.3,38.881021315341,38.142135623731)) ;
#16665=CARTESIAN_POINT('',(33.3,38.7236546708329,38.2329912999347)) ;
#16666=CARTESIAN_POINT('Ctrl Pts',(33.3,38.7236546708329,38.2329912999347)) ;
#16667=CARTESIAN_POINT('Ctrl Pts',(33.3233880959029,38.7494983360852,38.1882287586638)) ;
#16668=CARTESIAN_POINT('Ctrl Pts',(33.3499999794484,38.7761102199465,38.1421356237309)) ;
#16669=CARTESIAN_POINT('',(33.3,37.9625403858273,39.5512799119308)) ;
#16670=CARTESIAN_POINT('Origin',(33.3,39.642135623731,39.6421356)) ;
#16671=CARTESIAN_POINT('',(33.35,37.9100848161621,39.642135623731)) ;
#16672=CARTESIAN_POINT('Ctrl Pts',(33.35,37.9100848161621,39.642135623731)) ;
#16673=CARTESIAN_POINT('Ctrl Pts',(33.3233881049254,37.9366967106052,39.5960424704698)) ;
#16674=CARTESIAN_POINT('Ctrl Pts',(33.3,37.9625403858273,39.5512799119308)) ;
#16675=CARTESIAN_POINT('',(33.45,37.8100848161621,39.6421356)) ;
#16676=CARTESIAN_POINT('',(33.3,37.9625403886601,39.7329913404377)) ;
#16677=CARTESIAN_POINT('Ctrl Pts',(33.3,37.9625403886601,39.7329913404377)) ;
#16678=CARTESIAN_POINT('Ctrl Pts',(33.3233881047512,37.9366967120424,39.6882287794813)) ;
#16679=CARTESIAN_POINT('Ctrl Pts',(33.35,37.9100848161621,39.6421356237309)) ;
#16680=CARTESIAN_POINT('',(33.3,38.7236546268969,41.0512798714278)) ;
#16681=CARTESIAN_POINT('Origin',(33.3,39.642135623731,39.6421356)) ;
#16682=CARTESIAN_POINT('Ctrl Pts',(33.3500000205516,38.7761102199465,41.142135623731)) ;
#16683=CARTESIAN_POINT('Ctrl Pts',(33.3233881137737,38.7494983134844,41.0960424496523)) ;
#16684=CARTESIAN_POINT('Ctrl Pts',(33.3,38.7236546268969,41.0512798714278)) ;
#16685=CARTESIAN_POINT('Origin',(33.45,39.642135623731,39.6421356)) ;
#16686=CARTESIAN_POINT('',(33.6,38.881021315341,38.142135623731)) ;
#16687=CARTESIAN_POINT('',(33.45,38.881021315341,38.142135623731)) ;
#16688=CARTESIAN_POINT('',(33.6,40.4032499321209,38.142135623731)) ;
#16689=CARTESIAN_POINT('',(33.45,40.4032499321209,38.142135623731)) ;
#16690=CARTESIAN_POINT('Origin',(33.6,39.642135623731,39.6421356)) ;
#16691=CARTESIAN_POINT('Origin',(33.45,39.642135623731,39.6421356)) ;
#16692=CARTESIAN_POINT('',(33.6,41.3217308616346,39.5512799119308)) ;
#16693=CARTESIAN_POINT('',(33.45,41.3217308616346,39.5512799119308)) ;
#16694=CARTESIAN_POINT('',(33.6,40.560616576629,38.2329912999347)) ;
#16695=CARTESIAN_POINT('Origin',(33.6,39.642135623731,39.6421356)) ;
#16696=CARTESIAN_POINT('',(33.45,40.560616576629,38.2329912999347)) ;
#16697=CARTESIAN_POINT('Origin',(33.45,39.642135623731,39.6421356)) ;
#16698=CARTESIAN_POINT('',(33.6,37.9625403858273,39.5512799119308)) ;
#16699=CARTESIAN_POINT('',(33.45,37.9625403858273,39.5512799119308)) ;
#16700=CARTESIAN_POINT('',(33.6,38.7236546708329,38.2329912999347)) ;
#16701=CARTESIAN_POINT('',(33.45,38.7236546708329,38.2329912999347)) ;
#16702=CARTESIAN_POINT('Origin',(33.6,39.642135623731,39.6421356)) ;
#16703=CARTESIAN_POINT('Origin',(33.45,39.642135623731,39.6421356)) ;
#16704=CARTESIAN_POINT('',(33.6,40.560616620565,41.0512798714278)) ;
#16705=CARTESIAN_POINT('',(33.45,40.560616620565,41.0512798714278)) ;
#16706=CARTESIAN_POINT('',(33.6,41.3217308588018,39.7329913404377)) ;
#16707=CARTESIAN_POINT('Origin',(33.6,39.642135623731,39.6421356)) ;
#16708=CARTESIAN_POINT('',(33.45,41.3217308588018,39.7329913404377)) ;
#16709=CARTESIAN_POINT('Origin',(33.45,39.642135623731,39.6421356)) ;
#16710=CARTESIAN_POINT('',(33.6,38.7236546268969,41.0512798714278)) ;
#16711=CARTESIAN_POINT('',(33.45,38.7236546268969,41.0512798714278)) ;
#16712=CARTESIAN_POINT('',(33.6,37.9625403886601,39.7329913404377)) ;
#16713=CARTESIAN_POINT('',(33.45,37.9625403886601,39.7329913404377)) ;
#16714=CARTESIAN_POINT('Origin',(33.6,39.642135623731,39.6421356)) ;
#16715=CARTESIAN_POINT('Origin',(33.45,39.642135623731,39.6421356)) ;
#16716=CARTESIAN_POINT('',(33.6,38.8810214088786,41.142135623731)) ;
#16717=CARTESIAN_POINT('',(33.45,38.8810214088786,41.142135623731)) ;
#16718=CARTESIAN_POINT('',(33.6,40.4032498385833,41.142135623731)) ;
#16719=CARTESIAN_POINT('Origin',(33.6,39.642135623731,39.6421356)) ;
#16720=CARTESIAN_POINT('',(33.45,40.4032498385833,41.142135623731)) ;
#16721=CARTESIAN_POINT('Origin',(33.6,37.9100848161621,39.642135623731)) ;
#16722=CARTESIAN_POINT('',(33.6,38.1265911671082,40.017135623731)) ;
#16723=CARTESIAN_POINT('',(31.6,37.9100848161621,39.642135623731)) ;
#16724=CARTESIAN_POINT('',(33.6,37.9100848161621,39.642135623731)) ;
#16725=CARTESIAN_POINT('',(31.6,38.7761102199465,41.142135623731)) ;
#16726=CARTESIAN_POINT('',(31.6,38.7761102199465,41.142135623731)) ;
#16727=CARTESIAN_POINT('',(33.6,38.7761102199465,41.142135623731)) ;
#16728=CARTESIAN_POINT('Origin',(33.6,38.7761102199465,38.142135623731)) ;
#16729=CARTESIAN_POINT('',(33.6,38.5596038690004,38.517135623731)) ;
#16730=CARTESIAN_POINT('',(31.6,38.7761102199465,38.142135623731)) ;
#16731=CARTESIAN_POINT('',(33.6,38.7761102199465,38.142135623731)) ;
#16732=CARTESIAN_POINT('',(31.6,37.9100848161621,39.642135623731)) ;
#16733=CARTESIAN_POINT('Origin',(33.6,40.5081610275154,38.142135623731)) ;
#16734=CARTESIAN_POINT('',(33.6,40.0751483256232,38.142135623731)) ;
#16735=CARTESIAN_POINT('',(31.6,40.5081610275154,38.142135623731)) ;
#16736=CARTESIAN_POINT('',(33.6,40.5081610275154,38.142135623731)) ;
#16737=CARTESIAN_POINT('',(31.6,38.7761102199465,38.142135623731)) ;
#16738=CARTESIAN_POINT('Origin',(33.6,39.642135623731,39.642135623731)) ;
#16739=CARTESIAN_POINT('Origin',(33.6,39.642135623731,39.642135623731)) ;
#16740=CARTESIAN_POINT('Origin',(33.6,39.642135623731,39.642135623731)) ;
#16741=CARTESIAN_POINT('',(33.6,41.1576800803537,39.267135623731)) ;
#16742=CARTESIAN_POINT('Origin',(33.6,39.642135623731,39.642135623731)) ;
#16743=CARTESIAN_POINT('Origin',(33.6,39.642135623731,39.642135623731)) ;
#16744=CARTESIAN_POINT('',(33.6,40.7246673784615,40.7671356237309)) ;
#16745=CARTESIAN_POINT('Origin',(33.6,39.642135623731,39.642135623731)) ;
#16746=CARTESIAN_POINT('',(33.6,39.2091229218387,41.142135623731)) ;
#16747=CARTESIAN_POINT('Origin',(31.6,39.642135623731,39.6421356)) ;
#16748=CARTESIAN_POINT('',(31.6,40.5081610275154,41.142135623731)) ;
#16749=CARTESIAN_POINT('',(31.6,41.3741864312998,39.642135623731)) ;
#16750=CARTESIAN_POINT('',(31.6,41.3741864312998,39.642135623731)) ;
#16751=CARTESIAN_POINT('Origin',(31.6,39.642135623731,39.6421356)) ;
#16752=CARTESIAN_POINT('Origin',(31.6,39.642135623731,39.6421356)) ;
#16753=CARTESIAN_POINT('',(31.6,40.5081610275154,38.142135623731)) ;
#16754=CARTESIAN_POINT('Origin',(31.6,39.642135623731,39.6421356)) ;
#16755=CARTESIAN_POINT('Origin',(31.6,39.642135623731,39.6421356)) ;
#16756=CARTESIAN_POINT('Origin',(31.6,39.642135623731,39.6421356)) ;
#16757=CARTESIAN_POINT('Origin',(31.6,39.642135623731,39.6421356)) ;
#16758=CARTESIAN_POINT('Origin',(31.6,39.642135623731,39.6421356)) ;
#16759=CARTESIAN_POINT('Origin',(31.6,39.642135623731,39.6421356)) ;
#16760=CARTESIAN_POINT('Origin',(31.6,39.642135623731,39.6421356)) ;
#16761=CARTESIAN_POINT('Origin',(31.6,39.642135623731,39.6421356)) ;
#16762=CARTESIAN_POINT('',(31.6,40.5081610275154,41.142135623731)) ;
#16763=CARTESIAN_POINT('Origin',(31.6,39.642135623731,39.6421356)) ;
#16764=CARTESIAN_POINT('Origin',(31.0796394397885,39.642135623731,39.6421356)) ;
#16765=CARTESIAN_POINT('',(30.559278879577,39.642135623731,39.6421356)) ;
#16766=CARTESIAN_POINT('',(31.0796394397885,38.7761102199465,39.6421356)) ;
#16767=CARTESIAN_POINT('Origin',(33.6,40.5081610275154,41.142135623731)) ;
#16768=CARTESIAN_POINT('',(33.6,40.5081610275154,41.142135623731)) ;
#16769=CARTESIAN_POINT('',(33.6,41.3741864312998,39.642135623731)) ;
#16770=CARTESIAN_POINT('Origin',(33.6,38.7761102199465,41.142135623731)) ;
#16771=CARTESIAN_POINT('Origin',(33.6,41.3741864312998,39.642135623731)) ;
#16930=UNCERTAINTY_MEASURE_WITH_UNIT(LENGTH_MEASURE(0.01),#16943,
'DISTANCE_ACCURACY_VALUE',
'Maximum model space distance between geometric entities at asserted c
onnectivities') ;
#16933=UNCERTAINTY_MEASURE_WITH_UNIT(LENGTH_MEASURE(0.01),#16943,
'DISTANCE_ACCURACY_VALUE',
'Maximum model space distance between geometric entities at asserted c
onnectivities') ;
#16939=(
GEOMETRIC_REPRESENTATION_CONTEXT(3)
GLOBAL_UNCERTAINTY_ASSIGNED_CONTEXT((#16930))
GLOBAL_UNIT_ASSIGNED_CONTEXT((#16943,#16945,#16946))
REPRESENTATION_CONTEXT('','3D')
) ;
#16942=(
GEOMETRIC_REPRESENTATION_CONTEXT(3)
GLOBAL_UNCERTAINTY_ASSIGNED_CONTEXT((#16933))
GLOBAL_UNIT_ASSIGNED_CONTEXT((#16943,#16945,#16946))
REPRESENTATION_CONTEXT('','3D')
) ;
#16943=(
LENGTH_UNIT()
NAMED_UNIT(*)
SI_UNIT(.MILLI.,.METRE.)
) ;
#16945=(
NAMED_UNIT(*)
PLANE_ANGLE_UNIT()
SI_UNIT($,.RADIAN.)
) ;
#16946=(
NAMED_UNIT(*)
SI_UNIT($,.STERADIAN.)
SOLID_ANGLE_UNIT()
) ;
#16952=SHAPE_DEFINITION_REPRESENTATION(#16960,#17023) ;
#16960=PRODUCT_DEFINITION_SHAPE('',$,#17032) ;
#17023=SHAPE_REPRESENTATION('',(#8596),#16939) ;
#17026=PRODUCT_DEFINITION_CONTEXT('part definition',#17052,'design') ;
#17032=PRODUCT_DEFINITION('ISO 4762 - M4 x 10 - 12.9',
'ISO 4762 - M4 x 10 - 12.9',#17040,#17026) ;
#17040=PRODUCT_DEFINITION_FORMATION('',$,#17059) ;
#17052=APPLICATION_CONTEXT(
'Core Data for Automotive Mechanical Design Process') ;
#17053=PRODUCT_CONTEXT('part definition',#17052,'mechanical') ;
#17059=PRODUCT('ISO 4762 - M4 x 10 - 12.9','ISO 4762 - M4 x 10 - 12.9',$,
(#17053)) ;
#17067=PRESENTATION_STYLE_ASSIGNMENT((#17075)) ;
#17075=SURFACE_STYLE_USAGE(.BOTH.,#17083) ;
#17083=SURFACE_SIDE_STYLE('',(#17091)) ;
#17091=SURFACE_STYLE_FILL_AREA(#17099) ;
#17099=FILL_AREA_STYLE(
'MAS-257 Metallic Sheet - ISO 4762 - M4 x 10 - 12.9',(#17107)) ;
#17107=FILL_AREA_STYLE_COLOUR(
'MAS-257 Metallic Sheet - ISO 4762 - M4 x 10 - 12.9',#17115) ;
#17115=COLOUR_RGB('MAS-257 Metallic Sheet - ISO 4762 - M4 x 10 - 12.9', 0.08235294, 0.09019608, 0.10196078) ;
ENDSEC;
END-ISO-10303-21;
